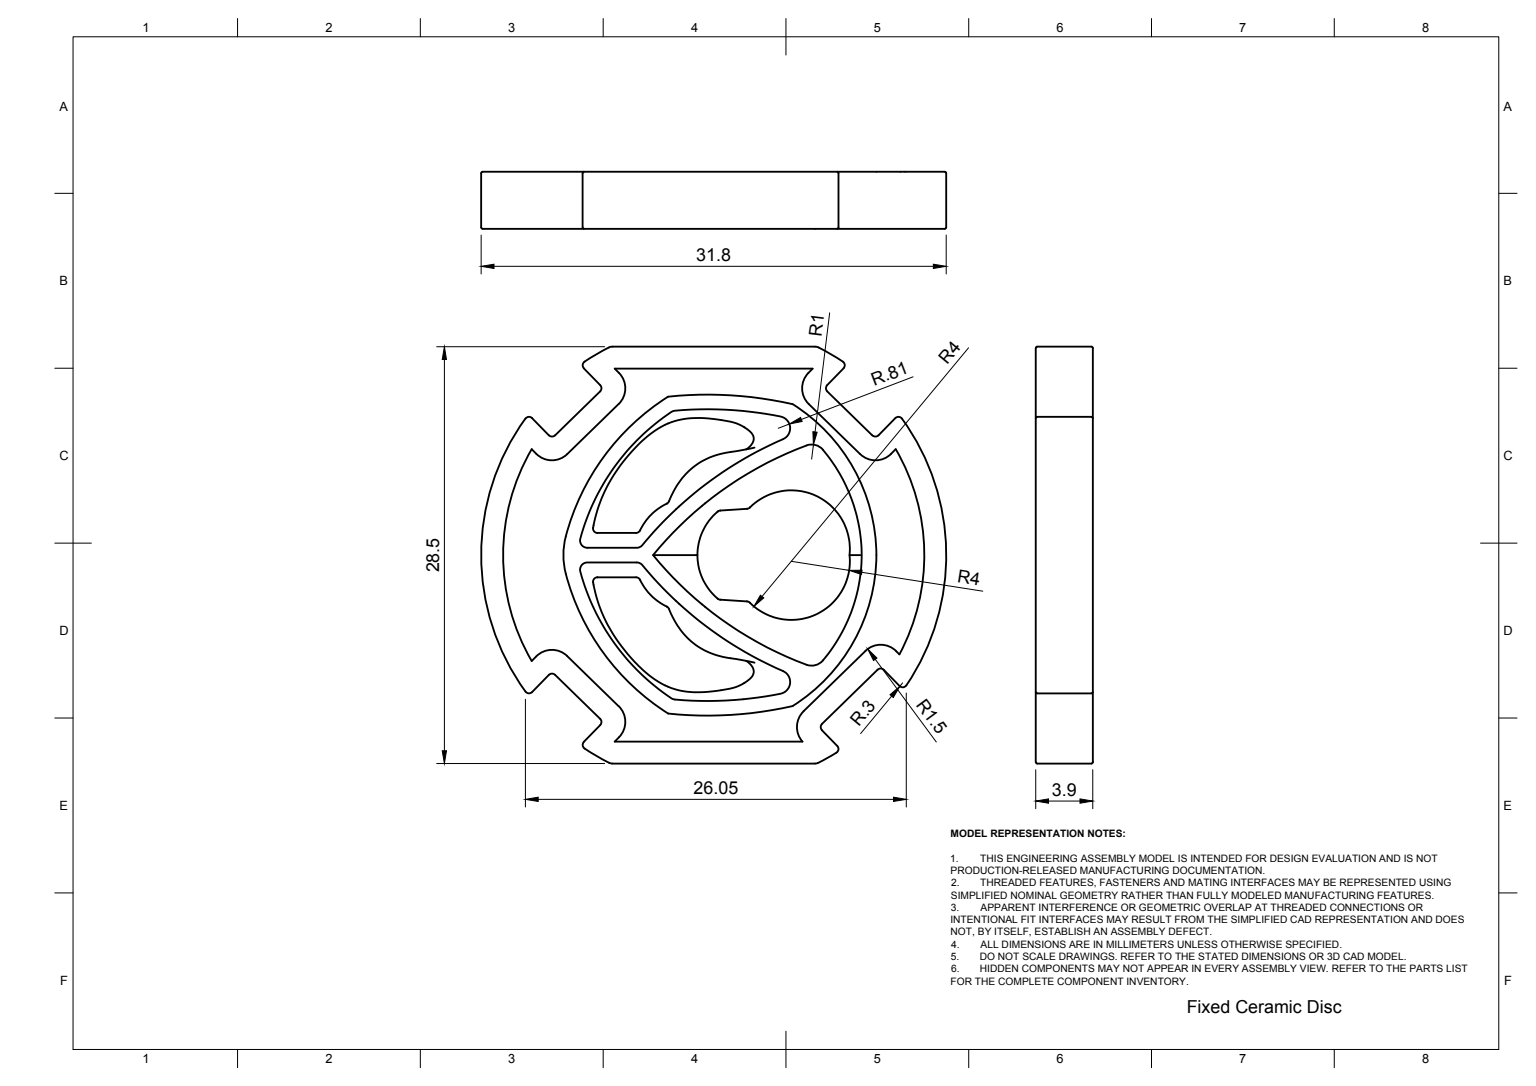
ISO-10303-21;
HEADER;
/* Generated by software containing ST-Developer
 * from STEP Tools, Inc. (www.steptools.com) 
 */

FILE_DESCRIPTION(
/* description */ ('STEP AP214'),
/* implementation_level */ '2;1');

FILE_NAME(
/* name */ 'Fixed Ceramic Disc.step',
/* time_stamp */ '2026-10-06T00:19:40-07:00',
/* author */ (''),
/* organization */ (''),
/* preprocessor_version */ 'ST-DEVELOPER v20.2',
/* originating_system */ 'Autodesk Translation Framework v15.15.0.0',
/* authorisation */ '');

FILE_SCHEMA (('AUTOMOTIVE_DESIGN { 1 0 10303 214 3 1 1 }'));
ENDSEC;

DATA;
#10=MECHANICAL_DESIGN_GEOMETRIC_PRESENTATION_REPRESENTATION('',(#2064),#98302);
#66=TOROIDAL_SURFACE('',#34375,15.8,0.1);
#67=TOROIDAL_SURFACE('',#34378,0.2,0.1);
#68=TOROIDAL_SURFACE('',#34386,0.4,0.1);
#69=TOROIDAL_SURFACE('',#34394,0.4,0.1);
#70=TOROIDAL_SURFACE('',#34402,0.2,0.1);
#71=TOROIDAL_SURFACE('',#34407,15.8,0.1);
#72=TOROIDAL_SURFACE('',#34412,0.4,0.1);
#73=TOROIDAL_SURFACE('',#34420,0.4,0.1);
#74=TOROIDAL_SURFACE('',#34425,15.8,0.1);
#75=TOROIDAL_SURFACE('',#34430,0.2,0.1);
#76=TOROIDAL_SURFACE('',#34438,0.4,0.1);
#77=TOROIDAL_SURFACE('',#34446,0.4,0.1);
#78=TOROIDAL_SURFACE('',#34454,0.2,0.1);
#79=TOROIDAL_SURFACE('',#34462,15.8,0.1);
#80=TOROIDAL_SURFACE('',#34464,0.2,0.1);
#81=TOROIDAL_SURFACE('',#34472,0.4,0.1);
#82=TOROIDAL_SURFACE('',#34480,0.4,0.1);
#83=TOROIDAL_SURFACE('',#34488,0.2,0.1);
#84=TOROIDAL_SURFACE('',#34493,15.8,0.1);
#85=TOROIDAL_SURFACE('',#34498,0.4,0.1);
#86=TOROIDAL_SURFACE('',#34506,0.4,0.1);
#87=TOROIDAL_SURFACE('',#34511,15.8,0.1);
#88=TOROIDAL_SURFACE('',#34516,0.2,0.1);
#89=TOROIDAL_SURFACE('',#34524,0.4,0.1);
#90=TOROIDAL_SURFACE('',#34532,0.2,0.1);
#91=TOROIDAL_SURFACE('',#34537,0.4,0.1);
#92=TOROIDAL_SURFACE('',#34602,15.8,0.1);
#93=TOROIDAL_SURFACE('',#34606,0.2,0.1);
#94=TOROIDAL_SURFACE('',#34611,0.4,0.1);
#95=TOROIDAL_SURFACE('',#34616,0.4,0.1);
#96=TOROIDAL_SURFACE('',#34621,0.2,0.1);
#97=TOROIDAL_SURFACE('',#34624,15.8,0.1);
#98=TOROIDAL_SURFACE('',#34627,0.4,0.1);
#99=TOROIDAL_SURFACE('',#34632,0.4,0.1);
#100=TOROIDAL_SURFACE('',#34635,15.8,0.1);
#101=TOROIDAL_SURFACE('',#34638,0.2,0.1);
#102=TOROIDAL_SURFACE('',#34643,0.4,0.1);
#103=TOROIDAL_SURFACE('',#34648,0.4,0.1);
#104=TOROIDAL_SURFACE('',#34653,0.2,0.1);
#105=TOROIDAL_SURFACE('',#34656,15.8,0.1);
#106=TOROIDAL_SURFACE('',#34659,0.2,0.1);
#107=TOROIDAL_SURFACE('',#34664,0.4,0.1);
#108=TOROIDAL_SURFACE('',#34669,0.4,0.1);
#109=TOROIDAL_SURFACE('',#34674,0.2,0.1);
#110=TOROIDAL_SURFACE('',#34677,15.8,0.1);
#111=TOROIDAL_SURFACE('',#34680,0.4,0.1);
#112=TOROIDAL_SURFACE('',#34685,0.4,0.1);
#113=TOROIDAL_SURFACE('',#34688,15.8,0.1);
#114=TOROIDAL_SURFACE('',#34691,0.2,0.1);
#115=TOROIDAL_SURFACE('',#34696,0.4,0.1);
#116=TOROIDAL_SURFACE('',#34701,0.2,0.1);
#117=TOROIDAL_SURFACE('',#34704,0.4,0.1);
#449=ELLIPSE('',#34351,0.0975089533003066,0.0318233698452749);
#450=ELLIPSE('',#34354,0.210203962458616,0.0684164528781414);
#451=ELLIPSE('',#34355,4.51181641557726,0.330426027279306);
#452=ELLIPSE('',#34356,0.371777616681055,0.0636641381433054);
#453=ELLIPSE('',#34358,1.12077531771054,0.208207940858736);
#454=ELLIPSE('',#34360,7.044836022966,0.27423437971207);
#455=ELLIPSE('',#34362,0.0975089533003066,0.0318233698452749);
#456=ELLIPSE('',#34364,7.044836022966,0.27423437971207);
#457=ELLIPSE('',#34365,1.12077531771054,0.208207940858736);
#458=ELLIPSE('',#34367,0.371777616681055,0.0636641381433054);
#459=ELLIPSE('',#34369,4.51181641557726,0.330426027279306);
#460=ELLIPSE('',#34370,0.210203962458616,0.0684164528781414);
#461=ELLIPSE('',#34546,4.64326105948723,1.41336611178093);
#462=ELLIPSE('',#34562,4.51762701288,1.39428357264109);
#463=ELLIPSE('',#34573,0.257803751558044,0.175002130709107);
#464=ELLIPSE('',#34575,0.1975438935833,0.117585941695249);
#465=ELLIPSE('',#34583,0.249924507512202,0.163903784221422);
#466=ELLIPSE('',#34586,0.1975438935833,0.117585941695249);
#467=ELLIPSE('',#34754,0.0363695267596646,0.0157585247759226);
#468=ELLIPSE('',#34757,0.0363695267596646,0.0157585247759226);
#469=ELLIPSE('',#34761,0.0439364458692703,0.0199986358668788);
#470=ELLIPSE('',#34763,0.751422058778054,0.147149952825287);
#471=ELLIPSE('',#34765,20.1759483174618,1.96800786553162);
#472=ELLIPSE('',#34766,20.1759483174618,1.96800786553162);
#473=ELLIPSE('',#34768,0.751422058778054,0.147149952825287);
#474=ELLIPSE('',#34770,0.0439364458692703,0.0199986358668788);
#475=ELLIPSE('',#34772,0.299969315421473,0.299941755102118);
#476=ELLIPSE('',#34773,0.299972264763754,0.299945275725425);
#477=ELLIPSE('',#34774,0.0990009013291418,0.0878823615802462);
#478=ELLIPSE('',#34780,0.299972288094039,0.299945322652049);
#479=ELLIPSE('',#34781,0.299969314787288,0.299941753885528);
#480=ELLIPSE('',#34782,0.0990009013291418,0.0878823615802462);
#481=ELLIPSE('',#34793,0.7851617239929,0.0246669925758606);
#482=ELLIPSE('',#34796,0.7851617239929,0.0246669925758606);
#710=SPHERICAL_SURFACE('',#34346,0.3);
#711=SPHERICAL_SURFACE('',#34785,0.3);
#862=B_SPLINE_SURFACE_WITH_KNOTS('',5,1,((#49366,#49367),(#49368,#49369),
(#49370,#49371),(#49372,#49373),(#49374,#49375),(#49376,#49377),(#49378,
#49379),(#49380,#49381),(#49382,#49383)),.UNSPECIFIED.,.F.,.F.,.F.,(6,3,
6),(2,2),(0.,2.10936312981,4.22279623369),(0.,3.10437234689),
 .UNSPECIFIED.);
#863=B_SPLINE_SURFACE_WITH_KNOTS('',5,1,((#49466,#49467),(#49468,#49469),
(#49470,#49471),(#49472,#49473),(#49474,#49475),(#49476,#49477),(#49478,
#49479),(#49480,#49481),(#49482,#49483)),.UNSPECIFIED.,.F.,.F.,.F.,(6,3,
6),(2,2),(0.11111371251,1.22636799075,2.75103476973),(0.,0.108300515181936),
 .UNSPECIFIED.);
#864=B_SPLINE_SURFACE_WITH_KNOTS('',5,1,((#49587,#49588),(#49589,#49590),
(#49591,#49592),(#49593,#49594),(#49595,#49596),(#49597,#49598),(#49599,
#49600),(#49601,#49602),(#49603,#49604),(#49605,#49606),(#49607,#49608),
(#49609,#49610),(#49611,#49612),(#49613,#49614),(#49615,#49616),(#49617,
#49618),(#49619,#49620),(#49621,#49622)),.UNSPECIFIED.,.F.,.F.,.F.,(6,3,
3,3,3,6),(2,2),(0.465128126763,3.42050470566,7.30063973795,10.0042092191,
12.4987596036,13.1731669678),(0.,0.115270049227219),.UNSPECIFIED.);
#865=B_SPLINE_SURFACE_WITH_KNOTS('',5,1,((#49746,#49747),(#49748,#49749),
(#49750,#49751),(#49752,#49753),(#49754,#49755),(#49756,#49757)),
 .UNSPECIFIED.,.F.,.F.,.F.,(6,6),(2,2),(0.,1.62525620495),(0.,0.103685293259447),
 .UNSPECIFIED.);
#866=B_SPLINE_SURFACE_WITH_KNOTS('',5,1,((#49791,#49792),(#49793,#49794),
(#49795,#49796),(#49797,#49798),(#49799,#49800),(#49801,#49802),(#49803,
#49804),(#49805,#49806),(#49807,#49808),(#49809,#49810),(#49811,#49812),
(#49813,#49814),(#49815,#49816),(#49817,#49818),(#49819,#49820)),
 .UNSPECIFIED.,.F.,.F.,.F.,(6,3,3,3,6),(2,2),(0.617889185003,0.915206541473,
1.58780472511,2.42003303229,2.57855093571),(0.,0.109749059692414),
 .UNSPECIFIED.);
#867=B_SPLINE_SURFACE_WITH_KNOTS('',5,1,((#49873,#49874),(#49875,#49876),
(#49877,#49878),(#49879,#49880),(#49881,#49882),(#49883,#49884)),
 .UNSPECIFIED.,.F.,.F.,.F.,(6,6),(2,2),(0.,0.788840280269),(0.,0.12),
 .UNSPECIFIED.);
#868=B_SPLINE_SURFACE_WITH_KNOTS('',5,1,((#49932,#49933),(#49934,#49935),
(#49936,#49937),(#49938,#49939),(#49940,#49941),(#49942,#49943),(#49944,
#49945),(#49946,#49947),(#49948,#49949)),.UNSPECIFIED.,.F.,.F.,.F.,(6,3,
6),(2,2),(0.248824060028,2.99459552346,6.14853595161),(0.,0.120001139724),
 .UNSPECIFIED.);
#869=B_SPLINE_SURFACE_WITH_KNOTS('',5,1,((#50067,#50068),(#50069,#50070),
(#50071,#50072),(#50073,#50074),(#50075,#50076),(#50077,#50078),(#50079,
#50080),(#50081,#50082),(#50083,#50084)),.UNSPECIFIED.,.F.,.F.,.F.,(6,3,
6),(2,2),(0.11111371251,1.22636799075,2.75103476973),(0.,0.108300515181936),
 .UNSPECIFIED.);
#870=B_SPLINE_SURFACE_WITH_KNOTS('',5,1,((#50165,#50166),(#50167,#50168),
(#50169,#50170),(#50171,#50172),(#50173,#50174),(#50175,#50176),(#50177,
#50178),(#50179,#50180),(#50181,#50182)),.UNSPECIFIED.,.F.,.F.,.F.,(6,3,
6),(2,2),(0.248824060028,2.99459552346,6.14853595161),(0.,0.120001139724),
 .UNSPECIFIED.);
#871=B_SPLINE_SURFACE_WITH_KNOTS('',5,1,((#50281,#50282),(#50283,#50284),
(#50285,#50286),(#50287,#50288),(#50289,#50290),(#50291,#50292)),
 .UNSPECIFIED.,.F.,.F.,.F.,(6,6),(2,2),(0.,0.788840280269),(0.,0.12),
 .UNSPECIFIED.);
#872=B_SPLINE_SURFACE_WITH_KNOTS('',5,1,((#50340,#50341),(#50342,#50343),
(#50344,#50345),(#50346,#50347),(#50348,#50349),(#50350,#50351),(#50352,
#50353),(#50354,#50355),(#50356,#50357),(#50358,#50359),(#50360,#50361),
(#50362,#50363),(#50364,#50365),(#50366,#50367),(#50368,#50369)),
 .UNSPECIFIED.,.F.,.F.,.F.,(6,3,3,3,6),(2,2),(0.617889185003,0.915206541473,
1.58780472511,2.42003303229,2.57855093571),(0.,0.109749059692414),
 .UNSPECIFIED.);
#873=B_SPLINE_SURFACE_WITH_KNOTS('',5,1,((#50555,#50556),(#50557,#50558),
(#50559,#50560),(#50561,#50562),(#50563,#50564),(#50565,#50566)),
 .UNSPECIFIED.,.F.,.F.,.F.,(6,6),(2,2),(0.,1.62525620495),(0.,0.103685293259447),
 .UNSPECIFIED.);
#874=B_SPLINE_SURFACE_WITH_KNOTS('',5,1,((#50600,#50601),(#50602,#50603),
(#50604,#50605),(#50606,#50607),(#50608,#50609),(#50610,#50611),(#50612,
#50613),(#50614,#50615),(#50616,#50617),(#50618,#50619),(#50620,#50621),
(#50622,#50623),(#50624,#50625),(#50626,#50627),(#50628,#50629),(#50630,
#50631),(#50632,#50633),(#50634,#50635)),.UNSPECIFIED.,.F.,.F.,.F.,(6,3,
3,3,3,6),(2,2),(0.465128126763,3.42050470566,7.30063973795,10.0042092191,
12.4987596036,13.1731669678),(0.,0.115270054056779),.UNSPECIFIED.);
#875=B_SPLINE_SURFACE_WITH_KNOTS('',5,1,((#51251,#51252),(#51253,#51254),
(#51255,#51256),(#51257,#51258),(#51259,#51260),(#51261,#51262)),
 .UNSPECIFIED.,.F.,.F.,.F.,(6,6),(2,2),(0.,0.600083611309),(0.,3.10437234689),
 .UNSPECIFIED.);
#876=B_SPLINE_SURFACE_WITH_KNOTS('',5,1,((#51336,#51337),(#51338,#51339),
(#51340,#51341),(#51342,#51343),(#51344,#51345),(#51346,#51347)),
 .UNSPECIFIED.,.F.,.F.,.F.,(6,6),(2,2),(0.,0.226010362356),(0.,3.10437234689),
 .UNSPECIFIED.);
#877=B_SPLINE_SURFACE_WITH_KNOTS('',5,1,((#51368,#51369),(#51370,#51371),
(#51372,#51373),(#51374,#51375),(#51376,#51377),(#51378,#51379),(#51380,
#51381),(#51382,#51383),(#51384,#51385),(#51386,#51387),(#51388,#51389),
(#51390,#51391)),.UNSPECIFIED.,.F.,.F.,.F.,(6,3,3,6),(2,2),(0.,2.83532528452,
6.09533201542,9.83397913335),(0.,3.10437234689),.UNSPECIFIED.);
#878=B_SPLINE_SURFACE_WITH_KNOTS('',5,1,((#51471,#51472),(#51473,#51474),
(#51475,#51476),(#51477,#51478),(#51479,#51480),(#51481,#51482)),
 .UNSPECIFIED.,.F.,.F.,.F.,(6,6),(2,2),(0.,0.224378834114),(0.,3.10437234689),
 .UNSPECIFIED.);
#879=B_SPLINE_SURFACE_WITH_KNOTS('',5,1,((#51514,#51515),(#51516,#51517),
(#51518,#51519),(#51520,#51521),(#51522,#51523),(#51524,#51525)),
 .UNSPECIFIED.,.F.,.F.,.F.,(6,6),(2,2),(0.,0.2489231439),(0.,3.10437234689),
 .UNSPECIFIED.);
#880=B_SPLINE_SURFACE_WITH_KNOTS('',5,1,((#51570,#51571),(#51572,#51573),
(#51574,#51575),(#51576,#51577),(#51578,#51579),(#51580,#51581),(#51582,
#51583),(#51584,#51585),(#51586,#51587),(#51588,#51589),(#51590,#51591),
(#51592,#51593)),.UNSPECIFIED.,.F.,.F.,.F.,(6,3,3,6),(2,2),(0.,0.629547398659,
1.2493532974,1.86132516749),(0.,3.10437234689),.UNSPECIFIED.);
#881=B_SPLINE_SURFACE_WITH_KNOTS('',5,1,((#51679,#51680),(#51681,#51682),
(#51683,#51684),(#51685,#51686),(#51687,#51688),(#51689,#51690)),
 .UNSPECIFIED.,.F.,.F.,.F.,(6,6),(2,2),(0.,0.482067685837),(0.,3.10437234689),
 .UNSPECIFIED.);
#882=B_SPLINE_SURFACE_WITH_KNOTS('',5,1,((#51717,#51718),(#51719,#51720),
(#51721,#51722),(#51723,#51724),(#51725,#51726),(#51727,#51728)),
 .UNSPECIFIED.,.F.,.F.,.F.,(6,6),(2,2),(0.,1.84813202664),(0.,3.10437234689),
 .UNSPECIFIED.);
#883=B_SPLINE_SURFACE_WITH_KNOTS('',5,5,((#51829,#51830,#51831,#51832,#51833,
#51834),(#51835,#51836,#51837,#51838,#51839,#51840),(#51841,#51842,#51843,
#51844,#51845,#51846),(#51847,#51848,#51849,#51850,#51851,#51852),(#51853,
#51854,#51855,#51856,#51857,#51858),(#51859,#51860,#51861,#51862,#51863,
#51864)),.UNSPECIFIED.,.F.,.F.,.F.,(6,6),(6,6),(0.840058180513,4.79280767082),
(0.,1.),.UNSPECIFIED.);
#884=B_SPLINE_SURFACE_WITH_KNOTS('',5,5,((#51900,#51901,#51902,#51903,#51904,
#51905),(#51906,#51907,#51908,#51909,#51910,#51911),(#51912,#51913,#51914,
#51915,#51916,#51917),(#51918,#51919,#51920,#51921,#51922,#51923),(#51924,
#51925,#51926,#51927,#51928,#51929),(#51930,#51931,#51932,#51933,#51934,
#51935),(#51936,#51937,#51938,#51939,#51940,#51941),(#51942,#51943,#51944,
#51945,#51946,#51947),(#51948,#51949,#51950,#51951,#51952,#51953)),
 .UNSPECIFIED.,.F.,.F.,.F.,(6,3,6),(6,6),(0.225815728085,0.523709124902,
0.747252061964),(0.,1.),.UNSPECIFIED.);
#885=B_SPLINE_SURFACE_WITH_KNOTS('',5,5,((#51995,#51996,#51997,#51998,#51999,
#52000),(#52001,#52002,#52003,#52004,#52005,#52006),(#52007,#52008,#52009,
#52010,#52011,#52012),(#52013,#52014,#52015,#52016,#52017,#52018),(#52019,
#52020,#52021,#52022,#52023,#52024),(#52025,#52026,#52027,#52028,#52029,
#52030)),.UNSPECIFIED.,.F.,.F.,.F.,(6,6),(6,6),(1.28339894164,1.34350433703),
(0.,1.),.UNSPECIFIED.);
#886=B_SPLINE_SURFACE_WITH_KNOTS('',5,5,((#52045,#52046,#52047,#52048,#52049,
#52050),(#52051,#52052,#52053,#52054,#52055,#52056),(#52057,#52058,#52059,
#52060,#52061,#52062),(#52063,#52064,#52065,#52066,#52067,#52068),(#52069,
#52070,#52071,#52072,#52073,#52074),(#52075,#52076,#52077,#52078,#52079,
#52080)),.UNSPECIFIED.,.F.,.F.,.F.,(6,6),(6,6),(1.036743613,1.10280574369),
(0.,1.),.UNSPECIFIED.);
#887=B_SPLINE_SURFACE_WITH_KNOTS('',5,5,((#52086,#52087,#52088,#52089,#52090,
#52091),(#52092,#52093,#52094,#52095,#52096,#52097),(#52098,#52099,#52100,
#52101,#52102,#52103),(#52104,#52105,#52106,#52107,#52108,#52109),(#52110,
#52111,#52112,#52113,#52114,#52115),(#52116,#52117,#52118,#52119,#52120,
#52121),(#52122,#52123,#52124,#52125,#52126,#52127),(#52128,#52129,#52130,
#52131,#52132,#52133),(#52134,#52135,#52136,#52137,#52138,#52139)),
 .UNSPECIFIED.,.F.,.F.,.F.,(6,3,6),(6,6),(0.342430056326,0.787545489389,
1.14838178471),(0.,1.),.UNSPECIFIED.);
#888=B_SPLINE_SURFACE_WITH_KNOTS('',5,5,((#52179,#52180,#52181,#52182,#52183,
#52184),(#52185,#52186,#52187,#52188,#52189,#52190),(#52191,#52192,#52193,
#52194,#52195,#52196),(#52197,#52198,#52199,#52200,#52201,#52202),(#52203,
#52204,#52205,#52206,#52207,#52208),(#52209,#52210,#52211,#52212,#52213,
#52214)),.UNSPECIFIED.,.F.,.F.,.F.,(6,6),(6,6),(1.40817420416,1.45205022904),
(0.,1.),.UNSPECIFIED.);
#889=B_SPLINE_SURFACE_WITH_KNOTS('',5,5,((#52216,#52217,#52218,#52219,#52220,
#52221),(#52222,#52223,#52224,#52225,#52226,#52227),(#52228,#52229,#52230,
#52231,#52232,#52233),(#52234,#52235,#52236,#52237,#52238,#52239),(#52240,
#52241,#52242,#52243,#52244,#52245),(#52246,#52247,#52248,#52249,#52250,
#52251),(#52252,#52253,#52254,#52255,#52256,#52257),(#52258,#52259,#52260,
#52261,#52262,#52263),(#52264,#52265,#52266,#52267,#52268,#52269),(#52270,
#52271,#52272,#52273,#52274,#52275),(#52276,#52277,#52278,#52279,#52280,
#52281),(#52282,#52283,#52284,#52285,#52286,#52287)),.UNSPECIFIED.,.F.,
 .F.,.F.,(6,3,3,6),(6,6),(4.46364567829,9.98301756848,13.6615164274,17.5757040899),
(0.,1.),.UNSPECIFIED.);
#890=B_SPLINE_SURFACE_WITH_KNOTS('',5,5,((#52425,#52426,#52427,#52428,#52429,
#52430),(#52431,#52432,#52433,#52434,#52435,#52436),(#52437,#52438,#52439,
#52440,#52441,#52442),(#52443,#52444,#52445,#52446,#52447,#52448),(#52449,
#52450,#52451,#52452,#52453,#52454),(#52455,#52456,#52457,#52458,#52459,
#52460),(#52461,#52462,#52463,#52464,#52465,#52466),(#52467,#52468,#52469,
#52470,#52471,#52472),(#52473,#52474,#52475,#52476,#52477,#52478)),
 .UNSPECIFIED.,.F.,.F.,.F.,(6,3,6),(6,6),(1.01054285509,1.23011259501,1.32384910338),
(0.,1.),.UNSPECIFIED.);
#891=B_SPLINE_SURFACE_WITH_KNOTS('',5,5,((#52506,#52507,#52508,#52509,#52510,
#52511),(#52512,#52513,#52514,#52515,#52516,#52517),(#52518,#52519,#52520,
#52521,#52522,#52523),(#52524,#52525,#52526,#52527,#52528,#52529),(#52530,
#52531,#52532,#52533,#52534,#52535),(#52536,#52537,#52538,#52539,#52540,
#52541),(#52542,#52543,#52544,#52545,#52546,#52547),(#52548,#52549,#52550,
#52551,#52552,#52553),(#52554,#52555,#52556,#52557,#52558,#52559)),
 .UNSPECIFIED.,.F.,.F.,.F.,(6,3,6),(6,6),(2.57539738198,5.72432320356,8.12037630607),
(0.,1.),.UNSPECIFIED.);
#892=B_SPLINE_SURFACE_WITH_KNOTS('',5,5,((#52650,#52651,#52652,#52653,#52654,
#52655),(#52656,#52657,#52658,#52659,#52660,#52661),(#52662,#52663,#52664,
#52665,#52666,#52667),(#52668,#52669,#52670,#52671,#52672,#52673),(#52674,
#52675,#52676,#52677,#52678,#52679),(#52680,#52681,#52682,#52683,#52684,
#52685)),.UNSPECIFIED.,.F.,.F.,.F.,(6,6),(6,6),(0.993700418328028,1.22287270565897),
(-0.00157928356897239,1.00011077696173),.UNSPECIFIED.);
#893=B_SPLINE_SURFACE_WITH_KNOTS('',5,5,((#52690,#52691,#52692,#52693,#52694,
#52695),(#52696,#52697,#52698,#52699,#52700,#52701),(#52702,#52703,#52704,
#52705,#52706,#52707),(#52708,#52709,#52710,#52711,#52712,#52713),(#52714,
#52715,#52716,#52717,#52718,#52719),(#52720,#52721,#52722,#52723,#52724,
#52725)),.UNSPECIFIED.,.F.,.F.,.F.,(6,6),(6,6),(2.37851323355,2.46410111513),
(0.,1.),.UNSPECIFIED.);
#894=B_SPLINE_SURFACE_WITH_KNOTS('',5,5,((#52738,#52739,#52740,#52741,#52742,
#52743),(#52744,#52745,#52746,#52747,#52748,#52749),(#52750,#52751,#52752,
#52753,#52754,#52755),(#52756,#52757,#52758,#52759,#52760,#52761),(#52762,
#52763,#52764,#52765,#52766,#52767),(#52768,#52769,#52770,#52771,#52772,
#52773),(#52774,#52775,#52776,#52777,#52778,#52779),(#52780,#52781,#52782,
#52783,#52784,#52785),(#52786,#52787,#52788,#52789,#52790,#52791)),
 .UNSPECIFIED.,.F.,.F.,.F.,(6,3,6),(6,6),(0.586327318555,1.59285457075,
2.96825275179),(0.,1.),.UNSPECIFIED.);
#895=B_SPLINE_SURFACE_WITH_KNOTS('',5,5,((#52906,#52907,#52908,#52909,#52910,
#52911),(#52912,#52913,#52914,#52915,#52916,#52917),(#52918,#52919,#52920,
#52921,#52922,#52923),(#52924,#52925,#52926,#52927,#52928,#52929),(#52930,
#52931,#52932,#52933,#52934,#52935),(#52936,#52937,#52938,#52939,#52940,
#52941)),.UNSPECIFIED.,.F.,.F.,.F.,(6,6),(6,6),(0.881014033286,0.963434555076),
(0.,1.),.UNSPECIFIED.);
#896=B_SPLINE_SURFACE_WITH_KNOTS('',5,5,((#52951,#52952,#52953,#52954,#52955,
#52956),(#52957,#52958,#52959,#52960,#52961,#52962),(#52963,#52964,#52965,
#52966,#52967,#52968),(#52969,#52970,#52971,#52972,#52973,#52974),(#52975,
#52976,#52977,#52978,#52979,#52980),(#52981,#52982,#52983,#52984,#52985,
#52986),(#52987,#52988,#52989,#52990,#52991,#52992),(#52993,#52994,#52995,
#52996,#52997,#52998),(#52999,#53000,#53001,#53002,#53003,#53004)),
 .UNSPECIFIED.,.F.,.F.,.F.,(6,3,6),(6,6),(0.734432475987,1.16119681048,
1.33983380059),(0.,1.),.UNSPECIFIED.);
#897=B_SPLINE_SURFACE_WITH_KNOTS('',5,5,((#53026,#53027,#53028,#53029,#53030,
#53031),(#53032,#53033,#53034,#53035,#53036,#53037),(#53038,#53039,#53040,
#53041,#53042,#53043),(#53044,#53045,#53046,#53047,#53048,#53049),(#53050,
#53051,#53052,#53053,#53054,#53055),(#53056,#53057,#53058,#53059,#53060,
#53061),(#53062,#53063,#53064,#53065,#53066,#53067),(#53068,#53069,#53070,
#53071,#53072,#53073),(#53074,#53075,#53076,#53077,#53078,#53079),(#53080,
#53081,#53082,#53083,#53084,#53085),(#53086,#53087,#53088,#53089,#53090,
#53091),(#53092,#53093,#53094,#53095,#53096,#53097)),.UNSPECIFIED.,.F.,
 .F.,.F.,(6,3,3,6),(6,6),(1.14300114544,1.64244110169,2.30706085766,3.58561463726),
(0.,1.),.UNSPECIFIED.);
#898=B_SPLINE_SURFACE_WITH_KNOTS('',5,5,((#53200,#53201,#53202,#53203,#53204,
#53205),(#53206,#53207,#53208,#53209,#53210,#53211),(#53212,#53213,#53214,
#53215,#53216,#53217),(#53218,#53219,#53220,#53221,#53222,#53223),(#53224,
#53225,#53226,#53227,#53228,#53229),(#53230,#53231,#53232,#53233,#53234,
#53235)),.UNSPECIFIED.,.F.,.F.,.F.,(6,6),(6,6),(1.26425849888,1.32115953697),
(0.,1.),.UNSPECIFIED.);
#899=B_SPLINE_SURFACE_WITH_KNOTS('',5,1,((#53242,#53243),(#53244,#53245),
(#53246,#53247),(#53248,#53249),(#53250,#53251),(#53252,#53253)),
 .UNSPECIFIED.,.F.,.F.,.F.,(6,6),(2,2),(0.,0.898161272296),(0.,3.10437234689),
 .UNSPECIFIED.);
#900=B_SPLINE_SURFACE_WITH_KNOTS('',3,5,((#53286,#53287,#53288,#53289,#53290,
#53291),(#53292,#53293,#53294,#53295,#53296,#53297),(#53298,#53299,#53300,
#53301,#53302,#53303),(#53304,#53305,#53306,#53307,#53308,#53309)),
 .UNSPECIFIED.,.F.,.F.,.F.,(4,4),(6,6),(0.338318706236,0.636935495757),
(0.,1.),.UNSPECIFIED.);
#901=B_SPLINE_SURFACE_WITH_KNOTS('',5,1,((#53310,#53311),(#53312,#53313),
(#53314,#53315),(#53316,#53317),(#53318,#53319),(#53320,#53321),(#53322,
#53323),(#53324,#53325),(#53326,#53327)),.UNSPECIFIED.,.F.,.F.,.F.,(6,3,
6),(2,2),(0.,3.38335932988,6.7689179912),(-4.93438140460603E-6,3.10437234689),
 .UNSPECIFIED.);
#902=B_SPLINE_SURFACE_WITH_KNOTS('',5,5,((#53466,#53467,#53468,#53469,#53470,
#53471),(#53472,#53473,#53474,#53475,#53476,#53477),(#53478,#53479,#53480,
#53481,#53482,#53483),(#53484,#53485,#53486,#53487,#53488,#53489),(#53490,
#53491,#53492,#53493,#53494,#53495),(#53496,#53497,#53498,#53499,#53500,
#53501),(#53502,#53503,#53504,#53505,#53506,#53507),(#53508,#53509,#53510,
#53511,#53512,#53513),(#53514,#53515,#53516,#53517,#53518,#53519),(#53520,
#53521,#53522,#53523,#53524,#53525),(#53526,#53527,#53528,#53529,#53530,
#53531),(#53532,#53533,#53534,#53535,#53536,#53537)),.UNSPECIFIED.,.F.,
 .F.,.F.,(6,3,3,6),(6,6),(0.,2.20713855153,4.85810064575,8.61717037377),
(0.,1.),.UNSPECIFIED.);
#903=B_SPLINE_SURFACE_WITH_KNOTS('',5,5,((#53539,#53540,#53541,#53542,#53543,
#53544),(#53545,#53546,#53547,#53548,#53549,#53550),(#53551,#53552,#53553,
#53554,#53555,#53556),(#53557,#53558,#53559,#53560,#53561,#53562),(#53563,
#53564,#53565,#53566,#53567,#53568),(#53569,#53570,#53571,#53572,#53573,
#53574)),.UNSPECIFIED.,.F.,.F.,.F.,(6,6),(6,6),(2.946262962,2.98811189909),
(0.,1.),.UNSPECIFIED.);
#904=B_SPLINE_SURFACE_WITH_KNOTS('',5,5,((#53578,#53579,#53580,#53581,#53582,
#53583),(#53584,#53585,#53586,#53587,#53588,#53589),(#53590,#53591,#53592,
#53593,#53594,#53595),(#53596,#53597,#53598,#53599,#53600,#53601),(#53602,
#53603,#53604,#53605,#53606,#53607),(#53608,#53609,#53610,#53611,#53612,
#53613),(#53614,#53615,#53616,#53617,#53618,#53619),(#53620,#53621,#53622,
#53623,#53624,#53625),(#53626,#53627,#53628,#53629,#53630,#53631)),
 .UNSPECIFIED.,.F.,.F.,.F.,(6,3,6),(6,6),(0.160705691504905,0.296334742315,
0.49268070055009),(-0.00285589455108982,1.),.UNSPECIFIED.);
#905=B_SPLINE_SURFACE_WITH_KNOTS('',5,5,((#53652,#53653,#53654,#53655,#53656,
#53657),(#53658,#53659,#53660,#53661,#53662,#53663),(#53664,#53665,#53666,
#53667,#53668,#53669),(#53670,#53671,#53672,#53673,#53674,#53675),(#53676,
#53677,#53678,#53679,#53680,#53681),(#53682,#53683,#53684,#53685,#53686,
#53687)),.UNSPECIFIED.,.F.,.F.,.F.,(6,6),(6,6),(1.51692742518,1.55221398826),
(0.,1.),.UNSPECIFIED.);
#906=B_SPLINE_SURFACE_WITH_KNOTS('',5,5,((#53688,#53689,#53690,#53691,#53692,
#53693),(#53694,#53695,#53696,#53697,#53698,#53699),(#53700,#53701,#53702,
#53703,#53704,#53705),(#53706,#53707,#53708,#53709,#53710,#53711),(#53712,
#53713,#53714,#53715,#53716,#53717),(#53718,#53719,#53720,#53721,#53722,
#53723)),.UNSPECIFIED.,.F.,.F.,.F.,(6,6),(6,6),(1.28339894164,1.34350433703),
(0.,1.),.UNSPECIFIED.);
#907=B_SPLINE_SURFACE_WITH_KNOTS('',5,5,((#53738,#53739,#53740,#53741,#53742,
#53743),(#53744,#53745,#53746,#53747,#53748,#53749),(#53750,#53751,#53752,
#53753,#53754,#53755),(#53756,#53757,#53758,#53759,#53760,#53761),(#53762,
#53763,#53764,#53765,#53766,#53767),(#53768,#53769,#53770,#53771,#53772,
#53773),(#53774,#53775,#53776,#53777,#53778,#53779),(#53780,#53781,#53782,
#53783,#53784,#53785),(#53786,#53787,#53788,#53789,#53790,#53791)),
 .UNSPECIFIED.,.F.,.F.,.F.,(6,3,6),(6,6),(0.225815728085,0.523709124902,
0.747252061964),(0.,1.),.UNSPECIFIED.);
#908=B_SPLINE_SURFACE_WITH_KNOTS('',5,5,((#53802,#53803,#53804,#53805,#53806,
#53807),(#53808,#53809,#53810,#53811,#53812,#53813),(#53814,#53815,#53816,
#53817,#53818,#53819),(#53820,#53821,#53822,#53823,#53824,#53825),(#53826,
#53827,#53828,#53829,#53830,#53831),(#53832,#53833,#53834,#53835,#53836,
#53837)),.UNSPECIFIED.,.F.,.F.,.F.,(6,6),(6,6),(0.840058180513,4.79280767082),
(0.,1.),.UNSPECIFIED.);
#909=B_SPLINE_SURFACE_WITH_KNOTS('',5,5,((#53846,#53847,#53848,#53849,#53850,
#53851),(#53852,#53853,#53854,#53855,#53856,#53857),(#53858,#53859,#53860,
#53861,#53862,#53863),(#53864,#53865,#53866,#53867,#53868,#53869),(#53870,
#53871,#53872,#53873,#53874,#53875),(#53876,#53877,#53878,#53879,#53880,
#53881)),.UNSPECIFIED.,.F.,.F.,.F.,(6,6),(6,6),(1.51692742518,1.55221398826),
(0.,1.),.UNSPECIFIED.);
#910=B_SPLINE_SURFACE_WITH_KNOTS('',5,5,((#53886,#53887,#53888,#53889,#53890,
#53891),(#53892,#53893,#53894,#53895,#53896,#53897),(#53898,#53899,#53900,
#53901,#53902,#53903),(#53904,#53905,#53906,#53907,#53908,#53909),(#53910,
#53911,#53912,#53913,#53914,#53915),(#53916,#53917,#53918,#53919,#53920,
#53921),(#53922,#53923,#53924,#53925,#53926,#53927),(#53928,#53929,#53930,
#53931,#53932,#53933),(#53934,#53935,#53936,#53937,#53938,#53939)),
 .UNSPECIFIED.,.F.,.F.,.F.,(6,3,6),(6,6),(0.163561586047,0.296334742315,
0.489824805999),(0.,1.),.UNSPECIFIED.);
#911=B_SPLINE_SURFACE_WITH_KNOTS('',5,5,((#53941,#53942,#53943,#53944,#53945,
#53946),(#53947,#53948,#53949,#53950,#53951,#53952),(#53953,#53954,#53955,
#53956,#53957,#53958),(#53959,#53960,#53961,#53962,#53963,#53964),(#53965,
#53966,#53967,#53968,#53969,#53970),(#53971,#53972,#53973,#53974,#53975,
#53976)),.UNSPECIFIED.,.F.,.F.,.F.,(6,6),(6,6),(2.946262962,2.98811189909),
(0.,1.),.UNSPECIFIED.);
#912=B_SPLINE_SURFACE_WITH_KNOTS('',5,5,((#53978,#53979,#53980,#53981,#53982,
#53983),(#53984,#53985,#53986,#53987,#53988,#53989),(#53990,#53991,#53992,
#53993,#53994,#53995),(#53996,#53997,#53998,#53999,#54000,#54001),(#54002,
#54003,#54004,#54005,#54006,#54007),(#54008,#54009,#54010,#54011,#54012,
#54013),(#54014,#54015,#54016,#54017,#54018,#54019),(#54020,#54021,#54022,
#54023,#54024,#54025),(#54026,#54027,#54028,#54029,#54030,#54031),(#54032,
#54033,#54034,#54035,#54036,#54037),(#54038,#54039,#54040,#54041,#54042,
#54043),(#54044,#54045,#54046,#54047,#54048,#54049)),.UNSPECIFIED.,.F.,
 .F.,.F.,(6,3,3,6),(6,6),(0.,2.20713855153,4.85810064575,8.61717037377),
(0.,1.),.UNSPECIFIED.);
#913=B_SPLINE_SURFACE_WITH_KNOTS('',5,1,((#54062,#54063),(#54064,#54065),
(#54066,#54067),(#54068,#54069),(#54070,#54071),(#54072,#54073),(#54074,
#54075),(#54076,#54077),(#54078,#54079)),.UNSPECIFIED.,.F.,.F.,.F.,(6,3,
6),(2,2),(0.,3.38335932988,6.7689179912),(-1.30243697672538E-5,3.10437234689),
 .UNSPECIFIED.);
#914=B_SPLINE_SURFACE_WITH_KNOTS('',5,1,((#54088,#54089),(#54090,#54091),
(#54092,#54093),(#54094,#54095),(#54096,#54097),(#54098,#54099)),
 .UNSPECIFIED.,.F.,.F.,.F.,(6,6),(2,2),(0.,0.898161272296),(0.,3.10437234689),
 .UNSPECIFIED.);
#915=B_SPLINE_SURFACE_WITH_KNOTS('',3,5,((#54135,#54136,#54137,#54138,#54139,
#54140),(#54141,#54142,#54143,#54144,#54145,#54146),(#54147,#54148,#54149,
#54150,#54151,#54152),(#54153,#54154,#54155,#54156,#54157,#54158)),
 .UNSPECIFIED.,.F.,.F.,.F.,(4,4),(6,6),(0.338318706236,0.636935495757),
(0.,1.),.UNSPECIFIED.);
#916=B_SPLINE_SURFACE_WITH_KNOTS('',5,5,((#54160,#54161,#54162,#54163,#54164,
#54165),(#54166,#54167,#54168,#54169,#54170,#54171),(#54172,#54173,#54174,
#54175,#54176,#54177),(#54178,#54179,#54180,#54181,#54182,#54183),(#54184,
#54185,#54186,#54187,#54188,#54189),(#54190,#54191,#54192,#54193,#54194,
#54195)),.UNSPECIFIED.,.F.,.F.,.F.,(6,6),(6,6),(1.26425849888,1.32115953697),
(0.,1.),.UNSPECIFIED.);
#917=B_SPLINE_SURFACE_WITH_KNOTS('',5,5,((#54197,#54198,#54199,#54200,#54201,
#54202),(#54203,#54204,#54205,#54206,#54207,#54208),(#54209,#54210,#54211,
#54212,#54213,#54214),(#54215,#54216,#54217,#54218,#54219,#54220),(#54221,
#54222,#54223,#54224,#54225,#54226),(#54227,#54228,#54229,#54230,#54231,
#54232),(#54233,#54234,#54235,#54236,#54237,#54238),(#54239,#54240,#54241,
#54242,#54243,#54244),(#54245,#54246,#54247,#54248,#54249,#54250),(#54251,
#54252,#54253,#54254,#54255,#54256),(#54257,#54258,#54259,#54260,#54261,
#54262),(#54263,#54264,#54265,#54266,#54267,#54268)),.UNSPECIFIED.,.F.,
 .F.,.F.,(6,3,3,6),(6,6),(1.14300114544,1.64244110169,2.30706085766,3.58561463726),
(0.,1.),.UNSPECIFIED.);
#918=B_SPLINE_SURFACE_WITH_KNOTS('',5,5,((#54270,#54271,#54272,#54273,#54274,
#54275),(#54276,#54277,#54278,#54279,#54280,#54281),(#54282,#54283,#54284,
#54285,#54286,#54287),(#54288,#54289,#54290,#54291,#54292,#54293),(#54294,
#54295,#54296,#54297,#54298,#54299),(#54300,#54301,#54302,#54303,#54304,
#54305),(#54306,#54307,#54308,#54309,#54310,#54311),(#54312,#54313,#54314,
#54315,#54316,#54317),(#54318,#54319,#54320,#54321,#54322,#54323)),
 .UNSPECIFIED.,.F.,.F.,.F.,(6,3,6),(6,6),(0.734432475987,1.16119681048,
1.33983380059),(0.,1.),.UNSPECIFIED.);
#919=B_SPLINE_SURFACE_WITH_KNOTS('',5,5,((#54325,#54326,#54327,#54328,#54329,
#54330),(#54331,#54332,#54333,#54334,#54335,#54336),(#54337,#54338,#54339,
#54340,#54341,#54342),(#54343,#54344,#54345,#54346,#54347,#54348),(#54349,
#54350,#54351,#54352,#54353,#54354),(#54355,#54356,#54357,#54358,#54359,
#54360)),.UNSPECIFIED.,.F.,.F.,.F.,(6,6),(6,6),(0.881014033286,0.963434555076),
(0.,1.),.UNSPECIFIED.);
#920=B_SPLINE_SURFACE_WITH_KNOTS('',5,5,((#54362,#54363,#54364,#54365,#54366,
#54367),(#54368,#54369,#54370,#54371,#54372,#54373),(#54374,#54375,#54376,
#54377,#54378,#54379),(#54380,#54381,#54382,#54383,#54384,#54385),(#54386,
#54387,#54388,#54389,#54390,#54391),(#54392,#54393,#54394,#54395,#54396,
#54397),(#54398,#54399,#54400,#54401,#54402,#54403),(#54404,#54405,#54406,
#54407,#54408,#54409),(#54410,#54411,#54412,#54413,#54414,#54415)),
 .UNSPECIFIED.,.F.,.F.,.F.,(6,3,6),(6,6),(0.586327318555,1.59285457075,
2.96825275179),(0.,1.),.UNSPECIFIED.);
#921=B_SPLINE_SURFACE_WITH_KNOTS('',5,5,((#54417,#54418,#54419,#54420,#54421,
#54422),(#54423,#54424,#54425,#54426,#54427,#54428),(#54429,#54430,#54431,
#54432,#54433,#54434),(#54435,#54436,#54437,#54438,#54439,#54440),(#54441,
#54442,#54443,#54444,#54445,#54446),(#54447,#54448,#54449,#54450,#54451,
#54452)),.UNSPECIFIED.,.F.,.F.,.F.,(6,6),(6,6),(2.37851323355,2.46410111513),
(0.,1.),.UNSPECIFIED.);
#922=B_SPLINE_SURFACE_WITH_KNOTS('',5,5,((#54454,#54455,#54456,#54457,#54458,
#54459),(#54460,#54461,#54462,#54463,#54464,#54465),(#54466,#54467,#54468,
#54469,#54470,#54471),(#54472,#54473,#54474,#54475,#54476,#54477),(#54478,
#54479,#54480,#54481,#54482,#54483),(#54484,#54485,#54486,#54487,#54488,
#54489),(#54490,#54491,#54492,#54493,#54494,#54495),(#54496,#54497,#54498,
#54499,#54500,#54501),(#54502,#54503,#54504,#54505,#54506,#54507)),
 .UNSPECIFIED.,.F.,.F.,.F.,(6,3,6),(6,6),(2.57539738198,5.72432320356,8.12037630607),
(0.,1.),.UNSPECIFIED.);
#923=B_SPLINE_SURFACE_WITH_KNOTS('',5,5,((#54509,#54510,#54511,#54512,#54513,
#54514),(#54515,#54516,#54517,#54518,#54519,#54520),(#54521,#54522,#54523,
#54524,#54525,#54526),(#54527,#54528,#54529,#54530,#54531,#54532),(#54533,
#54534,#54535,#54536,#54537,#54538),(#54539,#54540,#54541,#54542,#54543,
#54544),(#54545,#54546,#54547,#54548,#54549,#54550),(#54551,#54552,#54553,
#54554,#54555,#54556),(#54557,#54558,#54559,#54560,#54561,#54562)),
 .UNSPECIFIED.,.F.,.F.,.F.,(6,3,6),(6,6),(1.01054285509,1.23011259501,1.32384910338),
(0.,1.),.UNSPECIFIED.);
#924=B_SPLINE_SURFACE_WITH_KNOTS('',5,5,((#54564,#54565,#54566,#54567,#54568,
#54569),(#54570,#54571,#54572,#54573,#54574,#54575),(#54576,#54577,#54578,
#54579,#54580,#54581),(#54582,#54583,#54584,#54585,#54586,#54587),(#54588,
#54589,#54590,#54591,#54592,#54593),(#54594,#54595,#54596,#54597,#54598,
#54599),(#54600,#54601,#54602,#54603,#54604,#54605),(#54606,#54607,#54608,
#54609,#54610,#54611),(#54612,#54613,#54614,#54615,#54616,#54617),(#54618,
#54619,#54620,#54621,#54622,#54623),(#54624,#54625,#54626,#54627,#54628,
#54629),(#54630,#54631,#54632,#54633,#54634,#54635)),.UNSPECIFIED.,.F.,
 .F.,.F.,(6,3,3,6),(6,6),(4.46364567829,9.98301756848,13.6615164274,17.5757040899),
(0.,1.),.UNSPECIFIED.);
#925=B_SPLINE_SURFACE_WITH_KNOTS('',5,5,((#54637,#54638,#54639,#54640,#54641,
#54642),(#54643,#54644,#54645,#54646,#54647,#54648),(#54649,#54650,#54651,
#54652,#54653,#54654),(#54655,#54656,#54657,#54658,#54659,#54660),(#54661,
#54662,#54663,#54664,#54665,#54666),(#54667,#54668,#54669,#54670,#54671,
#54672)),.UNSPECIFIED.,.F.,.F.,.F.,(6,6),(6,6),(0.994217933968,1.222355190019),
(-0.00106176792899955,1.00011077696173),.UNSPECIFIED.);
#926=B_SPLINE_SURFACE_WITH_KNOTS('',5,5,((#54674,#54675,#54676,#54677,#54678,
#54679),(#54680,#54681,#54682,#54683,#54684,#54685),(#54686,#54687,#54688,
#54689,#54690,#54691),(#54692,#54693,#54694,#54695,#54696,#54697),(#54698,
#54699,#54700,#54701,#54702,#54703),(#54704,#54705,#54706,#54707,#54708,
#54709)),.UNSPECIFIED.,.F.,.F.,.F.,(6,6),(6,6),(1.40817420416,1.45205022904),
(0.,1.),.UNSPECIFIED.);
#927=B_SPLINE_SURFACE_WITH_KNOTS('',5,5,((#54712,#54713,#54714,#54715,#54716,
#54717),(#54718,#54719,#54720,#54721,#54722,#54723),(#54724,#54725,#54726,
#54727,#54728,#54729),(#54730,#54731,#54732,#54733,#54734,#54735),(#54736,
#54737,#54738,#54739,#54740,#54741),(#54742,#54743,#54744,#54745,#54746,
#54747),(#54748,#54749,#54750,#54751,#54752,#54753),(#54754,#54755,#54756,
#54757,#54758,#54759),(#54760,#54761,#54762,#54763,#54764,#54765)),
 .UNSPECIFIED.,.F.,.F.,.F.,(6,3,6),(6,6),(0.342430056326,0.787545489389,
1.14838178471),(0.,1.),.UNSPECIFIED.);
#928=B_SPLINE_SURFACE_WITH_KNOTS('',5,5,((#54767,#54768,#54769,#54770,#54771,
#54772),(#54773,#54774,#54775,#54776,#54777,#54778),(#54779,#54780,#54781,
#54782,#54783,#54784),(#54785,#54786,#54787,#54788,#54789,#54790),(#54791,
#54792,#54793,#54794,#54795,#54796),(#54797,#54798,#54799,#54800,#54801,
#54802)),.UNSPECIFIED.,.F.,.F.,.F.,(6,6),(6,6),(1.036743613,1.10280574369),
(0.,1.),.UNSPECIFIED.);
#929=B_SPLINE_SURFACE_WITH_KNOTS('',5,1,((#55071,#55072),(#55073,#55074),
(#55075,#55076),(#55077,#55078),(#55079,#55080),(#55081,#55082)),
 .UNSPECIFIED.,.F.,.F.,.F.,(6,6),(2,2),(0.,3.0373684949),(0.,3.10437234689),
 .UNSPECIFIED.);
#930=B_SPLINE_SURFACE_WITH_KNOTS('',5,1,((#55109,#55110),(#55111,#55112),
(#55113,#55114),(#55115,#55116),(#55117,#55118),(#55119,#55120)),
 .UNSPECIFIED.,.F.,.F.,.F.,(6,6),(2,2),(0.,0.392615054569),(0.,3.10437234689),
 .UNSPECIFIED.);
#931=B_SPLINE_SURFACE_WITH_KNOTS('',5,1,((#55137,#55138),(#55139,#55140),
(#55141,#55142),(#55143,#55144),(#55145,#55146),(#55147,#55148)),
 .UNSPECIFIED.,.F.,.F.,.F.,(6,6),(2,2),(0.,0.226010362356),(0.,3.10437234689),
 .UNSPECIFIED.);
#932=B_SPLINE_SURFACE_WITH_KNOTS('',5,1,((#55159,#55160),(#55161,#55162),
(#55163,#55164),(#55165,#55166),(#55167,#55168),(#55169,#55170)),
 .UNSPECIFIED.,.F.,.F.,.F.,(6,6),(2,2),(0.,0.600083611309),(0.,3.10437234689),
 .UNSPECIFIED.);
#933=B_SPLINE_SURFACE_WITH_KNOTS('',5,1,((#55181,#55182),(#55183,#55184),
(#55185,#55186),(#55187,#55188),(#55189,#55190),(#55191,#55192),(#55193,
#55194),(#55195,#55196),(#55197,#55198),(#55199,#55200),(#55201,#55202),
(#55203,#55204)),.UNSPECIFIED.,.F.,.F.,.F.,(6,3,3,6),(2,2),(0.,2.83532528452,
6.09533201542,9.83397913335),(0.,3.10437234689),.UNSPECIFIED.);
#934=B_SPLINE_SURFACE_WITH_KNOTS('',5,1,((#55271,#55272),(#55273,#55274),
(#55275,#55276),(#55277,#55278),(#55279,#55280),(#55281,#55282)),
 .UNSPECIFIED.,.F.,.F.,.F.,(6,6),(2,2),(0.,0.224378834114),(0.,3.10437234689),
 .UNSPECIFIED.);
#935=B_SPLINE_SURFACE_WITH_KNOTS('',5,1,((#55291,#55292),(#55293,#55294),
(#55295,#55296),(#55297,#55298),(#55299,#55300),(#55301,#55302),(#55303,
#55304),(#55305,#55306),(#55307,#55308)),.UNSPECIFIED.,.F.,.F.,.F.,(6,3,
6),(2,2),(0.,2.10936312981,4.22279623369),(0.,3.10437234689),
 .UNSPECIFIED.);
#936=B_SPLINE_SURFACE_WITH_KNOTS('',5,1,((#55351,#55352),(#55353,#55354),
(#55355,#55356),(#55357,#55358),(#55359,#55360),(#55361,#55362)),
 .UNSPECIFIED.,.F.,.F.,.F.,(6,6),(2,2),(0.,1.84821844080963),(0.,3.10437234689),
 .UNSPECIFIED.);
#937=B_SPLINE_SURFACE_WITH_KNOTS('',5,1,((#55396,#55397),(#55398,#55399),
(#55400,#55401),(#55402,#55403),(#55404,#55405),(#55406,#55407)),
 .UNSPECIFIED.,.F.,.F.,.F.,(6,6),(2,2),(0.,0.482067685837),(0.,3.10437234689),
 .UNSPECIFIED.);
#938=B_SPLINE_SURFACE_WITH_KNOTS('',5,1,((#55411,#55412),(#55413,#55414),
(#55415,#55416),(#55417,#55418),(#55419,#55420),(#55421,#55422),(#55423,
#55424),(#55425,#55426),(#55427,#55428),(#55429,#55430),(#55431,#55432),
(#55433,#55434)),.UNSPECIFIED.,.F.,.F.,.F.,(6,3,3,6),(2,2),(0.,0.629547398659,
1.2493532974,1.86132516749),(0.,3.10437234689),.UNSPECIFIED.);
#939=B_SPLINE_SURFACE_WITH_KNOTS('',5,1,((#55504,#55505),(#55506,#55507),
(#55508,#55509),(#55510,#55511),(#55512,#55513),(#55514,#55515)),
 .UNSPECIFIED.,.F.,.F.,.F.,(6,6),(2,2),(0.,0.2489231439),(0.,3.10437234689),
 .UNSPECIFIED.);
#940=B_SPLINE_SURFACE_WITH_KNOTS('',5,1,((#55517,#55518),(#55519,#55520),
(#55521,#55522),(#55523,#55524),(#55525,#55526),(#55527,#55528)),
 .UNSPECIFIED.,.F.,.F.,.F.,(6,6),(2,2),(0.,3.0373684949),(0.,3.10437234689),
 .UNSPECIFIED.);
#941=B_SPLINE_SURFACE_WITH_KNOTS('',5,1,((#55553,#55554),(#55555,#55556),
(#55557,#55558),(#55559,#55560),(#55561,#55562),(#55563,#55564)),
 .UNSPECIFIED.,.F.,.F.,.F.,(6,6),(2,2),(0.,0.392615054569),(0.,3.10437234689),
 .UNSPECIFIED.);
#942=B_SPLINE_SURFACE_WITH_KNOTS('',5,5,((#55575,#55576,#55577,#55578,#55579,
#55580),(#55581,#55582,#55583,#55584,#55585,#55586),(#55587,#55588,#55589,
#55590,#55591,#55592),(#55593,#55594,#55595,#55596,#55597,#55598),(#55599,
#55600,#55601,#55602,#55603,#55604),(#55605,#55606,#55607,#55608,#55609,
#55610),(#55611,#55612,#55613,#55614,#55615,#55616),(#55617,#55618,#55619,
#55620,#55621,#55622),(#55623,#55624,#55625,#55626,#55627,#55628)),
 .UNSPECIFIED.,.F.,.F.,.F.,(6,3,6),(6,6),(8.63627991204,12.3201261581,17.1386583361),
(0.,0.3),.UNSPECIFIED.);
#943=B_SPLINE_SURFACE_WITH_KNOTS('',5,5,((#55795,#55796,#55797,#55798,#55799,
#55800),(#55801,#55802,#55803,#55804,#55805,#55806),(#55807,#55808,#55809,
#55810,#55811,#55812),(#55813,#55814,#55815,#55816,#55817,#55818),(#55819,
#55820,#55821,#55822,#55823,#55824),(#55825,#55826,#55827,#55828,#55829,
#55830),(#55831,#55832,#55833,#55834,#55835,#55836),(#55837,#55838,#55839,
#55840,#55841,#55842),(#55843,#55844,#55845,#55846,#55847,#55848)),
 .UNSPECIFIED.,.F.,.F.,.F.,(6,3,6),(6,6),(1.56090158029,2.52299916049,2.93530749734),
(0.,0.3),.UNSPECIFIED.);
#944=B_SPLINE_SURFACE_WITH_KNOTS('',5,5,((#55877,#55878,#55879,#55880,#55881,
#55882),(#55883,#55884,#55885,#55886,#55887,#55888),(#55889,#55890,#55891,
#55892,#55893,#55894),(#55895,#55896,#55897,#55898,#55899,#55900),(#55901,
#55902,#55903,#55904,#55905,#55906),(#55907,#55908,#55909,#55910,#55911,
#55912),(#55913,#55914,#55915,#55916,#55917,#55918),(#55919,#55920,#55921,
#55922,#55923,#55924),(#55925,#55926,#55927,#55928,#55929,#55930)),
 .UNSPECIFIED.,.F.,.F.,.F.,(6,3,6),(6,6),(3.22008961045,5.63866638969,8.97249770267),
(0.,0.3),.UNSPECIFIED.);
#945=B_SPLINE_SURFACE_WITH_KNOTS('',5,5,((#55998,#55999,#56000,#56001,#56002,
#56003),(#56004,#56005,#56006,#56007,#56008,#56009),(#56010,#56011,#56012,
#56013,#56014,#56015),(#56016,#56017,#56018,#56019,#56020,#56021),(#56022,
#56023,#56024,#56025,#56026,#56027),(#56028,#56029,#56030,#56031,#56032,
#56033),(#56034,#56035,#56036,#56037,#56038,#56039),(#56040,#56041,#56042,
#56043,#56044,#56045),(#56046,#56047,#56048,#56049,#56050,#56051)),
 .UNSPECIFIED.,.F.,.F.,.F.,(6,3,6),(6,6),(1.72939840805139,1.80499037738,
1.87215083229958),(-2.7802799580615E-5,0.3),.UNSPECIFIED.);
#946=B_SPLINE_SURFACE_WITH_KNOTS('',5,5,((#56388,#56389,#56390,#56391,#56392,
#56393),(#56394,#56395,#56396,#56397,#56398,#56399),(#56400,#56401,#56402,
#56403,#56404,#56405),(#56406,#56407,#56408,#56409,#56410,#56411),(#56412,
#56413,#56414,#56415,#56416,#56417),(#56418,#56419,#56420,#56421,#56422,
#56423)),.UNSPECIFIED.,.F.,.F.,.F.,(6,6),(6,6),(1.03921348145,1.16363378049),
(0.,0.3),.UNSPECIFIED.);
#947=B_SPLINE_SURFACE_WITH_KNOTS('',5,5,((#56432,#56433,#56434,#56435,#56436,
#56437),(#56438,#56439,#56440,#56441,#56442,#56443),(#56444,#56445,#56446,
#56447,#56448,#56449),(#56450,#56451,#56452,#56453,#56454,#56455),(#56456,
#56457,#56458,#56459,#56460,#56461),(#56462,#56463,#56464,#56465,#56466,
#56467)),.UNSPECIFIED.,.F.,.F.,.F.,(6,6),(6,6),(0.594536305137334,3.46674155179467),
(-0.000626841014666089,0.3),.UNSPECIFIED.);
#948=B_SPLINE_SURFACE_WITH_KNOTS('',5,5,((#56486,#56487,#56488,#56489,#56490,
#56491),(#56492,#56493,#56494,#56495,#56496,#56497),(#56498,#56499,#56500,
#56501,#56502,#56503),(#56504,#56505,#56506,#56507,#56508,#56509),(#56510,
#56511,#56512,#56513,#56514,#56515),(#56516,#56517,#56518,#56519,#56520,
#56521)),.UNSPECIFIED.,.F.,.F.,.F.,(6,6),(6,6),(3.1034218264,3.1199806069),
(0.,0.3),.UNSPECIFIED.);
#949=B_SPLINE_SURFACE_WITH_KNOTS('',5,5,((#56525,#56526,#56527,#56528,#56529,
#56530),(#56531,#56532,#56533,#56534,#56535,#56536),(#56537,#56538,#56539,
#56540,#56541,#56542),(#56543,#56544,#56545,#56546,#56547,#56548),(#56549,
#56550,#56551,#56552,#56553,#56554),(#56555,#56556,#56557,#56558,#56559,
#56560),(#56561,#56562,#56563,#56564,#56565,#56566),(#56567,#56568,#56569,
#56570,#56571,#56572),(#56573,#56574,#56575,#56576,#56577,#56578)),
 .UNSPECIFIED.,.F.,.F.,.F.,(6,3,6),(6,6),(0.0737511682725,0.240560274088,
0.36600685554),(0.,0.3),.UNSPECIFIED.);
#950=B_SPLINE_SURFACE_WITH_KNOTS('',4,5,((#56590,#56591,#56592,#56593,#56594,
#56595),(#56596,#56597,#56598,#56599,#56600,#56601),(#56602,#56603,#56604,
#56605,#56606,#56607),(#56608,#56609,#56610,#56611,#56612,#56613),(#56614,
#56615,#56616,#56617,#56618,#56619)),.UNSPECIFIED.,.F.,.F.,.F.,(5,5),(6,
6),(1.03670984253,1.04687754685),(0.,0.3),.UNSPECIFIED.);
#951=B_SPLINE_SURFACE_WITH_KNOTS('',5,5,((#56626,#56627,#56628,#56629,#56630,
#56631),(#56632,#56633,#56634,#56635,#56636,#56637),(#56638,#56639,#56640,
#56641,#56642,#56643),(#56644,#56645,#56646,#56647,#56648,#56649),(#56650,
#56651,#56652,#56653,#56654,#56655),(#56656,#56657,#56658,#56659,#56660,
#56661),(#56662,#56663,#56664,#56665,#56666,#56667),(#56668,#56669,#56670,
#56671,#56672,#56673),(#56674,#56675,#56676,#56677,#56678,#56679)),
 .UNSPECIFIED.,.F.,.F.,.F.,(6,3,6),(6,6),(1.01756015018,3.02586880249,6.44209971341),
(0.,0.3),.UNSPECIFIED.);
#952=B_SPLINE_SURFACE_WITH_KNOTS('',5,5,((#56691,#56692,#56693,#56694,#56695,
#56696),(#56697,#56698,#56699,#56700,#56701,#56702),(#56703,#56704,#56705,
#56706,#56707,#56708),(#56709,#56710,#56711,#56712,#56713,#56714),(#56715,
#56716,#56717,#56718,#56719,#56720),(#56721,#56722,#56723,#56724,#56725,
#56726),(#56727,#56728,#56729,#56730,#56731,#56732),(#56733,#56734,#56735,
#56736,#56737,#56738),(#56739,#56740,#56741,#56742,#56743,#56744)),
 .UNSPECIFIED.,.F.,.F.,.F.,(6,3,6),(6,6),(1.01756015018,3.02586880249,6.44209971341),
(0.,0.3),.UNSPECIFIED.);
#953=B_SPLINE_SURFACE_WITH_KNOTS('',4,5,((#56844,#56845,#56846,#56847,#56848,
#56849),(#56850,#56851,#56852,#56853,#56854,#56855),(#56856,#56857,#56858,
#56859,#56860,#56861),(#56862,#56863,#56864,#56865,#56866,#56867),(#56868,
#56869,#56870,#56871,#56872,#56873)),.UNSPECIFIED.,.F.,.F.,.F.,(5,5),(6,
6),(1.03670984253,1.04687754685),(0.,0.3),.UNSPECIFIED.);
#954=B_SPLINE_SURFACE_WITH_KNOTS('',5,5,((#56880,#56881,#56882,#56883,#56884,
#56885),(#56886,#56887,#56888,#56889,#56890,#56891),(#56892,#56893,#56894,
#56895,#56896,#56897),(#56898,#56899,#56900,#56901,#56902,#56903),(#56904,
#56905,#56906,#56907,#56908,#56909),(#56910,#56911,#56912,#56913,#56914,
#56915),(#56916,#56917,#56918,#56919,#56920,#56921),(#56922,#56923,#56924,
#56925,#56926,#56927),(#56928,#56929,#56930,#56931,#56932,#56933)),
 .UNSPECIFIED.,.F.,.F.,.F.,(6,3,6),(6,6),(0.0737511682725,0.240560274088,
0.36600685554),(0.,0.3),.UNSPECIFIED.);
#955=B_SPLINE_SURFACE_WITH_KNOTS('',5,5,((#56958,#56959,#56960,#56961,#56962,
#56963),(#56964,#56965,#56966,#56967,#56968,#56969),(#56970,#56971,#56972,
#56973,#56974,#56975),(#56976,#56977,#56978,#56979,#56980,#56981),(#56982,
#56983,#56984,#56985,#56986,#56987),(#56988,#56989,#56990,#56991,#56992,
#56993)),.UNSPECIFIED.,.F.,.F.,.F.,(6,6),(6,6),(3.1034218264,3.1199806069),
(0.,0.3),.UNSPECIFIED.);
#956=B_SPLINE_SURFACE_WITH_KNOTS('',5,5,((#56997,#56998,#56999,#57000,#57001,
#57002),(#57003,#57004,#57005,#57006,#57007,#57008),(#57009,#57010,#57011,
#57012,#57013,#57014),(#57015,#57016,#57017,#57018,#57019,#57020),(#57021,
#57022,#57023,#57024,#57025,#57026),(#57027,#57028,#57029,#57030,#57031,
#57032)),.UNSPECIFIED.,.F.,.F.,.F.,(6,6),(6,6),(0.594419717825406,3.46685813910659),
(-0.000743428326593711,0.3),.UNSPECIFIED.);
#957=B_SPLINE_SURFACE_WITH_KNOTS('',5,5,((#57039,#57040,#57041,#57042,#57043,
#57044),(#57045,#57046,#57047,#57048,#57049,#57050),(#57051,#57052,#57053,
#57054,#57055,#57056),(#57057,#57058,#57059,#57060,#57061,#57062),(#57063,
#57064,#57065,#57066,#57067,#57068),(#57069,#57070,#57071,#57072,#57073,
#57074)),.UNSPECIFIED.,.F.,.F.,.F.,(6,6),(6,6),(1.03921348145,1.16363378049),
(0.,0.3),.UNSPECIFIED.);
#958=B_SPLINE_SURFACE_WITH_KNOTS('',5,5,((#57092,#57093,#57094,#57095,#57096,
#57097),(#57098,#57099,#57100,#57101,#57102,#57103),(#57104,#57105,#57106,
#57107,#57108,#57109),(#57110,#57111,#57112,#57113,#57114,#57115),(#57116,
#57117,#57118,#57119,#57120,#57121),(#57122,#57123,#57124,#57125,#57126,
#57127),(#57128,#57129,#57130,#57131,#57132,#57133),(#57134,#57135,#57136,
#57137,#57138,#57139),(#57140,#57141,#57142,#57143,#57144,#57145)),
 .UNSPECIFIED.,.F.,.F.,.F.,(6,3,6),(6,6),(1.72942608575,1.80499037738,1.8721230295),
(0.,0.3),.UNSPECIFIED.);
#959=B_SPLINE_SURFACE_WITH_KNOTS('',5,5,((#57164,#57165,#57166,#57167,#57168,
#57169),(#57170,#57171,#57172,#57173,#57174,#57175),(#57176,#57177,#57178,
#57179,#57180,#57181),(#57182,#57183,#57184,#57185,#57186,#57187),(#57188,
#57189,#57190,#57191,#57192,#57193),(#57194,#57195,#57196,#57197,#57198,
#57199),(#57200,#57201,#57202,#57203,#57204,#57205),(#57206,#57207,#57208,
#57209,#57210,#57211),(#57212,#57213,#57214,#57215,#57216,#57217)),
 .UNSPECIFIED.,.F.,.F.,.F.,(6,3,6),(6,6),(3.22008961045,5.63866638969,8.97249770267),
(0.,0.3),.UNSPECIFIED.);
#960=B_SPLINE_SURFACE_WITH_KNOTS('',5,5,((#57269,#57270,#57271,#57272,#57273,
#57274),(#57275,#57276,#57277,#57278,#57279,#57280),(#57281,#57282,#57283,
#57284,#57285,#57286),(#57287,#57288,#57289,#57290,#57291,#57292),(#57293,
#57294,#57295,#57296,#57297,#57298),(#57299,#57300,#57301,#57302,#57303,
#57304),(#57305,#57306,#57307,#57308,#57309,#57310),(#57311,#57312,#57313,
#57314,#57315,#57316),(#57317,#57318,#57319,#57320,#57321,#57322)),
 .UNSPECIFIED.,.F.,.F.,.F.,(6,3,6),(6,6),(1.56090158029,2.52299916049,2.93530749734),
(0.,0.3),.UNSPECIFIED.);
#961=B_SPLINE_SURFACE_WITH_KNOTS('',5,5,((#57341,#57342,#57343,#57344,#57345,
#57346),(#57347,#57348,#57349,#57350,#57351,#57352),(#57353,#57354,#57355,
#57356,#57357,#57358),(#57359,#57360,#57361,#57362,#57363,#57364),(#57365,
#57366,#57367,#57368,#57369,#57370),(#57371,#57372,#57373,#57374,#57375,
#57376),(#57377,#57378,#57379,#57380,#57381,#57382),(#57383,#57384,#57385,
#57386,#57387,#57388),(#57389,#57390,#57391,#57392,#57393,#57394)),
 .UNSPECIFIED.,.F.,.F.,.F.,(6,3,6),(6,6),(8.63480411392599,12.3201261581,
17.1386583361),(0.,0.301475798114014),.UNSPECIFIED.);
#962=B_SPLINE_SURFACE_WITH_KNOTS('',5,5,((#57528,#57529,#57530,#57531,#57532,
#57533),(#57534,#57535,#57536,#57537,#57538,#57539),(#57540,#57541,#57542,
#57543,#57544,#57545),(#57546,#57547,#57548,#57549,#57550,#57551),(#57552,
#57553,#57554,#57555,#57556,#57557),(#57558,#57559,#57560,#57561,#57562,
#57563),(#57564,#57565,#57566,#57567,#57568,#57569),(#57570,#57571,#57572,
#57573,#57574,#57575),(#57576,#57577,#57578,#57579,#57580,#57581)),
 .UNSPECIFIED.,.F.,.F.,.F.,(6,3,6),(6,6),(-3.25426975736,0.,6.50853951471),
(0.,3.45067933061),.UNSPECIFIED.);
#963=B_SPLINE_SURFACE_WITH_KNOTS('',5,5,((#57612,#57613,#57614,#57615,#57616,
#57617),(#57618,#57619,#57620,#57621,#57622,#57623),(#57624,#57625,#57626,
#57627,#57628,#57629),(#57630,#57631,#57632,#57633,#57634,#57635),(#57636,
#57637,#57638,#57639,#57640,#57641),(#57642,#57643,#57644,#57645,#57646,
#57647),(#57648,#57649,#57650,#57651,#57652,#57653),(#57654,#57655,#57656,
#57657,#57658,#57659),(#57660,#57661,#57662,#57663,#57664,#57665)),
 .UNSPECIFIED.,.F.,.F.,.F.,(6,3,6),(6,6),(-3.25426975736,0.,6.50853951471),
(0.,3.45067933061),.UNSPECIFIED.);
#964=B_SPLINE_SURFACE_WITH_KNOTS('',5,1,((#57674,#57675),(#57676,#57677),
(#57678,#57679),(#57680,#57681),(#57682,#57683),(#57684,#57685)),
 .UNSPECIFIED.,.F.,.F.,.F.,(6,6),(2,2),(0.,1.06471780544),(0.,3.45067933061),
 .UNSPECIFIED.);
#965=B_SPLINE_SURFACE_WITH_KNOTS('',5,1,((#57689,#57690),(#57691,#57692),
(#57693,#57694),(#57695,#57696),(#57697,#57698),(#57699,#57700)),
 .UNSPECIFIED.,.F.,.F.,.F.,(6,6),(2,2),(0.,4.45911142417),(0.,3.45067933061),
 .UNSPECIFIED.);
#966=B_SPLINE_SURFACE_WITH_KNOTS('',5,1,((#57704,#57705),(#57706,#57707),
(#57708,#57709),(#57710,#57711),(#57712,#57713),(#57714,#57715)),
 .UNSPECIFIED.,.F.,.F.,.F.,(6,6),(2,2),(0.,0.261676985017),(0.,3.45067933061),
 .UNSPECIFIED.);
#967=B_SPLINE_SURFACE_WITH_KNOTS('',5,1,((#57719,#57720),(#57721,#57722),
(#57723,#57724),(#57725,#57726),(#57727,#57728),(#57729,#57730)),
 .UNSPECIFIED.,.F.,.F.,.F.,(6,6),(2,2),(0.,2.2409741083),(0.,3.45067933061),
 .UNSPECIFIED.);
#968=B_SPLINE_SURFACE_WITH_KNOTS('',5,1,((#57739,#57740),(#57741,#57742),
(#57743,#57744),(#57745,#57746),(#57747,#57748),(#57749,#57750)),
 .UNSPECIFIED.,.F.,.F.,.F.,(6,6),(2,2),(0.,0.230635297438),(0.,3.45067933061),
 .UNSPECIFIED.);
#969=B_SPLINE_SURFACE_WITH_KNOTS('',5,1,((#57754,#57755),(#57756,#57757),
(#57758,#57759),(#57760,#57761),(#57762,#57763),(#57764,#57765)),
 .UNSPECIFIED.,.F.,.F.,.F.,(6,6),(2,2),(0.,4.13278827108),(0.,3.45067933061),
 .UNSPECIFIED.);
#970=B_SPLINE_SURFACE_WITH_KNOTS('',5,1,((#57769,#57770),(#57771,#57772),
(#57773,#57774),(#57775,#57776),(#57777,#57778),(#57779,#57780)),
 .UNSPECIFIED.,.F.,.F.,.F.,(6,6),(2,2),(0.,4.13278827108),(0.,3.45067933061),
 .UNSPECIFIED.);
#971=B_SPLINE_SURFACE_WITH_KNOTS('',5,1,((#57784,#57785),(#57786,#57787),
(#57788,#57789),(#57790,#57791),(#57792,#57793),(#57794,#57795)),
 .UNSPECIFIED.,.F.,.F.,.F.,(6,6),(2,2),(0.,0.230635297438),(0.,3.45067933061),
 .UNSPECIFIED.);
#972=B_SPLINE_SURFACE_WITH_KNOTS('',5,1,((#57799,#57800),(#57801,#57802),
(#57803,#57804),(#57805,#57806),(#57807,#57808),(#57809,#57810)),
 .UNSPECIFIED.,.F.,.F.,.F.,(6,6),(2,2),(0.,2.2409741083),(0.,3.45067933061),
 .UNSPECIFIED.);
#973=B_SPLINE_SURFACE_WITH_KNOTS('',5,1,((#57819,#57820),(#57821,#57822),
(#57823,#57824),(#57825,#57826),(#57827,#57828),(#57829,#57830)),
 .UNSPECIFIED.,.F.,.F.,.F.,(6,6),(2,2),(0.,0.261676985017),(0.,3.45067933061),
 .UNSPECIFIED.);
#974=B_SPLINE_SURFACE_WITH_KNOTS('',5,1,((#57834,#57835),(#57836,#57837),
(#57838,#57839),(#57840,#57841),(#57842,#57843),(#57844,#57845)),
 .UNSPECIFIED.,.F.,.F.,.F.,(6,6),(2,2),(0.,4.45911142417),(0.,3.45067933061),
 .UNSPECIFIED.);
#975=B_SPLINE_SURFACE_WITH_KNOTS('',5,1,((#57849,#57850),(#57851,#57852),
(#57853,#57854),(#57855,#57856),(#57857,#57858),(#57859,#57860)),
 .UNSPECIFIED.,.F.,.F.,.F.,(6,6),(2,2),(0.,1.06471780544),(0.,3.45067933061),
 .UNSPECIFIED.);
#1254=FACE_BOUND('',#5426,.T.);
#1255=FACE_BOUND('',#5427,.T.);
#1256=FACE_BOUND('',#5428,.T.);
#1257=FACE_BOUND('',#5633,.T.);
#1258=FACE_BOUND('',#5711,.T.);
#1259=FACE_BOUND('',#5712,.T.);
#1260=FACE_BOUND('',#5713,.T.);
#1261=FACE_BOUND('',#5722,.T.);
#1332=B_SPLINE_CURVE_WITH_KNOTS('',5,(#49225,#49226,#49227,#49228,#49229,
#49230,#49231),.UNSPECIFIED.,.F.,.F.,(6,1,6),(0.,0.465407720561711,1.),
 .UNSPECIFIED.);
#1333=B_SPLINE_CURVE_WITH_KNOTS('',5,(#49233,#49234,#49235,#49236,#49237,
#49238),.UNSPECIFIED.,.F.,.F.,(6,6),(0.,0.788840280269),.UNSPECIFIED.);
#1334=B_SPLINE_CURVE_WITH_KNOTS('',5,(#49240,#49241,#49242,#49243,#49244,
#49245,#49246,#49247,#49248,#49249,#49250),.UNSPECIFIED.,.F.,.F.,(6,3,1,
1,6),(0.,0.151641330465487,0.494687846976795,0.919150815604558,1.),
 .UNSPECIFIED.);
#1335=B_SPLINE_CURVE_WITH_KNOTS('',5,(#49252,#49253,#49254,#49255,#49256,
#49257),.UNSPECIFIED.,.F.,.F.,(6,6),(0.,1.62525620495),.UNSPECIFIED.);
#1336=B_SPLINE_CURVE_WITH_KNOTS('',5,(#49259,#49260,#49261,#49262,#49263,
#49264,#49265,#49266,#49267,#49268,#49269),.UNSPECIFIED.,.F.,.F.,(6,2,1,
1,1,6),(0.,0.232559611743824,0.537888788088502,0.750633611657941,0.946930649753588,
1.),.UNSPECIFIED.);
#1337=B_SPLINE_CURVE_WITH_KNOTS('',5,(#49276,#49277,#49278,#49279,#49280,
#49281,#49282,#49283),.UNSPECIFIED.,.F.,.F.,(6,2,6),(0.,0.422457434925888,
1.),.UNSPECIFIED.);
#1338=B_SPLINE_CURVE_WITH_KNOTS('',5,(#49305,#49306,#49307,#49308,#49309,
#49310,#49311,#49312,#49313,#49314,#49315,#49316,#49317,#49318,#49319,#49320,
#49321,#49322),.UNSPECIFIED.,.F.,.F.,(6,3,3,3,3,6),(0.465128126763,3.42050470566,
7.30063973795,10.0042092191,12.4987596036,13.1731669678),.UNSPECIFIED.);
#1339=B_SPLINE_CURVE_WITH_KNOTS('',5,(#49324,#49325,#49326,#49327,#49328,
#49329),.UNSPECIFIED.,.F.,.F.,(6,6),(0.,1.62525620495),.UNSPECIFIED.);
#1340=B_SPLINE_CURVE_WITH_KNOTS('',5,(#49331,#49332,#49333,#49334,#49335,
#49336,#49337,#49338,#49339,#49340,#49341,#49342,#49343,#49344,#49345),
 .UNSPECIFIED.,.F.,.F.,(6,3,3,3,6),(0.617889185003,0.915206541473,1.58780472511,
2.42003303229,2.57855093571),.UNSPECIFIED.);
#1341=B_SPLINE_CURVE_WITH_KNOTS('',5,(#49347,#49348,#49349,#49350,#49351,
#49352),.UNSPECIFIED.,.F.,.F.,(6,6),(0.,0.788840280269),.UNSPECIFIED.);
#1342=B_SPLINE_CURVE_WITH_KNOTS('',3,(#49354,#49355,#49356,#49357),
 .UNSPECIFIED.,.F.,.F.,(4,4),(0.,1.),.UNSPECIFIED.);
#1343=B_SPLINE_CURVE_WITH_KNOTS('',3,(#49361,#49362,#49363,#49364),
 .UNSPECIFIED.,.F.,.F.,(4,4),(0.,1.),.UNSPECIFIED.);
#1344=B_SPLINE_CURVE_WITH_KNOTS('',5,(#49388,#49389,#49390,#49391,#49392,
#49393,#49394,#49395,#49396),.UNSPECIFIED.,.F.,.F.,(6,3,6),(0.,0.500481905098514,
1.),.UNSPECIFIED.);
#1345=B_SPLINE_CURVE_WITH_KNOTS('',3,(#49400,#49401,#49402,#49403,#49404,
#49405,#49406,#49407,#49408,#49409),.UNSPECIFIED.,.F.,.F.,(4,3,3,4),(-2.46410111513,
-2.43212843610953,-2.39098596142,-2.37851323355),.UNSPECIFIED.);
#1346=B_SPLINE_CURVE_WITH_KNOTS('',3,(#49410,#49411,#49412,#49413,#49414,
#49415,#49416,#49417,#49418,#49419,#49420,#49421,#49422,#49423,#49424,#49425,
#49426,#49427,#49428,#49429,#49430,#49431,#49432,#49433,#49434,#49435,#49436,
#49437,#49438,#49439,#49440,#49441,#49442,#49443,#49444,#49445,#49446,#49447,
#49448,#49449,#49450,#49451,#49452),.UNSPECIFIED.,.F.,.F.,(4,3,3,3,3,3,
3,3,3,3,3,3,3,3,4),(0.,0.0613221810056141,0.125866562481823,0.192962198900169,
0.263336451623022,0.341802092378546,0.427968116931692,0.536199508330899,
0.56788778905896,0.661002984718601,0.746254481470477,0.828376996970244,
0.907920904739906,0.984520534711008,1.),.UNSPECIFIED.);
#1347=B_SPLINE_CURVE_WITH_KNOTS('',3,(#49487,#49488,#49489,#49490,#49491,
#49492,#49493,#49494,#49495,#49496,#49497,#49498,#49499,#49500,#49501,#49502,
#49503,#49504,#49505,#49506,#49507,#49508,#49509,#49510,#49511,#49512,#49513,
#49514,#49515,#49516,#49517,#49518,#49519,#49520),.UNSPECIFIED.,.F.,.F.,
(4,3,3,3,3,3,3,3,3,3,3,4),(0.,0.0987514676261084,0.196101602166033,0.2928935924342,
0.389205363491127,0.421433182784012,0.517619219660985,0.613998257361256,
0.711154034512961,0.808967652077894,0.908370062273473,1.),.UNSPECIFIED.);
#1348=B_SPLINE_CURVE_WITH_KNOTS('',5,(#49526,#49527,#49528,#49529,#49530,
#49531,#49532,#49533,#49534),.UNSPECIFIED.,.F.,.F.,(6,3,6),(0.,0.571293900064368,
1.),.UNSPECIFIED.);
#1349=B_SPLINE_CURVE_WITH_KNOTS('',3,(#49546,#49547,#49548,#49549,#49550,
#49551,#49552,#49553,#49554,#49555,#49556,#49557,#49558,#49559,#49560,#49561,
#49562,#49563,#49564,#49565,#49566,#49567,#49568,#49569,#49570,#49571,#49572,
#49573,#49574,#49575,#49576,#49577,#49578,#49579,#49580,#49581,#49582,#49583,
#49584,#49585),.UNSPECIFIED.,.F.,.F.,(4,3,3,3,3,3,3,3,3,3,3,3,3,4),(0.342430056326,
0.416647889440572,0.493342454420148,0.569706842465,0.648977821089767,0.726755174830412,
0.787545489389,0.864698238944471,0.942373129697395,1.0113837312,1.09481342684991,
1.13043704811,1.14340426682165,1.14838178471),.UNSPECIFIED.);
#1350=B_SPLINE_CURVE_WITH_KNOTS('',3,(#49626,#49627,#49628,#49629,#49630,
#49631,#49632,#49633,#49634,#49635,#49636,#49637,#49638,#49639,#49640,#49641,
#49642,#49643,#49644,#49645,#49646,#49647,#49648,#49649,#49650,#49651,#49652,
#49653,#49654,#49655,#49656,#49657,#49658,#49659,#49660,#49661,#49662,#49663,
#49664,#49665,#49666,#49667,#49668),.UNSPECIFIED.,.F.,.F.,(4,3,3,3,3,3,
3,3,3,3,3,3,3,3,4),(0.,0.0615954828555703,0.126643630853992,0.19444062384319,
0.265752116217026,0.345130620933528,0.430362574402989,0.517900008063448,
0.56788778905896,0.648999236771598,0.731976639456588,0.810477923749653,
0.885206012171236,0.955092587390329,1.),.UNSPECIFIED.);
#1351=B_SPLINE_CURVE_WITH_KNOTS('',3,(#49672,#49673,#49674,#49675,#49676,
#49677,#49678,#49679,#49680,#49681,#49682,#49683,#49684,#49685,#49686,#49687,
#49688,#49689,#49690,#49691,#49692,#49693,#49694,#49695,#49696,#49697,#49698,
#49699,#49700,#49701,#49702,#49703,#49704,#49705,#49706,#49707,#49708,#49709,
#49710,#49711,#49712,#49713,#49714,#49715,#49716,#49717,#49718,#49719,#49720,
#49721,#49722,#49723,#49724,#49725,#49726,#49727,#49728,#49729,#49730,#49731,
#49732,#49733,#49734,#49735,#49736,#49737,#49738,#49739,#49740,#49741,#49742,
#49743,#49744),.UNSPECIFIED.,.F.,.F.,(4,3,3,3,3,3,3,3,3,3,3,3,3,3,3,3,3,
3,3,3,3,3,3,3,4),(0.,0.0579967491242001,0.114812082591792,0.170568659950085,
0.225368908089845,0.278879773402611,0.331734010550692,0.383645284356977,
0.420938628926706,0.491074429566194,0.5407475186248,0.583067918566761,0.62318719578254,
0.662334513633599,0.699082071276243,0.701481831484658,0.731160497591717,
0.762275003148169,0.796507016141887,0.833748546202765,0.875311409652074,
0.913808413863513,0.949129309301143,0.981275404426876,1.),.UNSPECIFIED.);
#1352=B_SPLINE_CURVE_WITH_KNOTS('',5,(#49761,#49762,#49763,#49764,#49765,
#49766,#49767,#49768,#49769,#49770,#49771,#49772,#49773,#49774,#49775,#49776,
#49777,#49778,#49779,#49780,#49781),.UNSPECIFIED.,.F.,.F.,(6,3,3,3,3,3,
6),(-2.96825275179,-2.92587181617,-2.2858594369,-1.59285457075,-0.896955996606,
-0.723663994252,-0.586327318555),.UNSPECIFIED.);
#1353=B_SPLINE_CURVE_WITH_KNOTS('',5,(#49782,#49783,#49784,#49785,#49786,
#49787,#49788,#49789,#49790),.UNSPECIFIED.,.F.,.F.,(6,3,6),(-2.46410111513,
-2.39098596142,-2.37851323355),.UNSPECIFIED.);
#1354=B_SPLINE_CURVE_WITH_KNOTS('',5,(#49824,#49825,#49826,#49827,#49828,
#49829),.UNSPECIFIED.,.F.,.F.,(6,6),(1.26425849888,1.32115953697),
 .UNSPECIFIED.);
#1355=B_SPLINE_CURVE_WITH_KNOTS('',5,(#49831,#49832,#49833,#49834,#49835,
#49836,#49837,#49838,#49839,#49840,#49841,#49842),.UNSPECIFIED.,.F.,.F.,
(6,3,3,6),(0.,0.204469498724444,0.476563204173844,1.),.UNSPECIFIED.);
#1356=B_SPLINE_CURVE_WITH_KNOTS('',3,(#49844,#49845,#49846,#49847,#49848,
#49849,#49850,#49851,#49852,#49853,#49854,#49855,#49856,#49857,#49858,#49859,
#49860,#49861,#49862,#49863,#49864,#49865,#49866,#49867,#49868,#49869,#49870,
#49871),.UNSPECIFIED.,.F.,.F.,(4,3,3,3,3,3,3,3,3,4),(0.734432475987,0.878942275291463,
1.02006954288573,1.13913894251985,1.16119681048,1.21800796315046,1.27362568942023,
1.32243285508689,1.32924341569,1.33983380059),.UNSPECIFIED.);
#1357=B_SPLINE_CURVE_WITH_KNOTS('',3,(#49888,#49889,#49890,#49891,#49892,
#49893,#49894,#49895,#49896,#49897,#49898,#49899,#49900,#49901,#49902,#49903,
#49904,#49905,#49906,#49907,#49908,#49909,#49910,#49911,#49912,#49913,#49914,
#49915),.UNSPECIFIED.,.F.,.F.,(4,3,3,3,3,3,3,3,3,4),(-0.449080636148,-0.386865408847563,
-0.322025197047738,-0.251338921065949,-0.174920549069412,-0.0882035124128814,
0.0321179319799293,0.11744275401646,0.190820231313568,0.223602276698668),
 .UNSPECIFIED.);
#1358=B_SPLINE_CURVE_WITH_KNOTS('',3,(#49916,#49917,#49918,#49919,#49920,
#49921,#49922,#49923,#49924,#49925,#49926,#49927,#49928,#49929,#49930,#49931),
 .UNSPECIFIED.,.F.,.F.,(4,3,3,3,3,4),(0.338318706278865,0.442835581668533,
0.499233337792,0.619722435757,0.632996657825859,0.636935495757),
 .UNSPECIFIED.);
#1359=B_SPLINE_CURVE_WITH_KNOTS('',5,(#49953,#49954,#49955,#49956,#49957,
#49958,#49959,#49960,#49961,#49962,#49963,#49964),.UNSPECIFIED.,.F.,.F.,
(6,3,3,6),(0.,0.256132634704352,0.563769826408177,1.),.UNSPECIFIED.);
#1360=B_SPLINE_CURVE_WITH_KNOTS('',3,(#49965,#49966,#49967,#49968,#49969,
#49970,#49971,#49972,#49973,#49974),.UNSPECIFIED.,.F.,.F.,(4,3,3,4),(-0.0251761006649752,
-0.0188988511851622,-0.0125941833993852,0.),.UNSPECIFIED.);
#1361=B_SPLINE_CURVE_WITH_KNOTS('',3,(#49979,#49980,#49981,#49982,#49983,
#49984,#49985,#49986,#49987,#49988,#49989,#49990,#49991,#49992,#49993,#49994,
#49995,#49996,#49997,#49998,#49999,#50000,#50001,#50002,#50003,#50004,#50005,
#50006,#50007,#50008,#50009,#50010,#50011,#50012,#50013,#50014,#50015),
 .UNSPECIFIED.,.F.,.F.,(4,3,3,3,3,3,3,3,3,3,3,3,4),(0.163561610997277,0.16915058569,
0.199330059882,0.239135552965268,0.288418810440543,0.296334742315,0.337325345442903,
0.387217551940764,0.393295704107,0.436743632052119,0.473947536009189,0.486796678315,
0.489824805999),.UNSPECIFIED.);
#1362=B_SPLINE_CURVE_WITH_KNOTS('',3,(#50016,#50017,#50018,#50019),
 .UNSPECIFIED.,.F.,.F.,(4,4),(1.51692742518,1.55218902186356),
 .UNSPECIFIED.);
#1363=B_SPLINE_CURVE_WITH_KNOTS('',3,(#50026,#50027,#50028,#50029,#50030,
#50031,#50032,#50033,#50034,#50035,#50036,#50037,#50038,#50039,#50040,#50041,
#50042,#50043,#50044,#50045,#50046,#50047,#50048,#50049,#50050,#50051,#50052,
#50053,#50054,#50055,#50056,#50057,#50058,#50059,#50060,#50061,#50062,#50063,
#50064,#50065),.UNSPECIFIED.,.F.,.F.,(4,3,3,3,3,3,3,3,3,3,3,3,3,4),(0.,
0.0857703502139699,0.202245136770962,0.249999999999987,0.374999999999982,
0.422227909912381,0.468749804048871,0.499999999999978,0.574024073550536,
0.678093006562412,0.80341871283679,0.901709356418395,0.986122227259525,
1.),.UNSPECIFIED.);
#1364=B_SPLINE_CURVE_WITH_KNOTS('',3,(#50087,#50088,#50089,#50090,#50091,
#50092,#50093,#50094,#50095,#50096,#50097,#50098,#50099,#50100,#50101,#50102,
#50103,#50104,#50105,#50106,#50107,#50108,#50109,#50110,#50111,#50112,#50113,
#50114,#50115,#50116,#50117),.UNSPECIFIED.,.F.,.F.,(4,3,3,3,3,3,3,3,3,3,
4),(0.,0.11725177973149,0.25,0.345012070684631,0.440412902381579,0.5,0.640595034330486,
0.770463094223691,0.885231547111846,0.984266783604693,1.),.UNSPECIFIED.);
#1365=B_SPLINE_CURVE_WITH_KNOTS('',3,(#50122,#50123,#50124,#50125),
 .UNSPECIFIED.,.F.,.F.,(4,4),(1.51692742518,1.55218902180838),
 .UNSPECIFIED.);
#1366=B_SPLINE_CURVE_WITH_KNOTS('',3,(#50127,#50128,#50129,#50130,#50131,
#50132,#50133,#50134,#50135,#50136,#50137,#50138,#50139,#50140,#50141,#50142,
#50143,#50144,#50145,#50146,#50147,#50148,#50149,#50150,#50151,#50152,#50153,
#50154,#50155,#50156,#50157,#50158,#50159,#50160,#50161,#50162,#50163),
 .UNSPECIFIED.,.F.,.F.,(4,3,3,3,3,3,3,3,3,3,3,3,4),(0.163561610982573,0.16915058569,
0.199330059882,0.239135552965207,0.288418810441504,0.296334742315,0.337325345442626,
0.387217551940201,0.393295704107,0.436743632052091,0.473947536009078,0.486796678315,
0.489824805999),.UNSPECIFIED.);
#1367=B_SPLINE_CURVE_WITH_KNOTS('',3,(#50186,#50187,#50188,#50189,#50190,
#50191,#50192,#50193,#50194,#50195),.UNSPECIFIED.,.F.,.F.,(4,3,3,4),(-0.00626621565194798,
0.,0.0062935857631533,0.0188656317516384),.UNSPECIFIED.);
#1368=B_SPLINE_CURVE_WITH_KNOTS('',3,(#50196,#50197,#50198,#50199,#50200,
#50201,#50202,#50203,#50204,#50205,#50206,#50207,#50208,#50209,#50210,#50211,
#50212,#50213,#50214,#50215,#50216,#50217,#50218,#50219,#50220,#50221,#50222,
#50223,#50224,#50225,#50226,#50227,#50228,#50229,#50230,#50231,#50232,#50233,
#50234,#50235,#50236,#50237,#50238,#50239,#50240,#50241,#50242,#50243,#50244,
#50245,#50246,#50247,#50248,#50249,#50250,#50251,#50252,#50253,#50254,#50255,
#50256,#50257,#50258,#50259,#50260,#50261,#50262,#50263,#50264,#50265,#50266,
#50267,#50268,#50269,#50270,#50271,#50272,#50273,#50274,#50275,#50276,#50277,
#50278,#50279,#50280),.UNSPECIFIED.,.F.,.F.,(4,3,3,3,3,3,3,3,3,3,3,3,3,
3,3,3,3,3,3,3,3,3,3,3,3,3,3,3,4),(0.,0.0261765866933127,0.0558812683481721,
0.0885809143277048,0.125000000000002,0.183303332963854,0.187500000000003,
0.218750000000004,0.234375000000004,0.242187500000004,0.248195335397347,
0.250000000000004,0.256143136739208,0.313732104674438,0.375000000000005,
0.459378985198149,0.468750000000005,0.484375000000005,0.500000000000005,
0.564457131029769,0.625000000000004,0.709768961389738,0.734375000000003,
0.744291071006186,0.750000000000003,0.840934014400701,0.920467007200351,
0.992154975959462,1.),.UNSPECIFIED.);
#1369=B_SPLINE_CURVE_WITH_KNOTS('',3,(#50296,#50297,#50298,#50299,#50300,
#50301,#50302,#50303,#50304,#50305,#50306,#50307,#50308,#50309,#50310,#50311),
 .UNSPECIFIED.,.F.,.F.,(4,3,3,3,3,4),(0.338318706280354,0.44283558131635,
0.499233337792,0.619722435757,0.63299665782586,0.636935495757),
 .UNSPECIFIED.);
#1370=B_SPLINE_CURVE_WITH_KNOTS('',3,(#50312,#50313,#50314,#50315,#50316,
#50317,#50318,#50319,#50320,#50321,#50322,#50323,#50324,#50325,#50326,#50327,
#50328,#50329,#50330,#50331,#50332,#50333,#50334,#50335,#50336,#50337,#50338,
#50339),.UNSPECIFIED.,.F.,.F.,(4,3,3,3,3,3,3,3,3,4),(-0.449080636148,-0.386865408847633,
-0.32202519704816,-0.251338921067123,-0.174920549071681,-0.0882035124172373,
0.0321179319856406,0.117442754022834,0.190820231321014,0.223602276698669),
 .UNSPECIFIED.);
#1371=B_SPLINE_CURVE_WITH_KNOTS('',3,(#50375,#50376,#50377,#50378,#50379,
#50380,#50381,#50382,#50383,#50384,#50385,#50386,#50387,#50388,#50389,#50390,
#50391,#50392,#50393,#50394,#50395,#50396,#50397,#50398,#50399,#50400,#50401,
#50402),.UNSPECIFIED.,.F.,.F.,(4,3,3,3,3,3,3,3,3,4),(0.734432475987,0.878942275291463,
1.02006954288573,1.13913894251985,1.16119681048,1.21800796315046,1.27362568942023,
1.32243285508689,1.32924341569,1.33983380059),.UNSPECIFIED.);
#1372=B_SPLINE_CURVE_WITH_KNOTS('',3,(#50404,#50405,#50406,#50407,#50408,
#50409,#50410,#50411,#50412,#50413,#50414,#50415,#50416,#50417,#50418,#50419,
#50420,#50421,#50422,#50423,#50424,#50425,#50426,#50427,#50428,#50429,#50430,
#50431,#50432,#50433,#50434,#50435,#50436,#50437,#50438,#50439,#50440,#50441,
#50442,#50443,#50444,#50445,#50446,#50447,#50448,#50449,#50450,#50451,#50452,
#50453,#50454,#50455,#50456,#50457,#50458,#50459,#50460,#50461,#50462,#50463,
#50464,#50465,#50466,#50467,#50468,#50469,#50470,#50471,#50472,#50473,#50474,
#50475,#50476,#50477,#50478,#50479,#50480,#50481,#50482,#50483,#50484,#50485,
#50486,#50487,#50488,#50489,#50490,#50491,#50492,#50493,#50494,#50495,#50496,
#50497,#50498,#50499,#50500,#50501,#50502,#50503,#50504,#50505,#50506,#50507,
#50508,#50509,#50510,#50511,#50512,#50513,#50514,#50515,#50516,#50517,#50518,
#50519,#50520,#50521,#50522,#50523,#50524,#50525,#50526,#50527,#50528,#50529,
#50530,#50531,#50532,#50533,#50534,#50535,#50536,#50537,#50538,#50539,#50540,
#50541,#50542,#50543,#50544,#50545,#50546,#50547,#50548),.UNSPECIFIED.,
 .F.,.F.,(4,3,3,3,3,3,3,3,3,3,3,3,3,3,3,3,3,3,3,3,3,3,3,3,3,3,3,3,3,3,3,
3,3,3,3,3,3,3,3,3,3,3,3,3,3,3,3,3,4),(0.,0.0231346004295628,0.0500178550406402,
0.0845397778945774,0.119463675079143,0.125000000000173,0.165311219448787,
0.185320585969123,0.187500000000259,0.218750000000302,0.234375000000321,
0.242187500000328,0.247147468670735,0.250000000000335,0.286201553004801,
0.312500000000395,0.343750000000423,0.357088132051338,0.370908028354747,
0.375000000000451,0.411074730266149,0.437500000000507,0.465051541454789,
0.468750000000537,0.479325552184636,0.484375000000548,0.492187500000553,
0.496093750000553,0.498918789229101,0.500000000000554,0.536570602248778,
0.57402753795025,0.613446187852256,0.625000000000409,0.661047947208312,
0.687500000000338,0.717129701733469,0.718750000000303,0.734375000000285,
0.742187500000277,0.747463775729895,0.750000000000268,0.788333005300937,
0.827104022079326,0.867124780858469,0.875000000000134,0.915207770758867,
0.958291812587217,1.),.UNSPECIFIED.);
#1373=B_SPLINE_CURVE_WITH_KNOTS('',5,(#50549,#50550,#50551,#50552,#50553,
#50554),.UNSPECIFIED.,.F.,.F.,(6,6),(1.26425849888,1.32115953697),
 .UNSPECIFIED.);
#1374=B_SPLINE_CURVE_WITH_KNOTS('',5,(#50570,#50571,#50572,#50573,#50574,
#50575,#50576,#50577,#50578),.UNSPECIFIED.,.F.,.F.,(6,3,6),(-2.46410111513,
-2.39098596142,-2.37851323355),.UNSPECIFIED.);
#1375=B_SPLINE_CURVE_WITH_KNOTS('',5,(#50579,#50580,#50581,#50582,#50583,
#50584,#50585,#50586,#50587,#50588,#50589,#50590,#50591,#50592,#50593,#50594,
#50595,#50596,#50597,#50598,#50599),.UNSPECIFIED.,.F.,.F.,(6,3,3,3,3,3,
6),(-2.96825275179,-2.92587181617,-2.2858594369,-1.59285457075,-0.896955996606,
-0.723663994252,-0.586327318555),.UNSPECIFIED.);
#1376=B_SPLINE_CURVE_WITH_KNOTS('',3,(#50641,#50642,#50643,#50644,#50645,
#50646,#50647,#50648,#50649,#50650,#50651,#50652,#50653,#50654,#50655,#50656,
#50657,#50658,#50659,#50660,#50661,#50662,#50663,#50664,#50665,#50666,#50667,
#50668,#50669,#50670,#50671,#50672,#50673,#50674,#50675,#50676,#50677,#50678,
#50679,#50680,#50681,#50682,#50683,#50684,#50685,#50686,#50687,#50688,#50689,
#50690,#50691,#50692,#50693,#50694,#50695,#50696,#50697,#50698,#50699,#50700,
#50701,#50702,#50703,#50704,#50705,#50706,#50707,#50708,#50709,#50710,#50711,
#50712,#50713,#50714,#50715,#50716,#50717,#50718,#50719,#50720,#50721,#50722,
#50723,#50724,#50725,#50726,#50727,#50728,#50729,#50730,#50731,#50732,#50733,
#50734,#50735,#50736,#50737,#50738,#50739,#50740,#50741,#50742,#50743,#50744,
#50745,#50746,#50747,#50748,#50749,#50750,#50751,#50752,#50753,#50754,#50755,
#50756,#50757,#50758,#50759,#50760,#50761,#50762,#50763,#50764,#50765,#50766,
#50767,#50768,#50769,#50770,#50771,#50772,#50773,#50774,#50775,#50776,#50777,
#50778,#50779,#50780,#50781,#50782),.UNSPECIFIED.,.F.,.F.,(4,3,3,3,3,3,
3,3,3,3,3,3,3,3,3,3,3,3,3,3,3,3,3,3,3,3,3,3,3,3,3,3,3,3,3,3,3,3,3,3,3,3,
3,3,3,3,3,4),(0.,0.0482800745763561,0.0999928168250673,0.124999999999995,
0.174135612129771,0.229896375932678,0.249999999999991,0.316269512578206,
0.374999999999986,0.422793611779239,0.428296583176361,0.478606275337593,
0.492187499999981,0.497939634911579,0.499999999999981,0.534178550728474,
0.569174422590688,0.606755351723731,0.624999999999974,0.668818159693521,
0.687499999999971,0.690040383775526,0.718749999999969,0.734374999999968,
0.742187499999968,0.746337890624969,0.748348236083954,0.748842969536751,
0.74896984420037,0.749080959617201,0.749572830868696,0.749817805808406,
0.749921584695242,0.749993974242736,0.750061734871237,0.783289856320991,
0.81080130211654,0.842900651058264,0.858950325529126,0.866975162764558,
0.870987581382273,0.872993790691131,0.873164733602404,0.874999999999989,
0.909721106998409,0.943020259505496,0.975183165959494,1.),.UNSPECIFIED.);
#1377=B_SPLINE_CURVE_WITH_KNOTS('',3,(#50785,#50786,#50787,#50788,#50789,
#50790,#50791,#50792,#50793,#50794,#50795,#50796,#50797,#50798,#50799,#50800,
#50801,#50802,#50803,#50804,#50805,#50806,#50807,#50808,#50809,#50810,#50811,
#50812,#50813,#50814,#50815,#50816,#50817,#50818,#50819,#50820,#50821,#50822,
#50823,#50824,#50825,#50826,#50827,#50828,#50829,#50830,#50831,#50832,#50833,
#50834,#50835,#50836,#50837,#50838,#50839,#50840,#50841,#50842,#50843,#50844,
#50845,#50846,#50847,#50848,#50849,#50850,#50851,#50852,#50853,#50854,#50855,
#50856,#50857,#50858,#50859,#50860,#50861,#50862,#50863,#50864,#50865,#50866,
#50867,#50868,#50869,#50870,#50871,#50872),.UNSPECIFIED.,.F.,.F.,(4,3,3,
3,3,3,3,3,3,3,3,3,3,3,3,3,3,3,3,3,3,3,3,3,3,3,3,3,3,4),(0.,0.0677279874926389,
0.125000000000004,0.187500000000006,0.234375000000007,0.238769531250007,
0.240898132324226,0.241827442804597,0.242623468185741,0.246760234804936,
0.24876398113611,0.249960312481452,0.250461958420372,0.319628467835613,
0.37500000000001,0.43750000000001,0.468750000000011,0.484375000000011,0.492187500000011,
0.496093750000011,0.500000000000011,0.581594064625126,0.590609029780262,
0.664723012700118,0.735690189997278,0.750000000000005,0.823627905476949,
0.911813952738474,0.970263966690367,1.),.UNSPECIFIED.);
#1378=B_SPLINE_CURVE_WITH_KNOTS('',3,(#50879,#50880,#50881,#50882,#50883,
#50884,#50885,#50886,#50887,#50888,#50889,#50890,#50891,#50892,#50893,#50894,
#50895,#50896,#50897,#50898,#50899,#50900,#50901,#50902,#50903,#50904,#50905,
#50906,#50907,#50908,#50909,#50910,#50911,#50912,#50913,#50914,#50915,#50916,
#50917,#50918),.UNSPECIFIED.,.F.,.F.,(4,3,3,3,3,3,3,3,3,3,3,3,3,4),(0.342430056326,
0.416647889440572,0.493342454420148,0.569706842465,0.648977821089767,0.726755174830412,
0.787545489389,0.864698238944471,0.942373129697395,1.0113837312,1.09481342684991,
1.13043704811,1.14340426682165,1.14838178471),.UNSPECIFIED.);
#1379=B_SPLINE_CURVE_WITH_KNOTS('',3,(#51267,#51268,#51269,#51270,#51271,
#51272,#51273,#51274,#51275,#51276),.UNSPECIFIED.,.F.,.F.,(4,2,2,2,4),(0.,
0.0166816603056456,0.0333322760364835,0.0499757597117433,0.0666639750956066),
 .UNSPECIFIED.);
#1380=B_SPLINE_CURVE_WITH_KNOTS('',3,(#51279,#51280,#51281,#51282,#51283,
#51284,#51285,#51286,#51287,#51288,#51289,#51290,#51291,#51292,#51293,#51294,
#51295,#51296,#51297,#51298,#51299,#51300,#51301,#51302,#51303,#51304,#51305,
#51306,#51307,#51308,#51309,#51310,#51311,#51312,#51313,#51314,#51315,#51316,
#51317,#51318,#51319,#51320,#51321,#51322,#51323,#51324,#51325,#51326,#51327),
 .UNSPECIFIED.,.F.,.F.,(4,3,3,3,3,3,3,3,3,3,3,3,3,3,3,3,4),(0.342430099983039,
0.406155276626072,0.471478495422541,0.538329105188344,0.569706842465,0.635135726209432,
0.678900017195,0.741518988230734,0.787545489389,0.852180995271464,0.919332213618591,
0.987762598983568,1.0113837312,1.07392703039314,1.13043704811,1.14591870241,
1.14838178471),.UNSPECIFIED.);
#1381=B_SPLINE_CURVE_WITH_KNOTS('',3,(#51349,#51350,#51351,#51352,#51353,
#51354),.UNSPECIFIED.,.F.,.F.,(4,2,4),(-0.025439056349247,-0.0127192586494339,
0.),.UNSPECIFIED.);
#1382=B_SPLINE_CURVE_WITH_KNOTS('',5,(#51358,#51359,#51360,#51361,#51362,
#51363,#51364,#51365,#51366),.UNSPECIFIED.,.F.,.F.,(6,3,6),(0.995280026640254,
1.21544696444,1.22129342209),.UNSPECIFIED.);
#1383=B_SPLINE_CURVE_WITH_KNOTS('',3,(#51393,#51394,#51395,#51396,#51397,
#51398,#51399,#51400,#51401,#51402,#51403,#51404,#51405,#51406,#51407,#51408,
#51409,#51410,#51411,#51412,#51413,#51414,#51415,#51416,#51417,#51418,#51419,
#51420,#51421,#51422,#51423,#51424,#51425,#51426,#51427,#51428,#51429,#51430,
#51431,#51432,#51433,#51434,#51435,#51436,#51437,#51438,#51439,#51440,#51441,
#51442,#51443,#51444,#51445,#51446,#51447,#51448,#51449,#51450,#51451,#51452,
#51453,#51454,#51455,#51456),.UNSPECIFIED.,.F.,.F.,(4,3,3,3,3,3,3,3,3,3,
3,3,3,3,3,3,3,3,3,3,3,4),(0.,0.948237676895928,2.04200576184201,3.37474848426459,
4.40850535538508,5.30596315772473,5.58045964467773,6.71900177794048,8.10021196688407,
9.27267325358068,10.1040285365416,10.4451345402773,10.8737182939327,11.3495434571161,
11.699840638544,11.8670612467535,12.5378975955484,13.1340007751306,13.642280142205,
14.1090493942805,14.5397893196166,14.6803195994),.UNSPECIFIED.);
#1384=B_SPLINE_CURVE_WITH_KNOTS('',5,(#51459,#51460,#51461,#51462,#51463,
#51464,#51465,#51466,#51467,#51468,#51469,#51470),.UNSPECIFIED.,.F.,.F.,
(6,3,3,6),(6.85951996631323E-8,0.420938628926706,0.701481831484658,0.999999989476295),
 .UNSPECIFIED.);
#1385=B_SPLINE_CURVE_WITH_KNOTS('',3,(#51483,#51484,#51485,#51486,#51487,
#51488),.UNSPECIFIED.,.F.,.F.,(4,2,4),(-0.0251203830680402,-0.0125600919312397,
0.),.UNSPECIFIED.);
#1386=B_SPLINE_CURVE_WITH_KNOTS('',3,(#51489,#51490,#51491,#51492,#51493,
#51494,#51495,#51496,#51497,#51498,#51499,#51500,#51501,#51502,#51503,#51504,
#51505,#51506,#51507,#51508,#51509,#51510,#51511,#51512,#51513),
 .UNSPECIFIED.,.F.,.F.,(4,3,3,3,3,3,3,3,4),(1.01054286647469,1.0614593193646,
1.11979310493141,1.18952357816526,1.23011259501,1.26531612164489,1.29489655211715,
1.31773496162,1.32384910338),.UNSPECIFIED.);
#1387=B_SPLINE_CURVE_WITH_KNOTS('',3,(#51533,#51534,#51535,#51536,#51537,
#51538,#51539,#51540,#51541,#51542,#51543,#51544,#51545,#51546,#51547,#51548,
#51549,#51550,#51551,#51552,#51553,#51554,#51555,#51556,#51557,#51558,#51559,
#51560,#51561,#51562,#51563,#51564,#51565,#51566,#51567,#51568,#51569),
 .UNSPECIFIED.,.F.,.F.,(4,3,3,3,3,3,3,3,3,3,3,3,4),(0.163561586048556,0.16915058569,
0.199330059882,0.239717424431074,0.289567767371195,0.296334742315,0.342221563674437,
0.389994474503767,0.393295704107,0.435638979152134,0.473912817661004,0.486796678315,
0.489824805999),.UNSPECIFIED.);
#1388=B_SPLINE_CURVE_WITH_KNOTS('',3,(#51598,#51599,#51600,#51601,#51602,
#51603,#51604,#51605,#51606,#51607,#51608,#51609,#51610,#51611,#51612,#51613,
#51614,#51615,#51616,#51617,#51618,#51619,#51620,#51621,#51622,#51623,#51624,
#51625,#51626,#51627,#51628,#51629,#51630,#51631,#51632,#51633,#51634,#51635,
#51636,#51637,#51638,#51639,#51640,#51641,#51642,#51643,#51644,#51645,#51646,
#51647,#51648,#51649,#51650,#51651,#51652,#51653,#51654,#51655,#51656,#51657,
#51658,#51659,#51660,#51661,#51662,#51663,#51664),.UNSPECIFIED.,.F.,.F.,
(4,3,3,3,3,3,3,3,3,3,3,3,3,3,3,3,3,3,3,3,3,3,4),(0.,0.150485130188399,0.30297850459967,
0.457031628712122,0.561567306255,0.709215379177615,0.854264253416426,0.913473553147556,
1.04884917352124,1.12559454297,1.28001930589065,1.43693558960681,1.58742667059295,
1.69044089606,1.82557173927566,1.8394563651115,1.98772408517656,2.13847260473739,
2.25475688458,2.40866618427487,2.56165891031834,2.71215471728285,2.77932659819),
 .UNSPECIFIED.);
#1389=B_SPLINE_CURVE_WITH_KNOTS('',5,(#51667,#51668,#51669,#51670,#51671,
#51672,#51673,#51674,#51675,#51676,#51677,#51678),.UNSPECIFIED.,.F.,.F.,
(6,3,3,6),(0.,0.204469498724444,0.476563204173844,1.),.UNSPECIFIED.);
#1390=B_SPLINE_CURVE_WITH_KNOTS('',3,(#51695,#51696,#51697,#51698,#51699,
#51700,#51701,#51702,#51703,#51704,#51705,#51706,#51707,#51708,#51709,#51710,
#51711,#51712,#51713,#51714,#51715,#51716),.UNSPECIFIED.,.F.,.F.,(4,3,3,
3,3,3,3,4),(0.734432475987,0.897425480061445,1.04019709468454,1.16119681048,
1.22610423484268,1.28628740602881,1.32924341569,1.33983379849382),
 .UNSPECIFIED.);
#1391=B_SPLINE_CURVE_WITH_KNOTS('',3,(#51729,#51730,#51731,#51732,#51733,
#51734,#51735,#51736,#51737,#51738,#51739,#51740,#51741,#51742,#51743,#51744,
#51745,#51746,#51747,#51748,#51749,#51750,#51751,#51752,#51753,#51754,#51755,
#51756,#51757,#51758,#51759),.UNSPECIFIED.,.F.,.F.,(4,3,3,3,3,3,3,3,3,3,
4),(0.,0.244795327918773,0.502847705033991,0.780409654548682,1.09688525358557,
1.52122108872678,1.83404989561054,2.11578718796133,2.37921313711228,2.62468126213379,
2.75757599775),.UNSPECIFIED.);
#1392=B_SPLINE_CURVE_WITH_KNOTS('',3,(#51761,#51762,#51763,#51764,#51765,
#51766,#51767),.UNSPECIFIED.,.F.,.F.,(4,3,4),(0.881014033286,0.948965831295187,
0.963434555076),.UNSPECIFIED.);
#1393=B_SPLINE_CURVE_WITH_KNOTS('',3,(#51768,#51769,#51770,#51771,#51772,
#51773,#51774,#51775,#51776,#51777,#51778,#51779,#51780,#51781,#51782,#51783,
#51784,#51785,#51786,#51787,#51788,#51789,#51790,#51791,#51792,#51793,#51794,
#51795,#51796,#51797,#51798,#51799,#51800,#51801,#51802,#51803,#51804,#51805,
#51806,#51807,#51808,#51809,#51810,#51811,#51812,#51813,#51814,#51815,#51816),
 .UNSPECIFIED.,.F.,.F.,(4,3,3,3,3,3,3,3,3,3,3,3,3,3,3,3,4),(-2.96825275179,
-2.92587181617,-2.75740998902055,-2.58343808727891,-2.39896382434401,-2.2858594369,
-2.08411702426915,-1.87893514117023,-1.67994580319545,-1.59285457075,-1.39361191417081,
-1.20541337865871,-1.0344021207881,-0.896955996606,-0.740414779189322,-0.723663994252,
-0.586327318555),.UNSPECIFIED.);
#1394=B_SPLINE_CURVE_WITH_KNOTS('',3,(#51868,#51869,#51870,#51871,#51872,
#51873,#51874,#51875,#51876,#51877,#51878,#51879,#51880,#51881,#51882,#51883,
#51884,#51885,#51886,#51887,#51888,#51889,#51890,#51891,#51892,#51893,#51894,
#51895,#51896,#51897,#51898),.UNSPECIFIED.,.F.,.F.,(4,3,3,3,3,3,3,3,3,3,
4),(0.,0.106507047524963,0.214193650328982,0.326022688788743,0.446688121212756,
0.5,0.610700523139681,0.71326332802124,0.814167331458963,0.917046982929181,
1.),.UNSPECIFIED.);
#1395=B_SPLINE_CURVE_WITH_KNOTS('',3,(#51957,#51958,#51959,#51960,#51961,
#51962,#51963,#51964,#51965,#51966,#51967,#51968,#51969,#51970,#51971,#51972,
#51973,#51974,#51975,#51976,#51977,#51978,#51979,#51980,#51981,#51982,#51983,
#51984,#51985,#51986,#51987,#51988,#51989,#51990,#51991,#51992,#51993),
 .UNSPECIFIED.,.F.,.F.,(4,3,3,3,3,3,3,3,3,3,3,3,4),(0.,0.109774660407206,
0.236893273816627,0.249999999999999,0.323861363638668,0.396238624772552,
0.463887957515316,0.499999999999997,0.565010634550699,0.71662408184464,
0.842148144824872,0.956539659898614,1.),.UNSPECIFIED.);
#1396=B_SPLINE_CURVE_WITH_KNOTS('',3,(#52031,#52032,#52033,#52034,#52035,
#52036,#52037,#52038,#52039,#52040),.UNSPECIFIED.,.F.,.F.,(4,3,3,4),(1.28339894164,
1.30680607386887,1.3328892219684,1.34350433703),.UNSPECIFIED.);
#1397=B_SPLINE_CURVE_WITH_KNOTS('',3,(#52141,#52142,#52143,#52144,#52145,
#52146,#52147,#52148,#52149,#52150,#52151,#52152,#52153,#52154,#52155,#52156,
#52157,#52158,#52159,#52160,#52161,#52162,#52163,#52164,#52165,#52166,#52167,
#52168,#52169,#52170,#52171,#52172,#52173,#52174,#52175,#52176,#52177),
 .UNSPECIFIED.,.F.,.F.,(4,3,3,3,3,3,3,3,3,3,3,3,4),(5.1954086812113E-8,
0.0881831468536577,0.192584408778802,0.301488460118701,0.404564094688347,
0.5,0.561992944439645,0.652033254324342,0.748248539918247,0.841547093326746,
0.920773546663373,0.993552974112633,1.),.UNSPECIFIED.);
#1398=B_SPLINE_CURVE_WITH_KNOTS('',3,(#52291,#52292,#52293,#52294,#52295,
#52296,#52297,#52298,#52299,#52300,#52301,#52302,#52303,#52304,#52305,#52306,
#52307,#52308,#52309,#52310,#52311,#52312,#52313,#52314,#52315,#52316,#52317,
#52318,#52319,#52320,#52321,#52322,#52323,#52324,#52325,#52326,#52327,#52328,
#52329,#52330,#52331,#52332,#52333,#52334,#52335,#52336,#52337,#52338,#52339,
#52340,#52341,#52342,#52343,#52344,#52345,#52346,#52347,#52348,#52349,#52350,
#52351,#52352,#52353,#52354,#52355,#52356,#52357,#52358,#52359,#52360,#52361,
#52362,#52363,#52364,#52365,#52366,#52367,#52368,#52369,#52370,#52371,#52372,
#52373,#52374,#52375,#52376,#52377,#52378,#52379,#52380,#52381,#52382,#52383,
#52384,#52385,#52386,#52387,#52388,#52389,#52390,#52391,#52392,#52393,#52394,
#52395,#52396,#52397,#52398,#52399,#52400,#52401,#52402,#52403,#52404,#52405,
#52406,#52407,#52408,#52409,#52410,#52411,#52412,#52413,#52414,#52415,#52416,
#52417,#52418,#52419,#52420,#52421,#52422,#52423),.UNSPECIFIED.,.F.,.F.,
(4,3,3,3,3,3,3,3,3,3,3,3,3,3,3,3,3,3,3,3,3,3,3,3,3,3,3,3,3,3,3,3,3,3,3,
3,3,3,3,3,3,3,3,3,4),(0.,0.0449839752208177,0.094648655991429,0.125000000000001,
0.180289664252898,0.187500000000002,0.218750000000002,0.234375000000002,
0.242187500000002,0.246093750000002,0.250000000000003,0.307559572351956,
0.356504949280997,0.375000000000005,0.417469288796414,0.426882497257103,
0.437500000000006,0.468750000000007,0.487024846094567,0.500000000000007,
0.539444949446193,0.579065581700542,0.619687961577662,0.62500000000001,
0.667322932809044,0.687500000000011,0.696132105409999,0.718750000000011,
0.734375000000012,0.742187500000012,0.746093750000011,0.748046875000011,
0.750000000000011,0.787230005409161,0.812500000000007,0.843750000000005,
0.859375000000004,0.867187500000004,0.871093750000003,0.874404103182036,
0.875000000000003,0.910890016908024,0.944438319456343,0.97591609698468,
0.999999989299826),.UNSPECIFIED.);
#1399=B_SPLINE_CURVE_WITH_KNOTS('',3,(#52481,#52482,#52483,#52484,#52485,
#52486,#52487,#52488,#52489,#52490,#52491,#52492,#52493,#52494,#52495,#52496,
#52497,#52498,#52499,#52500,#52501,#52502,#52503,#52504,#52505),
 .UNSPECIFIED.,.F.,.F.,(4,3,3,3,3,3,3,3,4),(1.01054286443581,1.06145887153934,
1.11979195427008,1.18952209299618,1.23011254057257,1.26581096316738,1.29483003327369,
1.3210114243818,1.32384910338),.UNSPECIFIED.);
#1400=B_SPLINE_CURVE_WITH_KNOTS('',3,(#52562,#52563,#52564,#52565,#52566,
#52567,#52568,#52569,#52570,#52571,#52572,#52573,#52574,#52575,#52576,#52577,
#52578,#52579,#52580,#52581,#52582,#52583,#52584,#52585,#52586,#52587,#52588,
#52589,#52590,#52591,#52592,#52593,#52594,#52595,#52596,#52597,#52598,#52599,
#52600,#52601,#52602,#52603,#52604,#52605,#52606,#52607,#52608,#52609,#52610,
#52611,#52612,#52613,#52614,#52615,#52616,#52617,#52618,#52619,#52620,#52621,
#52622,#52623,#52624,#52625,#52626,#52627,#52628,#52629,#52630,#52631,#52632,
#52633,#52634,#52635,#52636,#52637,#52638,#52639,#52640,#52641,#52642,#52643,
#52644,#52645,#52646,#52647,#52648,#52649),.UNSPECIFIED.,.F.,.F.,(4,3,3,
3,3,3,3,3,3,3,3,3,3,3,3,3,3,3,3,3,3,3,3,3,3,3,3,3,3,4),(0.,0.0642476278262248,
0.125,0.1875,0.234375000000001,0.238769531250001,0.240898132324219,0.24178163869067,
0.242599226648374,0.246736750815612,0.248740864084118,0.249891670367119,
0.25033373353469,0.318681145396987,0.375000000000002,0.437500000000002,
0.468750000000002,0.484375000000002,0.492187500000003,0.496093750000003,
0.498046875000003,0.500000000000003,0.582577073350837,0.601597297982624,
0.677425679242019,0.750000000000001,0.824704147685727,0.912352073842863,
0.976551486277736,1.),.UNSPECIFIED.);
#1401=B_SPLINE_CURVE_WITH_KNOTS('',3,(#52686,#52687,#52688,#52689),
 .UNSPECIFIED.,.F.,.F.,(4,4),(0.995280026642634,1.22129342209),
 .UNSPECIFIED.);
#1402=B_SPLINE_CURVE_WITH_KNOTS('',3,(#52728,#52729,#52730,#52731,#52732,
#52733,#52734,#52735,#52736,#52737),.UNSPECIFIED.,.F.,.F.,(4,3,3,4),(-2.46410111513,
-2.43156045184461,-2.3842002845234,-2.37851323355),.UNSPECIFIED.);
#1403=B_SPLINE_CURVE_WITH_KNOTS('',3,(#52794,#52795,#52796,#52797,#52798,
#52799,#52800,#52801,#52802,#52803,#52804,#52805,#52806,#52807,#52808,#52809,
#52810,#52811,#52812,#52813,#52814,#52815,#52816,#52817,#52818,#52819,#52820,
#52821,#52822,#52823,#52824,#52825,#52826,#52827,#52828,#52829,#52830,#52831,
#52832,#52833,#52834,#52835,#52836,#52837,#52838,#52839,#52840,#52841,#52842,
#52843,#52844,#52845,#52846,#52847,#52848,#52849,#52850,#52851,#52852,#52853,
#52854,#52855,#52856,#52857,#52858,#52859,#52860,#52861,#52862,#52863,#52864,
#52865,#52866,#52867,#52868,#52869,#52870,#52871,#52872,#52873,#52874,#52875,
#52876,#52877,#52878,#52879,#52880,#52881,#52882,#52883,#52884,#52885,#52886,
#52887,#52888,#52889,#52890,#52891,#52892,#52893,#52894,#52895,#52896,#52897,
#52898,#52899,#52900,#52901,#52902,#52903,#52904,#52905),.UNSPECIFIED.,
 .F.,.F.,(4,3,3,3,3,3,3,3,3,3,3,3,3,3,3,3,3,3,3,3,3,3,3,3,3,3,3,3,3,3,3,
3,3,3,3,3,3,4),(0.,0.0477135724161135,0.0625000000000017,0.0937500000000023,
0.109375000000002,0.117187500000002,0.125000000000003,0.181640986341184,
0.187500000000002,0.218750000000002,0.234375000000003,0.248990132814251,
0.250000000000003,0.329265328614751,0.375000000000004,0.46359821529961,
0.479221960529419,0.483322124721982,0.48530594038562,0.498216219979678,
0.499936854854124,0.500928588655433,0.566229497664171,0.588588177138087,
0.624999999999997,0.684372375983187,0.687499999999994,0.718749999999992,
0.734374999999992,0.742187499999992,0.749136996345081,0.749999999999992,
0.796469608533299,0.844400751682625,0.891704275157033,0.93900736088884,
0.987732013854371,1.),.UNSPECIFIED.);
#1404=B_SPLINE_CURVE_WITH_KNOTS('',3,(#52944,#52945,#52946,#52947,#52948,
#52949,#52950),.UNSPECIFIED.,.F.,.F.,(4,3,4),(0.881014033286,0.948706774547412,
0.963434555076),.UNSPECIFIED.);
#1405=B_SPLINE_CURVE_WITH_KNOTS('',3,(#53007,#53008,#53009,#53010,#53011,
#53012,#53013,#53014,#53015,#53016,#53017,#53018,#53019,#53020,#53021,#53022,
#53023,#53024,#53025),.UNSPECIFIED.,.F.,.F.,(4,3,3,3,3,3,4),(0.,0.324828279928709,
0.585140352773158,0.649656559857417,0.772280636003616,0.895427880757141,
0.999999948942922),.UNSPECIFIED.);
#1406=B_SPLINE_CURVE_WITH_KNOTS('',3,(#53100,#53101,#53102,#53103,#53104,
#53105,#53106,#53107,#53108,#53109,#53110,#53111,#53112,#53113,#53114,#53115,
#53116,#53117,#53118,#53119,#53120,#53121,#53122,#53123,#53124,#53125,#53126,
#53127,#53128,#53129,#53130,#53131,#53132,#53133,#53134,#53135,#53136,#53137,
#53138,#53139,#53140,#53141,#53142,#53143,#53144,#53145,#53146,#53147,#53148,
#53149,#53150,#53151,#53152,#53153,#53154,#53155,#53156,#53157,#53158,#53159,
#53160,#53161,#53162,#53163,#53164,#53165,#53166,#53167,#53168,#53169,#53170,
#53171,#53172,#53173,#53174,#53175,#53176,#53177,#53178,#53179,#53180,#53181,
#53182,#53183,#53184,#53185,#53186,#53187,#53188,#53189,#53190,#53191,#53192,
#53193,#53194,#53195,#53196,#53197,#53198,#53199),.UNSPECIFIED.,.F.,.F.,
(4,3,3,3,3,3,3,3,3,3,3,3,3,3,3,3,3,3,3,3,3,3,3,3,3,3,3,3,3,3,3,3,3,4),(2.31347827906944E-9,
0.0304523904386003,0.0667565854045198,0.111071614656439,0.125000000000009,
0.166228903356154,0.196195787703402,0.218750000000012,0.23437500000001,
0.242763564282923,0.250000000000009,0.286657323311203,0.322698560618276,
0.357210368699332,0.375000000000006,0.406250000000004,0.437500000000003,
0.465316625673246,0.468750000000002,0.478007170175177,0.490299230010994,
0.500000000000001,0.533658524008943,0.56889649930393,0.606784435493325,
0.625000000000001,0.667117677043821,0.713500024564271,0.750000000000001,
0.806522802216992,0.865633153944195,0.9249705316322,0.984382807636567,1.),
 .UNSPECIFIED.);
#1407=B_SPLINE_CURVE_WITH_KNOTS('',3,(#53238,#53239,#53240,#53241),
 .UNSPECIFIED.,.F.,.F.,(4,4),(1.26426572301,1.32115953697),
 .UNSPECIFIED.);
#1408=B_SPLINE_CURVE_WITH_KNOTS('',3,(#53254,#53255,#53256,#53257,#53258,
#53259,#53260,#53261,#53262,#53263,#53264,#53265,#53266,#53267,#53268,#53269,
#53270,#53271,#53272,#53273,#53274,#53275),.UNSPECIFIED.,.F.,.F.,(4,3,3,
3,3,3,3,4),(0.338318706236,0.438258273139173,0.499233337792,0.545290114175537,
0.592030438707663,0.619722435757,0.633910105997971,0.636934808527437),
 .UNSPECIFIED.);
#1409=B_SPLINE_CURVE_WITH_KNOTS('',3,(#53279,#53280,#53281,#53282,#53283,
#53284),.UNSPECIFIED.,.F.,.F.,(4,2,4),(-0.10130067680855,-0.0506503369484061,
0.),.UNSPECIFIED.);
#1410=B_SPLINE_CURVE_WITH_KNOTS('',3,(#53329,#53330,#53331,#53332,#53333,
#53334,#53335,#53336,#53337,#53338,#53339,#53340,#53341,#53342,#53343,#53344,
#53345,#53346,#53347,#53348,#53349,#53350,#53351,#53352,#53353,#53354,#53355,
#53356,#53357,#53358,#53359,#53360,#53361,#53362,#53363,#53364,#53365,#53366,
#53367,#53368,#53369,#53370,#53371,#53372,#53373,#53374,#53375,#53376,#53377,
#53378,#53379,#53380,#53381,#53382,#53383,#53384,#53385,#53386,#53387,#53388,
#53389,#53390,#53391,#53392,#53393,#53394,#53395,#53396,#53397,#53398,#53399,
#53400,#53401,#53402,#53403,#53404,#53405,#53406,#53407,#53408,#53409,#53410,
#53411,#53412,#53413,#53414,#53415,#53416,#53417,#53418,#53419,#53420,#53421,
#53422,#53423,#53424,#53425,#53426,#53427,#53428,#53429,#53430,#53431,#53432,
#53433,#53434,#53435,#53436,#53437,#53438,#53439,#53440,#53441,#53442,#53443,
#53444,#53445,#53446,#53447,#53448,#53449,#53450,#53451,#53452,#53453,#53454,
#53455),.UNSPECIFIED.,.F.,.F.,(4,3,3,3,3,3,3,3,3,3,3,3,3,3,3,3,3,3,3,3,
3,3,3,3,3,3,3,3,3,3,3,3,3,3,3,3,3,3,3,3,3,3,4),(0.,0.0327143155580901,0.0625000000000028,
0.0937500000000044,0.109578455637257,0.125000000000006,0.163523013959447,
0.18750000000001,0.218750000000012,0.234375000000013,0.242187500000013,
0.246093750000014,0.249607117920692,0.250000000000014,0.257249878340838,
0.310510045979528,0.365381093929824,0.375000000000014,0.437500000000014,
0.468750000000014,0.484375000000014,0.489260595055283,0.491884315109107,
0.492587087124586,0.496959426734569,0.499008960926749,0.499641842136478,
0.500058671728224,0.552911785914761,0.56254452088432,0.615548813869578,
0.676384667730263,0.687500000000005,0.718750000000004,0.734375000000003,
0.742187500000003,0.74809367806907,0.750000000000003,0.809173214063901,
0.86756885888069,0.925738391101094,0.984348401097454,1.),.UNSPECIFIED.);
#1411=B_SPLINE_CURVE_WITH_KNOTS('',3,(#53460,#53461,#53462,#53463,#53464,
#53465),.UNSPECIFIED.,.F.,.F.,(4,2,4),(-0.750622279262213,-0.375340681565196,
0.),.UNSPECIFIED.);
#1412=B_SPLINE_CURVE_WITH_KNOTS('',3,(#53632,#53633,#53634,#53635,#53636,
#53637,#53638,#53639,#53640,#53641,#53642,#53643,#53644,#53645,#53646,#53647,
#53648,#53649,#53650),.UNSPECIFIED.,.F.,.F.,(4,3,3,3,3,3,4),(0.,0.158500319086325,
0.31863860447099,0.487780059128932,0.719403646007813,0.865891955512973,
0.999999739264845),.UNSPECIFIED.);
#1413=B_SPLINE_CURVE_WITH_KNOTS('',3,(#53727,#53728,#53729,#53730,#53731,
#53732,#53733,#53734,#53735,#53736),.UNSPECIFIED.,.F.,.F.,(4,3,3,4),(1.28339894164,
1.30680607386887,1.3328892219684,1.34350433703),.UNSPECIFIED.);
#1414=B_SPLINE_CURVE_WITH_KNOTS('',5,(#53792,#53793,#53794,#53795,#53796,
#53797,#53798,#53799,#53800),.UNSPECIFIED.,.F.,.F.,(6,3,6),(0.,0.571293900064368,
1.),.UNSPECIFIED.);
#1415=B_SPLINE_CURVE_WITH_KNOTS('',5,(#53840,#53841,#53842,#53843,#53844,
#53845),.UNSPECIFIED.,.F.,.F.,(6,6),(0.,1.),.UNSPECIFIED.);
#1416=B_SPLINE_CURVE_WITH_KNOTS('',5,(#54050,#54051,#54052,#54053,#54054,
#54055,#54056,#54057,#54058,#54059,#54060,#54061),.UNSPECIFIED.,.F.,.F.,
(6,3,3,6),(1.3907936820211E-8,0.256132634704352,0.563769826408177,1.),
 .UNSPECIFIED.);
#1417=B_SPLINE_CURVE_WITH_KNOTS('',3,(#54082,#54083,#54084,#54085,#54086,
#54087),.UNSPECIFIED.,.F.,.F.,(4,2,4),(-0.750622269444262,-0.375342208613163,
0.),.UNSPECIFIED.);
#1418=B_SPLINE_CURVE_WITH_KNOTS('',3,(#54100,#54101,#54102,#54103,#54104,
#54105),.UNSPECIFIED.,.F.,.F.,(4,2,4),(-0.101300676824578,-0.0506503372063276,
0.),.UNSPECIFIED.);
#1419=B_SPLINE_CURVE_WITH_KNOTS('',3,(#54107,#54108,#54109,#54110,#54111,
#54112,#54113,#54114,#54115,#54116,#54117,#54118,#54119,#54120,#54121,#54122,
#54123,#54124,#54125,#54126,#54127,#54128),.UNSPECIFIED.,.F.,.F.,(4,3,3,
3,3,3,3,4),(0.338318706236,0.438258273139173,0.499233337792,0.545290114175537,
0.592030438707663,0.619722435757,0.633910105997956,0.636934808527438),
 .UNSPECIFIED.);
#1420=B_SPLINE_CURVE_WITH_KNOTS('',5,(#54129,#54130,#54131,#54132,#54133,
#54134),.UNSPECIFIED.,.F.,.F.,(6,6),(1.26425849888,1.32115953697),
 .UNSPECIFIED.);
#1421=B_SPLINE_CURVE_WITH_KNOTS('',3,(#55086,#55087,#55088,#55089,#55090,
#55091,#55092,#55093,#55094,#55095,#55096,#55097,#55098,#55099,#55100,#55101,
#55102,#55103,#55104,#55105,#55106,#55107),.UNSPECIFIED.,.F.,.F.,(4,3,3,
3,3,3,3,4),(0.,0.528382896990167,1.08470689628943,1.66556978220358,2.28030783605745,
2.98182977652019,3.78815962830722,4.53770086709),.UNSPECIFIED.);
#1422=B_SPLINE_CURVE_WITH_KNOTS('',3,(#55123,#55124,#55125,#55126,#55127,
#55128,#55129,#55130,#55131,#55132),.UNSPECIFIED.,.F.,.F.,(4,2,2,2,4),(0.,
0.0110292280070327,0.0220815628933708,0.0331350655826502,0.0441631624440209),
 .UNSPECIFIED.);
#1423=B_SPLINE_CURVE_WITH_KNOTS('',3,(#55152,#55153,#55154,#55155,#55156,
#55157),.UNSPECIFIED.,.F.,.F.,(4,2,4),(-0.0254390562091683,-0.0127192554937957,
0.),.UNSPECIFIED.);
#1424=B_SPLINE_CURVE_WITH_KNOTS('',3,(#55171,#55172,#55173,#55174,#55175,
#55176,#55177,#55178,#55179,#55180),.UNSPECIFIED.,.F.,.F.,(4,2,2,2,4),(0.,
0.0166816603056456,0.0333322760364837,0.0499757597117436,0.066663975095607),
 .UNSPECIFIED.);
#1425=B_SPLINE_CURVE_WITH_KNOTS('',3,(#55207,#55208,#55209,#55210,#55211,
#55212,#55213,#55214,#55215,#55216,#55217,#55218,#55219,#55220,#55221,#55222,
#55223,#55224,#55225,#55226,#55227,#55228,#55229,#55230,#55231,#55232,#55233,
#55234,#55235,#55236,#55237,#55238,#55239,#55240,#55241,#55242,#55243,#55244,
#55245,#55246,#55247,#55248,#55249,#55250,#55251,#55252,#55253,#55254,#55255,
#55256,#55257,#55258,#55259,#55260,#55261,#55262,#55263,#55264,#55265,#55266,
#55267,#55268,#55269,#55270),.UNSPECIFIED.,.F.,.F.,(4,3,3,3,3,3,3,3,3,3,
3,3,3,3,3,3,3,3,3,3,3,4),(0.,0.948237676895928,2.04200576184201,3.37474848426459,
4.40850535538508,5.30596315772473,5.58045964467773,6.71900177794048,8.10021196688407,
9.27267325358068,10.1040285365416,10.4451345402773,10.8737182939327,11.3495434571161,
11.699840638544,11.8670612467535,12.5378975955484,13.1340007751306,13.642280142205,
14.1090493942805,14.5397893196166,14.6803195994),.UNSPECIFIED.);
#1426=B_SPLINE_CURVE_WITH_KNOTS('',3,(#55285,#55286,#55287,#55288,#55289,
#55290),.UNSPECIFIED.,.F.,.F.,(4,2,4),(-0.0251203830131541,-0.0125600904510716,
0.),.UNSPECIFIED.);
#1427=B_SPLINE_CURVE_WITH_KNOTS('',3,(#55311,#55312,#55313,#55314,#55315,
#55316,#55317,#55318,#55319,#55320,#55321,#55322,#55323,#55324,#55325,#55326,
#55327,#55328,#55329,#55330,#55331,#55332,#55333,#55334,#55335,#55336,#55337,
#55338,#55339,#55340,#55341,#55342,#55343,#55344,#55345,#55346,#55347,#55348,
#55349,#55350),.UNSPECIFIED.,.F.,.F.,(4,3,3,3,3,3,3,3,3,3,3,3,3,4),(0.,
0.070670504624755,0.148932316631556,0.249833176006254,0.34320409673537,
0.421793259367904,0.490751031937973,0.500382422000438,0.579388004174185,
0.668243342711819,0.83412167135591,0.917060835677955,0.993028978346361,
1.),.UNSPECIFIED.);
#1428=B_SPLINE_CURVE_WITH_KNOTS('',3,(#55365,#55366,#55367,#55368,#55369,
#55370,#55371,#55372,#55373,#55374,#55375,#55376,#55377,#55378,#55379,#55380,
#55381,#55382,#55383,#55384,#55385,#55386,#55387,#55388,#55389,#55390,#55391,
#55392,#55393,#55394,#55395),.UNSPECIFIED.,.F.,.F.,(4,3,3,3,3,3,3,3,3,3,
4),(0.,0.244795327918776,0.502847705033982,0.780409654548611,1.09688525358519,
1.52122108872658,1.83404989561042,2.11578718796133,2.37921313711243,2.62468126213374,
2.75757599775),.UNSPECIFIED.);
#1429=B_SPLINE_CURVE_WITH_KNOTS('',3,(#55435,#55436,#55437,#55438,#55439,
#55440,#55441,#55442,#55443,#55444,#55445,#55446,#55447,#55448,#55449,#55450,
#55451,#55452,#55453,#55454,#55455,#55456,#55457,#55458,#55459,#55460,#55461,
#55462,#55463,#55464,#55465,#55466,#55467,#55468,#55469,#55470,#55471,#55472,
#55473,#55474,#55475,#55476,#55477,#55478,#55479,#55480,#55481,#55482,#55483,
#55484,#55485,#55486,#55487,#55488,#55489,#55490,#55491,#55492,#55493,#55494,
#55495,#55496,#55497,#55498,#55499,#55500,#55501),.UNSPECIFIED.,.F.,.F.,
(4,3,3,3,3,3,3,3,3,3,3,3,3,3,3,3,3,3,3,3,3,3,4),(0.,0.150485130188399,0.30297850459967,
0.457031628712122,0.561567306255,0.709215379177615,0.854264253416426,0.913473553147556,
1.04884917352124,1.12559454297,1.28001930589065,1.43693558960681,1.58742667059295,
1.69044089606,1.82557173927566,1.8394563651115,1.98772408517656,2.13847260473739,
2.25475688458,2.40866618427487,2.56165891031834,2.71215471728285,2.77932659819),
 .UNSPECIFIED.);
#1430=B_SPLINE_CURVE_WITH_KNOTS('',3,(#55530,#55531,#55532,#55533,#55534,
#55535,#55536,#55537,#55538,#55539,#55540,#55541,#55542,#55543,#55544,#55545,
#55546,#55547,#55548,#55549,#55550,#55551),.UNSPECIFIED.,.F.,.F.,(4,3,3,
3,3,3,3,4),(0.,0.528382896990167,1.08470689628943,1.66556978220358,2.28030783605745,
2.98182977652019,3.78815962830722,4.53770086709),.UNSPECIFIED.);
#1431=B_SPLINE_CURVE_WITH_KNOTS('',3,(#55565,#55566,#55567,#55568,#55569,
#55570,#55571,#55572,#55573,#55574),.UNSPECIFIED.,.F.,.F.,(4,2,2,2,4),(0.,
0.0110292280070327,0.0220815628933709,0.0331350655826503,0.0441631624440211),
 .UNSPECIFIED.);
#1432=B_SPLINE_CURVE_WITH_KNOTS('',3,(#55631,#55632,#55633,#55634,#55635,
#55636,#55637,#55638,#55639,#55640,#55641,#55642,#55643,#55644,#55645,#55646,
#55647,#55648,#55649,#55650,#55651,#55652,#55653,#55654,#55655,#55656,#55657,
#55658,#55659,#55660,#55661,#55662,#55663,#55664,#55665,#55666,#55667,#55668,
#55669,#55670,#55671,#55672,#55673,#55674,#55675,#55676,#55677,#55678,#55679,
#55680,#55681,#55682,#55683,#55684,#55685,#55686,#55687,#55688,#55689,#55690,
#55691,#55692,#55693,#55694,#55695,#55696,#55697,#55698,#55699,#55700,#55701,
#55702,#55703,#55704,#55705,#55706,#55707,#55708,#55709,#55710,#55711,#55712,
#55713,#55714,#55715,#55716,#55717,#55718,#55719,#55720,#55721,#55722,#55723,
#55724,#55725,#55726,#55727,#55728,#55729,#55730,#55731,#55732,#55733,#55734,
#55735,#55736),.UNSPECIFIED.,.F.,.F.,(4,3,3,3,3,3,3,3,3,3,3,3,3,3,3,3,3,
3,3,3,3,3,3,3,3,3,3,3,3,3,3,3,3,3,3,4),(0.,0.0384119876990658,0.0763318975960008,
0.113412177947531,0.124999999999992,0.160716651462973,0.187499999999989,
0.218749999999986,0.232928769092456,0.246751174516542,0.249999999999984,
0.282386237316996,0.31654907127058,0.350680938752922,0.386159172447775,
0.419037573131334,0.455347724810625,0.489388492009961,0.497366796822306,
0.497748630780966,0.497988260492532,0.498153598164076,0.499133766917662,
0.499622894098407,0.499829505667003,0.499975189523554,0.500092687390758,
0.554153889445409,0.611580585028303,0.671171736573759,0.727934368287542,
0.770051355331336,0.840365849439072,0.913615318512178,0.990483335368595,
1.),.UNSPECIFIED.);
#1433=B_SPLINE_CURVE_WITH_KNOTS('',3,(#55740,#55741,#55742,#55743,#55744,
#55745,#55746,#55747,#55748,#55749,#55750,#55751,#55752,#55753,#55754,#55755,
#55756,#55757,#55758,#55759,#55760,#55761,#55762,#55763,#55764,#55765,#55766,
#55767,#55768,#55769,#55770,#55771,#55772,#55773,#55774,#55775,#55776,#55777,
#55778,#55779,#55780,#55781,#55782,#55783,#55784,#55785,#55786,#55787,#55788),
 .UNSPECIFIED.,.F.,.F.,(4,3,3,3,3,3,3,3,3,3,3,3,3,3,3,3,4),(0.,0.0676604284666797,
0.135784861932871,0.20460798040263,0.25,0.319653372776603,0.389866426888844,
0.437436993869913,0.504795728664956,0.576501433821266,0.649794474217745,
0.722270051336813,0.75,0.817235207241609,0.882009314671392,0.943423886769645,
1.),.UNSPECIFIED.);
#1434=B_SPLINE_CURVE_WITH_KNOTS('',3,(#55789,#55790,#55791,#55792,#55793,
#55794),.UNSPECIFIED.,.F.,.F.,(4,2,4),(3.06785140422797E-6,0.00589378101525545,
0.00795361422578012),.UNSPECIFIED.);
#1435=B_SPLINE_CURVE_WITH_KNOTS('',5,(#55852,#55853,#55854,#55855,#55856,
#55857,#55858,#55859,#55860),.UNSPECIFIED.,.F.,.F.,(6,3,6),(0.,0.70000977750811,
1.),.UNSPECIFIED.);
#1436=B_SPLINE_CURVE_WITH_KNOTS('',3,(#55861,#55862,#55863,#55864,#55865,
#55866,#55867,#55868,#55869,#55870,#55871,#55872,#55873,#55874,#55875,#55876),
 .UNSPECIFIED.,.F.,.F.,(4,3,3,3,3,4),(0.,0.310429118799804,0.624797217736552,
0.699629793433942,0.877551619350703,1.),.UNSPECIFIED.);
#1437=B_SPLINE_CURVE_WITH_KNOTS('',5,(#55934,#55935,#55936,#55937,#55938,
#55939,#55940,#55941,#55942),.UNSPECIFIED.,.F.,.F.,(6,3,6),(0.,0.420445966361648,
1.),.UNSPECIFIED.);
#1438=B_SPLINE_CURVE_WITH_KNOTS('',3,(#55943,#55944,#55945,#55946,#55947,
#55948,#55949,#55950,#55951,#55952,#55953,#55954,#55955,#55956,#55957,#55958,
#55959,#55960,#55961,#55962,#55963,#55964,#55965,#55966,#55967,#55968,#55969,
#55970,#55971,#55972,#55973,#55974,#55975,#55976,#55977,#55978,#55979,#55980,
#55981,#55982,#55983,#55984,#55985,#55986,#55987,#55988,#55989,#55990,#55991,
#55992,#55993,#55994,#55995,#55996,#55997),.UNSPECIFIED.,.F.,.F.,(4,3,3,
3,3,3,3,3,3,3,3,3,3,3,3,3,3,3,4),(0.,0.0948842995124858,0.190085202830028,
0.285409913484093,0.378133360715178,0.423302343602271,0.49609374999998,
0.499550986594487,0.49999999999998,0.557470780273894,0.613908528426856,
0.669611200661826,0.724088620846792,0.74999999999999,0.802588612033394,
0.853469118232013,0.903394163463505,0.951763239695998,1.),.UNSPECIFIED.);
#1439=B_SPLINE_CURVE_WITH_KNOTS('',3,(#56052,#56053,#56054,#56055,#56056,
#56057,#56058,#56059,#56060,#56061,#56062,#56063,#56064),.UNSPECIFIED.,
 .F.,.F.,(4,3,3,3,4),(0.,0.394963839602928,0.529543868594593,0.809415847321762,
1.),.UNSPECIFIED.);
#1440=B_SPLINE_CURVE_WITH_KNOTS('',3,(#56070,#56071,#56072,#56073,#56074,
#56075,#56076,#56077,#56078,#56079,#56080,#56081,#56082,#56083,#56084,#56085,
#56086,#56087,#56088,#56089,#56090,#56091,#56092,#56093,#56094,#56095,#56096,
#56097,#56098,#56099,#56100,#56101,#56102,#56103,#56104,#56105,#56106,#56107,
#56108,#56109,#56110,#56111,#56112,#56113,#56114,#56115,#56116,#56117,#56118),
 .UNSPECIFIED.,.F.,.F.,(4,3,3,3,3,3,3,3,3,3,3,3,3,3,3,3,4),(1.85172896462502E-10,
0.0694020177073269,0.138700016353406,0.207902958120875,0.27699293171057,
0.346014007423806,0.414958141095058,0.437324236739737,0.50765870411793,
0.575665169523303,0.643655775825584,0.711642092460888,0.779635683547978,
0.847672155976127,0.915732654483638,0.983852595780531,0.999999975765285),
 .UNSPECIFIED.);
#1441=B_SPLINE_CURVE_WITH_KNOTS('',3,(#56120,#56121,#56122,#56123,#56124,
#56125,#56126,#56127,#56128,#56129,#56130,#56131,#56132,#56133,#56134,#56135,
#56136,#56137,#56138),.UNSPECIFIED.,.F.,.F.,(4,3,3,3,3,3,4),(1.56090158029,
1.97847928202979,2.40343448569499,2.52299916049,2.76927079046744,2.93187648001,
2.93530749734),.UNSPECIFIED.);
#1442=B_SPLINE_CURVE_WITH_KNOTS('',5,(#56140,#56141,#56142,#56143,#56144,
#56145,#56146,#56147,#56148,#56149,#56150,#56151,#56152,#56153,#56154),
 .UNSPECIFIED.,.F.,.F.,(6,3,3,3,6),(3.22008961045,5.63866638969,7.2508178231,
8.95983620486,8.97249770267),.UNSPECIFIED.);
#1443=B_SPLINE_CURVE_WITH_KNOTS('',3,(#56166,#56167,#56168,#56169,#56170,
#56171,#56172,#56173,#56174,#56175,#56176,#56177,#56178,#56179,#56180,#56181,
#56182,#56183,#56184,#56185,#56186,#56187),.UNSPECIFIED.,.F.,.F.,(4,3,3,
3,3,3,3,4),(0.595163146152,1.08064893071393,1.40157444353,1.97827761057397,
2.70225888679198,3.29249008213981,3.42624016301,3.46611471078),
 .UNSPECIFIED.);
#1444=B_SPLINE_CURVE_WITH_KNOTS('',3,(#56193,#56194,#56195,#56196,#56197,
#56198,#56199,#56200,#56201,#56202,#56203,#56204,#56205,#56206,#56207,#56208,
#56209,#56210,#56211,#56212,#56213,#56214,#56215,#56216,#56217,#56218,#56219,
#56220),.UNSPECIFIED.,.F.,.F.,(4,3,3,3,3,3,3,3,3,4),(0.0737511725012,0.120582377595235,
0.156939526058,0.213622987505703,0.240560274088,0.296963246825959,0.324594419288,
0.356043030607,0.361284468446,0.36600685554),.UNSPECIFIED.);
#1445=B_SPLINE_CURVE_WITH_KNOTS('',5,(#56226,#56227,#56228,#56229,#56230,
#56231,#56232,#56233,#56234),.UNSPECIFIED.,.F.,.F.,(6,3,6),(7.03940069458791E-8,
0.360882270523195,1.),.UNSPECIFIED.);
#1446=B_SPLINE_CURVE_WITH_KNOTS('',3,(#56236,#56237,#56238,#56239,#56240,
#56241,#56242,#56243,#56244,#56245,#56246,#56247,#56248,#56249,#56250,#56251,
#56252,#56253,#56254,#56255,#56256,#56257,#56258,#56259,#56260,#56261,#56262,
#56263,#56264,#56265,#56266,#56267,#56268,#56269,#56270,#56271,#56272,#56273,
#56274,#56275,#56276,#56277,#56278,#56279,#56280,#56281,#56282,#56283,#56284,
#56285,#56286,#56287,#56288,#56289,#56290,#56291,#56292,#56293,#56294,#56295,
#56296,#56297,#56298,#56299,#56300,#56301,#56302,#56303,#56304,#56305,#56306,
#56307,#56308,#56309,#56310,#56311,#56312,#56313,#56314,#56315,#56316,#56317,
#56318,#56319,#56320,#56321,#56322,#56323,#56324,#56325,#56326),
 .UNSPECIFIED.,.F.,.F.,(4,3,3,3,3,3,3,3,3,3,3,3,3,3,3,3,3,3,3,3,3,3,3,3,
3,3,3,3,3,3,4),(7.24577941808172E-8,0.0512940021506198,0.103630723688098,
0.125000000000011,0.179593986387468,0.187500000000017,0.218750000000019,
0.234375000000021,0.242187500000021,0.248234663203568,0.250000000000022,
0.290930951812491,0.331940468398339,0.337768593684404,0.375000000000028,
0.417102508489356,0.459628379401037,0.496093750000034,0.498046875000034,
0.499027252197299,0.499516483396325,0.499778569489927,0.49997746513499,
0.500101039385769,0.576525095455382,0.652447461005577,0.72856119175266,
0.811259005869195,0.889711323751863,0.970201629824757,1.),.UNSPECIFIED.);
#1447=B_SPLINE_CURVE_WITH_KNOTS('',3,(#56332,#56333,#56334,#56335,#56336,
#56337,#56338,#56339,#56340,#56341,#56342,#56343,#56344,#56345,#56346,#56347,
#56348,#56349,#56350,#56351,#56352,#56353,#56354,#56355,#56356,#56357,#56358,
#56359),.UNSPECIFIED.,.F.,.F.,(4,3,3,3,3,3,3,3,3,4),(0.0737511725012,0.120582377595233,
0.156939526058,0.213622987505703,0.240560274088,0.296963246825932,0.324594419288,
0.356043030607,0.361284468446,0.36600685554),.UNSPECIFIED.);
#1448=B_SPLINE_CURVE_WITH_KNOTS('',3,(#56365,#56366,#56367,#56368,#56369,
#56370,#56371,#56372,#56373,#56374,#56375,#56376,#56377,#56378,#56379,#56380,
#56381,#56382,#56383,#56384,#56385,#56386),.UNSPECIFIED.,.F.,.F.,(4,3,3,
3,3,3,3,4),(0.595163146152,1.080648930714,1.40157444353,1.97827761057532,
2.70225888679266,3.29249008214117,3.42624016301,3.46611471078),
 .UNSPECIFIED.);
#1449=B_SPLINE_CURVE_WITH_KNOTS('',5,(#56426,#56427,#56428,#56429,#56430,
#56431),.UNSPECIFIED.,.F.,.F.,(6,6),(0.,1.),.UNSPECIFIED.);
#1450=B_SPLINE_CURVE_WITH_KNOTS('',3,(#56470,#56471,#56472,#56473,#56474,
#56475,#56476,#56477,#56478,#56479,#56480,#56481,#56482,#56483,#56484,#56485),
 .UNSPECIFIED.,.F.,.F.,(4,3,3,3,3,4),(0.,0.207236770649871,0.449803912628789,
0.724901956314395,0.939507656121702,1.),.UNSPECIFIED.);
#1451=B_SPLINE_CURVE_WITH_KNOTS('',5,(#56581,#56582,#56583,#56584,#56585,
#56586,#56587,#56588,#56589),.UNSPECIFIED.,.F.,.F.,(6,3,6),(0.,0.570764276223718,
1.),.UNSPECIFIED.);
#1452=B_SPLINE_CURVE_WITH_KNOTS('',3,(#56622,#56623,#56624,#56625),
 .UNSPECIFIED.,.F.,.F.,(4,4),(1.03670984253,1.04687754685),
 .UNSPECIFIED.);
#1453=B_SPLINE_CURVE_WITH_KNOTS('',5,(#56681,#56682,#56683,#56684,#56685,
#56686,#56687,#56688,#56689),.UNSPECIFIED.,.F.,.F.,(6,3,6),(2.76258508985744E-8,
0.359893824506783,1.),.UNSPECIFIED.);
#1454=B_SPLINE_CURVE_WITH_KNOTS('',3,(#56747,#56748,#56749,#56750,#56751,
#56752,#56753,#56754,#56755,#56756,#56757,#56758,#56759,#56760,#56761,#56762,
#56763,#56764,#56765,#56766,#56767,#56768,#56769,#56770,#56771,#56772,#56773,
#56774,#56775,#56776,#56777,#56778,#56779,#56780,#56781,#56782,#56783,#56784,
#56785,#56786,#56787,#56788,#56789,#56790,#56791,#56792,#56793,#56794,#56795,
#56796,#56797,#56798,#56799,#56800,#56801,#56802,#56803,#56804,#56805,#56806,
#56807,#56808,#56809,#56810,#56811,#56812,#56813,#56814,#56815,#56816,#56817,
#56818,#56819,#56820,#56821,#56822,#56823,#56824,#56825,#56826,#56827,#56828,
#56829,#56830,#56831,#56832,#56833,#56834,#56835,#56836,#56837,#56838,#56839,
#56840,#56841,#56842,#56843),.UNSPECIFIED.,.F.,.F.,(4,3,3,3,3,3,3,3,3,3,
3,3,3,3,3,3,3,3,3,3,3,3,3,3,3,3,3,3,3,3,3,3,4),(3.38230551104713E-8,0.0661085210548239,
0.130590121983721,0.196883083653977,0.250000000000032,0.331618079659059,
0.375000000000048,0.377020948134889,0.437500000000056,0.46875000000006,
0.484375000000062,0.492187500000063,0.496093750000063,0.498046875000064,
0.500000000000064,0.528452399150718,0.557731830669541,0.587365305364137,
0.617341747325477,0.625000000000077,0.65576171875008,0.685986908865822,
0.717016891932956,0.732531883466523,0.740289379233306,0.744677047469246,
0.747820353842888,0.748046875000089,0.750000000000089,0.812529999338103,
0.876411794971792,0.942357563683105,1.),.UNSPECIFIED.);
#1455=B_SPLINE_CURVE_WITH_KNOTS('',3,(#56876,#56877,#56878,#56879),
 .UNSPECIFIED.,.F.,.F.,(4,4),(1.03670984253,1.04687754685),
 .UNSPECIFIED.);
#1456=B_SPLINE_CURVE_WITH_KNOTS('',3,(#56936,#56937,#56938,#56939,#56940,
#56941,#56942,#56943,#56944,#56945,#56946,#56947,#56948,#56949,#56950,#56951,
#56952,#56953,#56954,#56955,#56956,#56957),.UNSPECIFIED.,.F.,.F.,(4,3,3,
3,3,3,3,4),(0.,0.164952116135099,0.340839944519898,0.529302228005302,0.588843624721089,
0.765500311524726,0.902274076507374,1.),.UNSPECIFIED.);
#1457=B_SPLINE_CURVE_WITH_KNOTS('',3,(#57035,#57036,#57037,#57038),
 .UNSPECIFIED.,.F.,.F.,(4,4),(0.,1.),.UNSPECIFIED.);
#1458=B_SPLINE_CURVE_WITH_KNOTS('',3,(#57077,#57078,#57079,#57080,#57081,
#57082,#57083,#57084,#57085,#57086,#57087,#57088,#57089),.UNSPECIFIED.,
 .F.,.F.,(4,3,3,3,4),(0.,0.302812745334426,0.611175192673633,0.89306501651859,
0.999999645076241),.UNSPECIFIED.);
#1459=B_SPLINE_CURVE_WITH_KNOTS('',3,(#57148,#57149,#57150,#57151,#57152,
#57153,#57154,#57155,#57156,#57157,#57158,#57159,#57160,#57161,#57162,#57163),
 .UNSPECIFIED.,.F.,.F.,(4,3,3,3,3,4),(0.,0.265384459220342,0.530768918440684,
0.765384459220342,0.96786815318798,1.),.UNSPECIFIED.);
#1460=B_SPLINE_CURVE_WITH_KNOTS('',3,(#57220,#57221,#57222,#57223,#57224,
#57225,#57226,#57227,#57228,#57229,#57230,#57231,#57232,#57233,#57234,#57235,
#57236,#57237,#57238,#57239,#57240,#57241,#57242,#57243,#57244,#57245,#57246,
#57247,#57248,#57249,#57250,#57251,#57252,#57253,#57254,#57255,#57256,#57257,
#57258,#57259,#57260,#57261,#57262,#57263,#57264,#57265,#57266,#57267,#57268),
 .UNSPECIFIED.,.F.,.F.,(4,3,3,3,3,3,3,3,3,3,3,3,3,3,3,3,4),(0.,0.076900072948699,
0.152363307739898,0.225801136908131,0.250000000000011,0.321091761249945,
0.390059812546072,0.430282639543951,0.492187500000021,0.49823793040025,
0.500000000000021,0.588209486901966,0.676836259388543,0.75000000000001,
0.850717574299832,0.949663866823197,1.),.UNSPECIFIED.);
#1461=B_SPLINE_CURVE_WITH_KNOTS('',3,(#57325,#57326,#57327,#57328,#57329,
#57330,#57331,#57332,#57333,#57334,#57335,#57336,#57337,#57338,#57339,#57340),
 .UNSPECIFIED.,.F.,.F.,(4,3,3,3,3,4),(0.,0.225369815259222,0.483809499590606,
0.692086551442115,0.90274357771896,1.),.UNSPECIFIED.);
#1462=B_SPLINE_CURVE_WITH_KNOTS('',3,(#57395,#57396,#57397,#57398,#57399,
#57400,#57401,#57402,#57403,#57404,#57405,#57406,#57407,#57408,#57409,#57410,
#57411,#57412,#57413,#57414,#57415,#57416,#57417,#57418,#57419,#57420,#57421,
#57422,#57423,#57424,#57425,#57426,#57427,#57428,#57429,#57430,#57431,#57432,
#57433,#57434,#57435,#57436,#57437,#57438,#57439,#57440,#57441,#57442,#57443,
#57444,#57445,#57446,#57447,#57448,#57449,#57450,#57451,#57452,#57453,#57454,
#57455,#57456,#57457,#57458,#57459,#57460,#57461,#57462,#57463,#57464,#57465,
#57466,#57467,#57468,#57469,#57470,#57471,#57472,#57473,#57474,#57475,#57476,
#57477,#57478,#57479,#57480,#57481,#57482,#57483,#57484,#57485,#57486,#57487,
#57488,#57489,#57490,#57491,#57492,#57493,#57494,#57495,#57496,#57497,#57498,
#57499,#57500,#57501,#57502,#57503,#57504,#57505,#57506,#57507,#57508,#57509,
#57510,#57511,#57512,#57513,#57514,#57515,#57516,#57517,#57518,#57519,#57520,
#57521,#57522,#57523,#57524,#57525,#57526,#57527),.UNSPECIFIED.,.F.,.F.,
(4,3,3,3,3,3,3,3,3,3,3,3,3,3,3,3,3,3,3,3,3,3,3,3,3,3,3,3,3,3,3,3,3,3,3,
3,3,3,3,3,3,3,3,3,4),(0.,0.0693839705898158,0.125000000000017,0.187500000000025,
0.218750000000029,0.234375000000031,0.242187500000032,0.246093750000032,
0.248046875000033,0.250000000000033,0.284634412927758,0.318997381436396,
0.352787785209862,0.375000000000025,0.407562306964218,0.437500000000021,
0.452477592263182,0.468750000000019,0.484375000000018,0.488525390625018,
0.49056816101076,0.491821161209957,0.49257078993287,0.496593121340169,0.498572862579699,
0.499804266710987,0.500267006315948,0.537432084962121,0.575039819621256,
0.61324330769772,0.652808414709024,0.693105958577131,0.721552979288567,
0.735776489644284,0.742888244822143,0.744666183616608,0.745999637712457,
0.746288571798483,0.749674538265303,0.750000000000002,0.812500000000002,
0.873474261559203,0.933084762257831,0.990543844166144,1.),.UNSPECIFIED.);
#1463=B_SPLINE_CURVE_WITH_KNOTS('',3,(#57583,#57584,#57585,#57586,#57587,
#57588,#57589,#57590,#57591,#57592,#57593,#57594,#57595),.UNSPECIFIED.,
 .F.,.F.,(4,3,3,3,4),(0.,0.242939372158968,0.486368987740473,0.730792780934889,
0.91853342156656),.UNSPECIFIED.);
#1464=B_SPLINE_CURVE_WITH_KNOTS('',3,(#57597,#57598,#57599,#57600),
 .UNSPECIFIED.,.F.,.F.,(4,4),(0.91853342156656,1.),.UNSPECIFIED.);
#1465=B_SPLINE_CURVE_WITH_KNOTS('',5,(#57602,#57603,#57604,#57605,#57606,
#57607,#57608,#57609,#57610),.UNSPECIFIED.,.F.,.F.,(6,3,6),(0.,0.0437456503794834,
1.),.UNSPECIFIED.);
#1466=B_SPLINE_CURVE_WITH_KNOTS('',3,(#57668,#57669,#57670,#57671,#57672,
#57673),.UNSPECIFIED.,.F.,.F.,(4,2,4),(0.,0.216978430582008,0.361147653076782),
 .UNSPECIFIED.);
#1467=B_SPLINE_CURVE_WITH_KNOTS('',3,(#57733,#57734,#57735,#57736,#57737,
#57738),.UNSPECIFIED.,.F.,.F.,(4,2,4),(-0.258354222257529,-0.129177105593006,
0.),.UNSPECIFIED.);
#1468=B_SPLINE_CURVE_WITH_KNOTS('',3,(#57813,#57814,#57815,#57816,#57817,
#57818),.UNSPECIFIED.,.F.,.F.,(4,2,4),(-0.258354222257541,-0.129177105593007,
0.),.UNSPECIFIED.);
#2044=SHAPE_REPRESENTATION_RELATIONSHIP('SRR','None',#98341,#2054);
#2054=ADVANCED_BREP_SHAPE_REPRESENTATION('',(#2074),#98293);
#2064=STYLED_ITEM('',(#98399),#2074);
#2074=MANIFOLD_SOLID_BREP('Body1',#34168);
#2084=PLANE('',#34307);
#2085=PLANE('',#34349);
#2086=PLANE('',#34352);
#2087=PLANE('',#34371);
#2088=PLANE('',#34385);
#2089=PLANE('',#34393);
#2090=PLANE('',#34401);
#2091=PLANE('',#34419);
#2092=PLANE('',#34437);
#2093=PLANE('',#34445);
#2094=PLANE('',#34453);
#2095=PLANE('',#34471);
#2096=PLANE('',#34479);
#2097=PLANE('',#34487);
#2098=PLANE('',#34505);
#2099=PLANE('',#34523);
#2100=PLANE('',#34531);
#2101=PLANE('',#34543);
#2102=PLANE('',#34544);
#2103=PLANE('',#34545);
#2104=PLANE('',#34550);
#2105=PLANE('',#34551);
#2106=PLANE('',#34708);
#2107=PLANE('',#34721);
#2108=PLANE('',#34722);
#2109=PLANE('',#34725);
#2110=PLANE('',#34728);
#2111=PLANE('',#34733);
#2112=PLANE('',#34736);
#2113=PLANE('',#34739);
#2114=PLANE('',#34742);
#2115=PLANE('',#34745);
#2116=PLANE('',#34746);
#2117=PLANE('',#34760);
#2118=PLANE('',#34769);
#2119=PLANE('',#34800);
#2120=PLANE('',#34822);
#2522=CYLINDRICAL_SURFACE('',#34304,0.3);
#2523=CYLINDRICAL_SURFACE('',#34350,0.3);
#2524=CYLINDRICAL_SURFACE('',#34353,0.3);
#2525=CYLINDRICAL_SURFACE('',#34359,0.3);
#2526=CYLINDRICAL_SURFACE('',#34361,0.3);
#2527=CYLINDRICAL_SURFACE('',#34363,0.3);
#2528=CYLINDRICAL_SURFACE('',#34368,0.3);
#2529=CYLINDRICAL_SURFACE('',#34372,15.9);
#2530=CYLINDRICAL_SURFACE('',#34381,0.3);
#2531=CYLINDRICAL_SURFACE('',#34383,0.100000000000003);
#2532=CYLINDRICAL_SURFACE('',#34389,0.300000000000001);
#2533=CYLINDRICAL_SURFACE('',#34391,0.100000000000003);
#2534=CYLINDRICAL_SURFACE('',#34397,0.299999999999999);
#2535=CYLINDRICAL_SURFACE('',#34399,0.1);
#2536=CYLINDRICAL_SURFACE('',#34405,0.3);
#2537=CYLINDRICAL_SURFACE('',#34410,15.9);
#2538=CYLINDRICAL_SURFACE('',#34415,0.5);
#2539=CYLINDRICAL_SURFACE('',#34417,0.0999999999999994);
#2540=CYLINDRICAL_SURFACE('',#34423,0.499999999999999);
#2541=CYLINDRICAL_SURFACE('',#34428,15.9);
#2542=CYLINDRICAL_SURFACE('',#34433,0.3);
#2543=CYLINDRICAL_SURFACE('',#34435,0.100000000000003);
#2544=CYLINDRICAL_SURFACE('',#34441,0.3);
#2545=CYLINDRICAL_SURFACE('',#34443,0.1);
#2546=CYLINDRICAL_SURFACE('',#34449,0.300000000000001);
#2547=CYLINDRICAL_SURFACE('',#34451,0.1);
#2548=CYLINDRICAL_SURFACE('',#34457,0.3);
#2549=CYLINDRICAL_SURFACE('',#34459,15.9);
#2550=CYLINDRICAL_SURFACE('',#34467,0.3);
#2551=CYLINDRICAL_SURFACE('',#34469,0.100000000000003);
#2552=CYLINDRICAL_SURFACE('',#34475,0.300000000000001);
#2553=CYLINDRICAL_SURFACE('',#34477,0.100000000000003);
#2554=CYLINDRICAL_SURFACE('',#34483,0.299999999999999);
#2555=CYLINDRICAL_SURFACE('',#34485,0.1);
#2556=CYLINDRICAL_SURFACE('',#34491,0.3);
#2557=CYLINDRICAL_SURFACE('',#34496,15.9);
#2558=CYLINDRICAL_SURFACE('',#34501,0.499999999999999);
#2559=CYLINDRICAL_SURFACE('',#34503,0.100000000000003);
#2560=CYLINDRICAL_SURFACE('',#34509,0.5);
#2561=CYLINDRICAL_SURFACE('',#34514,15.9);
#2562=CYLINDRICAL_SURFACE('',#34519,0.300000000000001);
#2563=CYLINDRICAL_SURFACE('',#34521,0.100000000000003);
#2564=CYLINDRICAL_SURFACE('',#34527,0.3);
#2565=CYLINDRICAL_SURFACE('',#34529,0.1);
#2566=CYLINDRICAL_SURFACE('',#34535,0.3);
#2567=CYLINDRICAL_SURFACE('',#34540,0.3);
#2568=CYLINDRICAL_SURFACE('',#34542,0.1);
#2569=CYLINDRICAL_SURFACE('',#34556,0.999997171346093);
#2570=CYLINDRICAL_SURFACE('',#34601,0.999997171346093);
#2571=CYLINDRICAL_SURFACE('',#34609,0.1);
#2572=CYLINDRICAL_SURFACE('',#34614,0.1);
#2573=CYLINDRICAL_SURFACE('',#34619,0.100000000000003);
#2574=CYLINDRICAL_SURFACE('',#34630,0.100000000000003);
#2575=CYLINDRICAL_SURFACE('',#34641,0.1);
#2576=CYLINDRICAL_SURFACE('',#34646,0.100000000000003);
#2577=CYLINDRICAL_SURFACE('',#34651,0.100000000000003);
#2578=CYLINDRICAL_SURFACE('',#34662,0.1);
#2579=CYLINDRICAL_SURFACE('',#34667,0.1);
#2580=CYLINDRICAL_SURFACE('',#34672,0.100000000000003);
#2581=CYLINDRICAL_SURFACE('',#34683,0.0999999999999994);
#2582=CYLINDRICAL_SURFACE('',#34694,0.1);
#2583=CYLINDRICAL_SURFACE('',#34699,0.100000000000003);
#2584=CYLINDRICAL_SURFACE('',#34707,0.100000000000003);
#2585=CYLINDRICAL_SURFACE('',#34719,14.4);
#2586=CYLINDRICAL_SURFACE('',#34723,1.5);
#2587=CYLINDRICAL_SURFACE('',#34726,1.5);
#2588=CYLINDRICAL_SURFACE('',#34729,1.5);
#2589=CYLINDRICAL_SURFACE('',#34731,1.5);
#2590=CYLINDRICAL_SURFACE('',#34734,14.4);
#2591=CYLINDRICAL_SURFACE('',#34737,1.5);
#2592=CYLINDRICAL_SURFACE('',#34740,1.5);
#2593=CYLINDRICAL_SURFACE('',#34743,1.5);
#2594=CYLINDRICAL_SURFACE('',#34748,1.5);
#2595=CYLINDRICAL_SURFACE('',#34755,4.00389099741);
#2596=CYLINDRICAL_SURFACE('',#34756,4.00389099741);
#2597=CYLINDRICAL_SURFACE('',#34758,0.3);
#2598=CYLINDRICAL_SURFACE('',#34762,0.3);
#2599=CYLINDRICAL_SURFACE('',#34764,3.89050581799);
#2600=CYLINDRICAL_SURFACE('',#34767,0.3);
#2601=CYLINDRICAL_SURFACE('',#34808,16.1875296363);
#2602=CYLINDRICAL_SURFACE('',#34810,26.2647265892);
#2603=CYLINDRICAL_SURFACE('',#34812,12.2773059952);
#2604=CYLINDRICAL_SURFACE('',#34814,12.2773059952);
#2605=CYLINDRICAL_SURFACE('',#34816,26.2647265892);
#2606=CYLINDRICAL_SURFACE('',#34818,16.1875296363);
#2607=CYLINDRICAL_SURFACE('',#34820,5.);
#3284=FACE_OUTER_BOUND('',#5424,.T.);
#3285=FACE_OUTER_BOUND('',#5425,.T.);
#3286=FACE_OUTER_BOUND('',#5429,.T.);
#3287=FACE_OUTER_BOUND('',#5430,.T.);
#3288=FACE_OUTER_BOUND('',#5431,.T.);
#3289=FACE_OUTER_BOUND('',#5432,.T.);
#3290=FACE_OUTER_BOUND('',#5433,.T.);
#3291=FACE_OUTER_BOUND('',#5434,.T.);
#3292=FACE_OUTER_BOUND('',#5435,.T.);
#3293=FACE_OUTER_BOUND('',#5436,.T.);
#3294=FACE_OUTER_BOUND('',#5437,.T.);
#3295=FACE_OUTER_BOUND('',#5438,.T.);
#3296=FACE_OUTER_BOUND('',#5439,.T.);
#3297=FACE_OUTER_BOUND('',#5440,.T.);
#3298=FACE_OUTER_BOUND('',#5441,.T.);
#3299=FACE_OUTER_BOUND('',#5442,.T.);
#3300=FACE_OUTER_BOUND('',#5443,.T.);
#3301=FACE_OUTER_BOUND('',#5444,.T.);
#3302=FACE_OUTER_BOUND('',#5445,.T.);
#3303=FACE_OUTER_BOUND('',#5446,.T.);
#3304=FACE_OUTER_BOUND('',#5447,.T.);
#3305=FACE_OUTER_BOUND('',#5448,.T.);
#3306=FACE_OUTER_BOUND('',#5449,.T.);
#3307=FACE_OUTER_BOUND('',#5450,.T.);
#3308=FACE_OUTER_BOUND('',#5451,.T.);
#3309=FACE_OUTER_BOUND('',#5452,.T.);
#3310=FACE_OUTER_BOUND('',#5453,.T.);
#3311=FACE_OUTER_BOUND('',#5454,.T.);
#3312=FACE_OUTER_BOUND('',#5455,.T.);
#3313=FACE_OUTER_BOUND('',#5456,.T.);
#3314=FACE_OUTER_BOUND('',#5457,.T.);
#3315=FACE_OUTER_BOUND('',#5458,.T.);
#3316=FACE_OUTER_BOUND('',#5459,.T.);
#3317=FACE_OUTER_BOUND('',#5460,.T.);
#3318=FACE_OUTER_BOUND('',#5461,.T.);
#3319=FACE_OUTER_BOUND('',#5462,.T.);
#3320=FACE_OUTER_BOUND('',#5463,.T.);
#3321=FACE_OUTER_BOUND('',#5464,.T.);
#3322=FACE_OUTER_BOUND('',#5465,.T.);
#3323=FACE_OUTER_BOUND('',#5466,.T.);
#3324=FACE_OUTER_BOUND('',#5467,.T.);
#3325=FACE_OUTER_BOUND('',#5468,.T.);
#3326=FACE_OUTER_BOUND('',#5469,.T.);
#3327=FACE_OUTER_BOUND('',#5470,.T.);
#3328=FACE_OUTER_BOUND('',#5471,.T.);
#3329=FACE_OUTER_BOUND('',#5472,.T.);
#3330=FACE_OUTER_BOUND('',#5473,.T.);
#3331=FACE_OUTER_BOUND('',#5474,.T.);
#3332=FACE_OUTER_BOUND('',#5475,.T.);
#3333=FACE_OUTER_BOUND('',#5476,.T.);
#3334=FACE_OUTER_BOUND('',#5477,.T.);
#3335=FACE_OUTER_BOUND('',#5478,.T.);
#3336=FACE_OUTER_BOUND('',#5479,.T.);
#3337=FACE_OUTER_BOUND('',#5480,.T.);
#3338=FACE_OUTER_BOUND('',#5481,.T.);
#3339=FACE_OUTER_BOUND('',#5482,.T.);
#3340=FACE_OUTER_BOUND('',#5483,.T.);
#3341=FACE_OUTER_BOUND('',#5484,.T.);
#3342=FACE_OUTER_BOUND('',#5485,.T.);
#3343=FACE_OUTER_BOUND('',#5486,.T.);
#3344=FACE_OUTER_BOUND('',#5487,.T.);
#3345=FACE_OUTER_BOUND('',#5488,.T.);
#3346=FACE_OUTER_BOUND('',#5489,.T.);
#3347=FACE_OUTER_BOUND('',#5490,.T.);
#3348=FACE_OUTER_BOUND('',#5491,.T.);
#3349=FACE_OUTER_BOUND('',#5492,.T.);
#3350=FACE_OUTER_BOUND('',#5493,.T.);
#3351=FACE_OUTER_BOUND('',#5494,.T.);
#3352=FACE_OUTER_BOUND('',#5495,.T.);
#3353=FACE_OUTER_BOUND('',#5496,.T.);
#3354=FACE_OUTER_BOUND('',#5497,.T.);
#3355=FACE_OUTER_BOUND('',#5498,.T.);
#3356=FACE_OUTER_BOUND('',#5499,.T.);
#3357=FACE_OUTER_BOUND('',#5500,.T.);
#3358=FACE_OUTER_BOUND('',#5501,.T.);
#3359=FACE_OUTER_BOUND('',#5502,.T.);
#3360=FACE_OUTER_BOUND('',#5503,.T.);
#3361=FACE_OUTER_BOUND('',#5504,.T.);
#3362=FACE_OUTER_BOUND('',#5505,.T.);
#3363=FACE_OUTER_BOUND('',#5506,.T.);
#3364=FACE_OUTER_BOUND('',#5507,.T.);
#3365=FACE_OUTER_BOUND('',#5508,.T.);
#3366=FACE_OUTER_BOUND('',#5509,.T.);
#3367=FACE_OUTER_BOUND('',#5510,.T.);
#3368=FACE_OUTER_BOUND('',#5511,.T.);
#3369=FACE_OUTER_BOUND('',#5512,.T.);
#3370=FACE_OUTER_BOUND('',#5513,.T.);
#3371=FACE_OUTER_BOUND('',#5514,.T.);
#3372=FACE_OUTER_BOUND('',#5515,.T.);
#3373=FACE_OUTER_BOUND('',#5516,.T.);
#3374=FACE_OUTER_BOUND('',#5517,.T.);
#3375=FACE_OUTER_BOUND('',#5518,.T.);
#3376=FACE_OUTER_BOUND('',#5519,.T.);
#3377=FACE_OUTER_BOUND('',#5520,.T.);
#3378=FACE_OUTER_BOUND('',#5521,.T.);
#3379=FACE_OUTER_BOUND('',#5522,.T.);
#3380=FACE_OUTER_BOUND('',#5523,.T.);
#3381=FACE_OUTER_BOUND('',#5524,.T.);
#3382=FACE_OUTER_BOUND('',#5525,.T.);
#3383=FACE_OUTER_BOUND('',#5526,.T.);
#3384=FACE_OUTER_BOUND('',#5527,.T.);
#3385=FACE_OUTER_BOUND('',#5528,.T.);
#3386=FACE_OUTER_BOUND('',#5529,.T.);
#3387=FACE_OUTER_BOUND('',#5530,.T.);
#3388=FACE_OUTER_BOUND('',#5531,.T.);
#3389=FACE_OUTER_BOUND('',#5532,.T.);
#3390=FACE_OUTER_BOUND('',#5533,.T.);
#3391=FACE_OUTER_BOUND('',#5534,.T.);
#3392=FACE_OUTER_BOUND('',#5535,.T.);
#3393=FACE_OUTER_BOUND('',#5536,.T.);
#3394=FACE_OUTER_BOUND('',#5537,.T.);
#3395=FACE_OUTER_BOUND('',#5538,.T.);
#3396=FACE_OUTER_BOUND('',#5539,.T.);
#3397=FACE_OUTER_BOUND('',#5540,.T.);
#3398=FACE_OUTER_BOUND('',#5541,.T.);
#3399=FACE_OUTER_BOUND('',#5542,.T.);
#3400=FACE_OUTER_BOUND('',#5543,.T.);
#3401=FACE_OUTER_BOUND('',#5544,.T.);
#3402=FACE_OUTER_BOUND('',#5545,.T.);
#3403=FACE_OUTER_BOUND('',#5546,.T.);
#3404=FACE_OUTER_BOUND('',#5547,.T.);
#3405=FACE_OUTER_BOUND('',#5548,.T.);
#3406=FACE_OUTER_BOUND('',#5549,.T.);
#3407=FACE_OUTER_BOUND('',#5550,.T.);
#3408=FACE_OUTER_BOUND('',#5551,.T.);
#3409=FACE_OUTER_BOUND('',#5552,.T.);
#3410=FACE_OUTER_BOUND('',#5553,.T.);
#3411=FACE_OUTER_BOUND('',#5554,.T.);
#3412=FACE_OUTER_BOUND('',#5555,.T.);
#3413=FACE_OUTER_BOUND('',#5556,.T.);
#3414=FACE_OUTER_BOUND('',#5557,.T.);
#3415=FACE_OUTER_BOUND('',#5558,.T.);
#3416=FACE_OUTER_BOUND('',#5559,.T.);
#3417=FACE_OUTER_BOUND('',#5560,.T.);
#3418=FACE_OUTER_BOUND('',#5561,.T.);
#3419=FACE_OUTER_BOUND('',#5562,.T.);
#3420=FACE_OUTER_BOUND('',#5563,.T.);
#3421=FACE_OUTER_BOUND('',#5564,.T.);
#3422=FACE_OUTER_BOUND('',#5565,.T.);
#3423=FACE_OUTER_BOUND('',#5566,.T.);
#3424=FACE_OUTER_BOUND('',#5567,.T.);
#3425=FACE_OUTER_BOUND('',#5568,.T.);
#3426=FACE_OUTER_BOUND('',#5569,.T.);
#3427=FACE_OUTER_BOUND('',#5570,.T.);
#3428=FACE_OUTER_BOUND('',#5571,.T.);
#3429=FACE_OUTER_BOUND('',#5572,.T.);
#3430=FACE_OUTER_BOUND('',#5573,.T.);
#3431=FACE_OUTER_BOUND('',#5574,.T.);
#3432=FACE_OUTER_BOUND('',#5575,.T.);
#3433=FACE_OUTER_BOUND('',#5576,.T.);
#3434=FACE_OUTER_BOUND('',#5577,.T.);
#3435=FACE_OUTER_BOUND('',#5578,.T.);
#3436=FACE_OUTER_BOUND('',#5579,.T.);
#3437=FACE_OUTER_BOUND('',#5580,.T.);
#3438=FACE_OUTER_BOUND('',#5581,.T.);
#3439=FACE_OUTER_BOUND('',#5582,.T.);
#3440=FACE_OUTER_BOUND('',#5583,.T.);
#3441=FACE_OUTER_BOUND('',#5584,.T.);
#3442=FACE_OUTER_BOUND('',#5585,.T.);
#3443=FACE_OUTER_BOUND('',#5586,.T.);
#3444=FACE_OUTER_BOUND('',#5587,.T.);
#3445=FACE_OUTER_BOUND('',#5588,.T.);
#3446=FACE_OUTER_BOUND('',#5589,.T.);
#3447=FACE_OUTER_BOUND('',#5590,.T.);
#3448=FACE_OUTER_BOUND('',#5591,.T.);
#3449=FACE_OUTER_BOUND('',#5592,.T.);
#3450=FACE_OUTER_BOUND('',#5593,.T.);
#3451=FACE_OUTER_BOUND('',#5594,.T.);
#3452=FACE_OUTER_BOUND('',#5595,.T.);
#3453=FACE_OUTER_BOUND('',#5596,.T.);
#3454=FACE_OUTER_BOUND('',#5597,.T.);
#3455=FACE_OUTER_BOUND('',#5598,.T.);
#3456=FACE_OUTER_BOUND('',#5599,.T.);
#3457=FACE_OUTER_BOUND('',#5600,.T.);
#3458=FACE_OUTER_BOUND('',#5601,.T.);
#3459=FACE_OUTER_BOUND('',#5602,.T.);
#3460=FACE_OUTER_BOUND('',#5603,.T.);
#3461=FACE_OUTER_BOUND('',#5604,.T.);
#3462=FACE_OUTER_BOUND('',#5605,.T.);
#3463=FACE_OUTER_BOUND('',#5606,.T.);
#3464=FACE_OUTER_BOUND('',#5607,.T.);
#3465=FACE_OUTER_BOUND('',#5608,.T.);
#3466=FACE_OUTER_BOUND('',#5609,.T.);
#3467=FACE_OUTER_BOUND('',#5610,.T.);
#3468=FACE_OUTER_BOUND('',#5611,.T.);
#3469=FACE_OUTER_BOUND('',#5612,.T.);
#3470=FACE_OUTER_BOUND('',#5613,.T.);
#3471=FACE_OUTER_BOUND('',#5614,.T.);
#3472=FACE_OUTER_BOUND('',#5615,.T.);
#3473=FACE_OUTER_BOUND('',#5616,.T.);
#3474=FACE_OUTER_BOUND('',#5617,.T.);
#3475=FACE_OUTER_BOUND('',#5618,.T.);
#3476=FACE_OUTER_BOUND('',#5619,.T.);
#3477=FACE_OUTER_BOUND('',#5620,.T.);
#3478=FACE_OUTER_BOUND('',#5621,.T.);
#3479=FACE_OUTER_BOUND('',#5622,.T.);
#3480=FACE_OUTER_BOUND('',#5623,.T.);
#3481=FACE_OUTER_BOUND('',#5624,.T.);
#3482=FACE_OUTER_BOUND('',#5625,.T.);
#3483=FACE_OUTER_BOUND('',#5626,.T.);
#3484=FACE_OUTER_BOUND('',#5627,.T.);
#3485=FACE_OUTER_BOUND('',#5628,.T.);
#3486=FACE_OUTER_BOUND('',#5629,.T.);
#3487=FACE_OUTER_BOUND('',#5630,.T.);
#3488=FACE_OUTER_BOUND('',#5631,.T.);
#3489=FACE_OUTER_BOUND('',#5632,.T.);
#3490=FACE_OUTER_BOUND('',#5634,.T.);
#3491=FACE_OUTER_BOUND('',#5635,.T.);
#3492=FACE_OUTER_BOUND('',#5636,.T.);
#3493=FACE_OUTER_BOUND('',#5637,.T.);
#3494=FACE_OUTER_BOUND('',#5638,.T.);
#3495=FACE_OUTER_BOUND('',#5639,.T.);
#3496=FACE_OUTER_BOUND('',#5640,.T.);
#3497=FACE_OUTER_BOUND('',#5641,.T.);
#3498=FACE_OUTER_BOUND('',#5642,.T.);
#3499=FACE_OUTER_BOUND('',#5643,.T.);
#3500=FACE_OUTER_BOUND('',#5644,.T.);
#3501=FACE_OUTER_BOUND('',#5645,.T.);
#3502=FACE_OUTER_BOUND('',#5646,.T.);
#3503=FACE_OUTER_BOUND('',#5647,.T.);
#3504=FACE_OUTER_BOUND('',#5648,.T.);
#3505=FACE_OUTER_BOUND('',#5649,.T.);
#3506=FACE_OUTER_BOUND('',#5650,.T.);
#3507=FACE_OUTER_BOUND('',#5651,.T.);
#3508=FACE_OUTER_BOUND('',#5652,.T.);
#3509=FACE_OUTER_BOUND('',#5653,.T.);
#3510=FACE_OUTER_BOUND('',#5654,.T.);
#3511=FACE_OUTER_BOUND('',#5655,.T.);
#3512=FACE_OUTER_BOUND('',#5656,.T.);
#3513=FACE_OUTER_BOUND('',#5657,.T.);
#3514=FACE_OUTER_BOUND('',#5658,.T.);
#3515=FACE_OUTER_BOUND('',#5659,.T.);
#3516=FACE_OUTER_BOUND('',#5660,.T.);
#3517=FACE_OUTER_BOUND('',#5661,.T.);
#3518=FACE_OUTER_BOUND('',#5662,.T.);
#3519=FACE_OUTER_BOUND('',#5663,.T.);
#3520=FACE_OUTER_BOUND('',#5664,.T.);
#3521=FACE_OUTER_BOUND('',#5665,.T.);
#3522=FACE_OUTER_BOUND('',#5666,.T.);
#3523=FACE_OUTER_BOUND('',#5667,.T.);
#3524=FACE_OUTER_BOUND('',#5668,.T.);
#3525=FACE_OUTER_BOUND('',#5669,.T.);
#3526=FACE_OUTER_BOUND('',#5670,.T.);
#3527=FACE_OUTER_BOUND('',#5671,.T.);
#3528=FACE_OUTER_BOUND('',#5672,.T.);
#3529=FACE_OUTER_BOUND('',#5673,.T.);
#3530=FACE_OUTER_BOUND('',#5674,.T.);
#3531=FACE_OUTER_BOUND('',#5675,.T.);
#3532=FACE_OUTER_BOUND('',#5676,.T.);
#3533=FACE_OUTER_BOUND('',#5677,.T.);
#3534=FACE_OUTER_BOUND('',#5678,.T.);
#3535=FACE_OUTER_BOUND('',#5679,.T.);
#3536=FACE_OUTER_BOUND('',#5680,.T.);
#3537=FACE_OUTER_BOUND('',#5681,.T.);
#3538=FACE_OUTER_BOUND('',#5682,.T.);
#3539=FACE_OUTER_BOUND('',#5683,.T.);
#3540=FACE_OUTER_BOUND('',#5684,.T.);
#3541=FACE_OUTER_BOUND('',#5685,.T.);
#3542=FACE_OUTER_BOUND('',#5686,.T.);
#3543=FACE_OUTER_BOUND('',#5687,.T.);
#3544=FACE_OUTER_BOUND('',#5688,.T.);
#3545=FACE_OUTER_BOUND('',#5689,.T.);
#3546=FACE_OUTER_BOUND('',#5690,.T.);
#3547=FACE_OUTER_BOUND('',#5691,.T.);
#3548=FACE_OUTER_BOUND('',#5692,.T.);
#3549=FACE_OUTER_BOUND('',#5693,.T.);
#3550=FACE_OUTER_BOUND('',#5694,.T.);
#3551=FACE_OUTER_BOUND('',#5695,.T.);
#3552=FACE_OUTER_BOUND('',#5696,.T.);
#3553=FACE_OUTER_BOUND('',#5697,.T.);
#3554=FACE_OUTER_BOUND('',#5698,.T.);
#3555=FACE_OUTER_BOUND('',#5699,.T.);
#3556=FACE_OUTER_BOUND('',#5700,.T.);
#3557=FACE_OUTER_BOUND('',#5701,.T.);
#3558=FACE_OUTER_BOUND('',#5702,.T.);
#3559=FACE_OUTER_BOUND('',#5703,.T.);
#3560=FACE_OUTER_BOUND('',#5704,.T.);
#3561=FACE_OUTER_BOUND('',#5705,.T.);
#3562=FACE_OUTER_BOUND('',#5706,.T.);
#3563=FACE_OUTER_BOUND('',#5707,.T.);
#3564=FACE_OUTER_BOUND('',#5708,.T.);
#3565=FACE_OUTER_BOUND('',#5709,.T.);
#3566=FACE_OUTER_BOUND('',#5710,.T.);
#3567=FACE_OUTER_BOUND('',#5714,.T.);
#3568=FACE_OUTER_BOUND('',#5715,.T.);
#3569=FACE_OUTER_BOUND('',#5716,.T.);
#3570=FACE_OUTER_BOUND('',#5717,.T.);
#3571=FACE_OUTER_BOUND('',#5718,.T.);
#3572=FACE_OUTER_BOUND('',#5719,.T.);
#3573=FACE_OUTER_BOUND('',#5720,.T.);
#3574=FACE_OUTER_BOUND('',#5721,.T.);
#5424=EDGE_LOOP('',(#21801,#21802,#21803,#21804));
#5425=EDGE_LOOP('',(#21805,#21806,#21807,#21808,#21809,#21810,#21811,#21812,
#21813,#21814,#21815,#21816,#21817,#21818,#21819,#21820,#21821,#21822,#21823,
#21824,#21825,#21826,#21827,#21828,#21829,#21830,#21831,#21832,#21833,#21834,
#21835,#21836,#21837,#21838,#21839,#21840,#21841,#21842,#21843,#21844));
#5426=EDGE_LOOP('',(#21845,#21846,#21847,#21848,#21849,#21850,#21851,#21852,
#21853,#21854));
#5427=EDGE_LOOP('',(#21855,#21856,#21857,#21858,#21859,#21860,#21861,#21862,
#21863));
#5428=EDGE_LOOP('',(#21864,#21865,#21866,#21867,#21868,#21869,#21870,#21871,
#21872,#21873));
#5429=EDGE_LOOP('',(#21874,#21875,#21876,#21877,#21878));
#5430=EDGE_LOOP('',(#21879,#21880,#21881));
#5431=EDGE_LOOP('',(#21882,#21883,#21884,#21885));
#5432=EDGE_LOOP('',(#21886,#21887,#21888,#21889));
#5433=EDGE_LOOP('',(#21890,#21891,#21892,#21893,#21894));
#5434=EDGE_LOOP('',(#21895,#21896,#21897,#21898));
#5435=EDGE_LOOP('',(#21899,#21900,#21901,#21902,#21903,#21904));
#5436=EDGE_LOOP('',(#21905,#21906,#21907,#21908,#21909,#21910,#21911));
#5437=EDGE_LOOP('',(#21912,#21913,#21914,#21915,#21916));
#5438=EDGE_LOOP('',(#21917,#21918,#21919,#21920,#21921,#21922,#21923));
#5439=EDGE_LOOP('',(#21924,#21925,#21926,#21927,#21928));
#5440=EDGE_LOOP('',(#21929,#21930,#21931,#21932,#21933));
#5441=EDGE_LOOP('',(#21934,#21935,#21936,#21937,#21938,#21939));
#5442=EDGE_LOOP('',(#21940,#21941,#21942,#21943,#21944));
#5443=EDGE_LOOP('',(#21945,#21946,#21947,#21948));
#5444=EDGE_LOOP('',(#21949,#21950,#21951,#21952,#21953,#21954));
#5445=EDGE_LOOP('',(#21955,#21956,#21957,#21958,#21959));
#5446=EDGE_LOOP('',(#21960,#21961,#21962,#21963,#21964));
#5447=EDGE_LOOP('',(#21965,#21966,#21967,#21968,#21969,#21970,#21971));
#5448=EDGE_LOOP('',(#21972,#21973,#21974,#21975,#21976));
#5449=EDGE_LOOP('',(#21977,#21978,#21979,#21980,#21981,#21982,#21983));
#5450=EDGE_LOOP('',(#21984,#21985,#21986,#21987,#21988,#21989));
#5451=EDGE_LOOP('',(#21990,#21991,#21992,#21993));
#5452=EDGE_LOOP('',(#21994,#21995,#21996,#21997));
#5453=EDGE_LOOP('',(#21998,#21999,#22000,#22001));
#5454=EDGE_LOOP('',(#22002,#22003,#22004,#22005));
#5455=EDGE_LOOP('',(#22006,#22007,#22008,#22009));
#5456=EDGE_LOOP('',(#22010,#22011,#22012,#22013));
#5457=EDGE_LOOP('',(#22014,#22015,#22016,#22017));
#5458=EDGE_LOOP('',(#22018,#22019,#22020,#22021));
#5459=EDGE_LOOP('',(#22022,#22023,#22024,#22025));
#5460=EDGE_LOOP('',(#22026,#22027,#22028,#22029));
#5461=EDGE_LOOP('',(#22030,#22031,#22032,#22033));
#5462=EDGE_LOOP('',(#22034,#22035,#22036,#22037));
#5463=EDGE_LOOP('',(#22038,#22039,#22040,#22041));
#5464=EDGE_LOOP('',(#22042,#22043,#22044,#22045));
#5465=EDGE_LOOP('',(#22046,#22047,#22048,#22049));
#5466=EDGE_LOOP('',(#22050,#22051,#22052,#22053));
#5467=EDGE_LOOP('',(#22054,#22055,#22056,#22057));
#5468=EDGE_LOOP('',(#22058,#22059,#22060,#22061));
#5469=EDGE_LOOP('',(#22062,#22063,#22064,#22065));
#5470=EDGE_LOOP('',(#22066,#22067,#22068,#22069));
#5471=EDGE_LOOP('',(#22070,#22071,#22072,#22073));
#5472=EDGE_LOOP('',(#22074,#22075,#22076,#22077));
#5473=EDGE_LOOP('',(#22078,#22079,#22080,#22081));
#5474=EDGE_LOOP('',(#22082,#22083,#22084,#22085));
#5475=EDGE_LOOP('',(#22086,#22087,#22088,#22089));
#5476=EDGE_LOOP('',(#22090,#22091,#22092,#22093));
#5477=EDGE_LOOP('',(#22094,#22095,#22096,#22097));
#5478=EDGE_LOOP('',(#22098,#22099,#22100,#22101));
#5479=EDGE_LOOP('',(#22102,#22103,#22104,#22105));
#5480=EDGE_LOOP('',(#22106,#22107,#22108,#22109));
#5481=EDGE_LOOP('',(#22110,#22111,#22112,#22113));
#5482=EDGE_LOOP('',(#22114,#22115,#22116,#22117));
#5483=EDGE_LOOP('',(#22118,#22119,#22120,#22121));
#5484=EDGE_LOOP('',(#22122,#22123,#22124,#22125));
#5485=EDGE_LOOP('',(#22126,#22127,#22128,#22129));
#5486=EDGE_LOOP('',(#22130,#22131,#22132,#22133));
#5487=EDGE_LOOP('',(#22134,#22135,#22136,#22137));
#5488=EDGE_LOOP('',(#22138,#22139,#22140,#22141));
#5489=EDGE_LOOP('',(#22142,#22143,#22144,#22145));
#5490=EDGE_LOOP('',(#22146,#22147,#22148,#22149));
#5491=EDGE_LOOP('',(#22150,#22151,#22152,#22153));
#5492=EDGE_LOOP('',(#22154,#22155,#22156,#22157));
#5493=EDGE_LOOP('',(#22158,#22159,#22160,#22161));
#5494=EDGE_LOOP('',(#22162,#22163,#22164,#22165));
#5495=EDGE_LOOP('',(#22166,#22167,#22168,#22169));
#5496=EDGE_LOOP('',(#22170,#22171,#22172,#22173));
#5497=EDGE_LOOP('',(#22174,#22175,#22176,#22177));
#5498=EDGE_LOOP('',(#22178,#22179,#22180,#22181));
#5499=EDGE_LOOP('',(#22182,#22183,#22184,#22185));
#5500=EDGE_LOOP('',(#22186,#22187,#22188,#22189));
#5501=EDGE_LOOP('',(#22190,#22191,#22192,#22193));
#5502=EDGE_LOOP('',(#22194,#22195,#22196,#22197));
#5503=EDGE_LOOP('',(#22198,#22199,#22200,#22201));
#5504=EDGE_LOOP('',(#22202,#22203,#22204,#22205));
#5505=EDGE_LOOP('',(#22206,#22207,#22208,#22209));
#5506=EDGE_LOOP('',(#22210,#22211,#22212,#22213));
#5507=EDGE_LOOP('',(#22214,#22215,#22216,#22217));
#5508=EDGE_LOOP('',(#22218,#22219,#22220,#22221));
#5509=EDGE_LOOP('',(#22222,#22223,#22224,#22225));
#5510=EDGE_LOOP('',(#22226,#22227,#22228,#22229));
#5511=EDGE_LOOP('',(#22230,#22231,#22232,#22233));
#5512=EDGE_LOOP('',(#22234,#22235,#22236,#22237));
#5513=EDGE_LOOP('',(#22238,#22239,#22240,#22241));
#5514=EDGE_LOOP('',(#22242,#22243,#22244,#22245));
#5515=EDGE_LOOP('',(#22246,#22247,#22248,#22249));
#5516=EDGE_LOOP('',(#22250,#22251,#22252,#22253));
#5517=EDGE_LOOP('',(#22254,#22255,#22256,#22257));
#5518=EDGE_LOOP('',(#22258,#22259,#22260,#22261));
#5519=EDGE_LOOP('',(#22262,#22263,#22264,#22265));
#5520=EDGE_LOOP('',(#22266,#22267,#22268,#22269));
#5521=EDGE_LOOP('',(#22270,#22271,#22272,#22273));
#5522=EDGE_LOOP('',(#22274,#22275,#22276,#22277));
#5523=EDGE_LOOP('',(#22278,#22279,#22280,#22281));
#5524=EDGE_LOOP('',(#22282,#22283,#22284,#22285));
#5525=EDGE_LOOP('',(#22286,#22287,#22288,#22289));
#5526=EDGE_LOOP('',(#22290,#22291,#22292,#22293));
#5527=EDGE_LOOP('',(#22294,#22295,#22296,#22297));
#5528=EDGE_LOOP('',(#22298,#22299,#22300,#22301));
#5529=EDGE_LOOP('',(#22302,#22303,#22304,#22305));
#5530=EDGE_LOOP('',(#22306,#22307,#22308,#22309));
#5531=EDGE_LOOP('',(#22310,#22311,#22312,#22313));
#5532=EDGE_LOOP('',(#22314,#22315,#22316,#22317));
#5533=EDGE_LOOP('',(#22318,#22319,#22320,#22321));
#5534=EDGE_LOOP('',(#22322,#22323,#22324,#22325,#22326));
#5535=EDGE_LOOP('',(#22327,#22328,#22329,#22330,#22331));
#5536=EDGE_LOOP('',(#22332,#22333,#22334,#22335));
#5537=EDGE_LOOP('',(#22336,#22337,#22338,#22339));
#5538=EDGE_LOOP('',(#22340,#22341,#22342,#22343));
#5539=EDGE_LOOP('',(#22344,#22345,#22346,#22347));
#5540=EDGE_LOOP('',(#22348,#22349,#22350,#22351));
#5541=EDGE_LOOP('',(#22352,#22353,#22354,#22355,#22356));
#5542=EDGE_LOOP('',(#22357,#22358,#22359,#22360));
#5543=EDGE_LOOP('',(#22361,#22362,#22363,#22364));
#5544=EDGE_LOOP('',(#22365,#22366,#22367,#22368));
#5545=EDGE_LOOP('',(#22369,#22370,#22371,#22372));
#5546=EDGE_LOOP('',(#22373,#22374,#22375,#22376));
#5547=EDGE_LOOP('',(#22377,#22378,#22379,#22380));
#5548=EDGE_LOOP('',(#22381,#22382,#22383,#22384));
#5549=EDGE_LOOP('',(#22385,#22386,#22387,#22388));
#5550=EDGE_LOOP('',(#22389,#22390,#22391,#22392));
#5551=EDGE_LOOP('',(#22393,#22394,#22395,#22396));
#5552=EDGE_LOOP('',(#22397,#22398,#22399,#22400));
#5553=EDGE_LOOP('',(#22401,#22402,#22403,#22404));
#5554=EDGE_LOOP('',(#22405,#22406,#22407,#22408));
#5555=EDGE_LOOP('',(#22409,#22410,#22411,#22412));
#5556=EDGE_LOOP('',(#22413,#22414,#22415,#22416));
#5557=EDGE_LOOP('',(#22417,#22418,#22419,#22420));
#5558=EDGE_LOOP('',(#22421,#22422,#22423,#22424));
#5559=EDGE_LOOP('',(#22425,#22426,#22427,#22428));
#5560=EDGE_LOOP('',(#22429,#22430,#22431,#22432));
#5561=EDGE_LOOP('',(#22433,#22434,#22435,#22436,#22437,#22438));
#5562=EDGE_LOOP('',(#22439,#22440,#22441));
#5563=EDGE_LOOP('',(#22442,#22443,#22444,#22445,#22446,#22447));
#5564=EDGE_LOOP('',(#22448,#22449,#22450));
#5565=EDGE_LOOP('',(#22451,#22452,#22453,#22454));
#5566=EDGE_LOOP('',(#22455,#22456,#22457,#22458));
#5567=EDGE_LOOP('',(#22459,#22460,#22461,#22462));
#5568=EDGE_LOOP('',(#22463,#22464,#22465,#22466));
#5569=EDGE_LOOP('',(#22467,#22468,#22469,#22470));
#5570=EDGE_LOOP('',(#22471,#22472,#22473,#22474));
#5571=EDGE_LOOP('',(#22475,#22476,#22477,#22478));
#5572=EDGE_LOOP('',(#22479,#22480,#22481,#22482));
#5573=EDGE_LOOP('',(#22483,#22484,#22485,#22486));
#5574=EDGE_LOOP('',(#22487,#22488,#22489));
#5575=EDGE_LOOP('',(#22490,#22491,#22492,#22493,#22494,#22495));
#5576=EDGE_LOOP('',(#22496,#22497,#22498,#22499,#22500,#22501));
#5577=EDGE_LOOP('',(#22502,#22503,#22504));
#5578=EDGE_LOOP('',(#22505,#22506,#22507,#22508));
#5579=EDGE_LOOP('',(#22509,#22510,#22511,#22512));
#5580=EDGE_LOOP('',(#22513,#22514,#22515,#22516));
#5581=EDGE_LOOP('',(#22517,#22518,#22519,#22520));
#5582=EDGE_LOOP('',(#22521,#22522,#22523,#22524));
#5583=EDGE_LOOP('',(#22525,#22526,#22527,#22528));
#5584=EDGE_LOOP('',(#22529,#22530,#22531,#22532));
#5585=EDGE_LOOP('',(#22533,#22534,#22535,#22536));
#5586=EDGE_LOOP('',(#22537,#22538,#22539,#22540));
#5587=EDGE_LOOP('',(#22541,#22542,#22543,#22544));
#5588=EDGE_LOOP('',(#22545,#22546,#22547,#22548));
#5589=EDGE_LOOP('',(#22549,#22550,#22551,#22552));
#5590=EDGE_LOOP('',(#22553,#22554,#22555,#22556));
#5591=EDGE_LOOP('',(#22557,#22558,#22559,#22560));
#5592=EDGE_LOOP('',(#22561,#22562,#22563,#22564));
#5593=EDGE_LOOP('',(#22565,#22566,#22567,#22568));
#5594=EDGE_LOOP('',(#22569,#22570,#22571,#22572));
#5595=EDGE_LOOP('',(#22573,#22574,#22575,#22576));
#5596=EDGE_LOOP('',(#22577,#22578,#22579,#22580));
#5597=EDGE_LOOP('',(#22581,#22582,#22583,#22584));
#5598=EDGE_LOOP('',(#22585,#22586,#22587,#22588));
#5599=EDGE_LOOP('',(#22589,#22590,#22591,#22592));
#5600=EDGE_LOOP('',(#22593,#22594,#22595,#22596));
#5601=EDGE_LOOP('',(#22597,#22598,#22599,#22600));
#5602=EDGE_LOOP('',(#22601,#22602,#22603,#22604));
#5603=EDGE_LOOP('',(#22605,#22606,#22607,#22608));
#5604=EDGE_LOOP('',(#22609,#22610,#22611,#22612));
#5605=EDGE_LOOP('',(#22613,#22614,#22615,#22616));
#5606=EDGE_LOOP('',(#22617,#22618,#22619,#22620));
#5607=EDGE_LOOP('',(#22621,#22622,#22623,#22624));
#5608=EDGE_LOOP('',(#22625,#22626,#22627,#22628));
#5609=EDGE_LOOP('',(#22629,#22630,#22631,#22632));
#5610=EDGE_LOOP('',(#22633,#22634,#22635,#22636));
#5611=EDGE_LOOP('',(#22637,#22638,#22639,#22640));
#5612=EDGE_LOOP('',(#22641,#22642,#22643,#22644));
#5613=EDGE_LOOP('',(#22645,#22646,#22647,#22648));
#5614=EDGE_LOOP('',(#22649,#22650,#22651,#22652));
#5615=EDGE_LOOP('',(#22653,#22654,#22655,#22656));
#5616=EDGE_LOOP('',(#22657,#22658,#22659,#22660));
#5617=EDGE_LOOP('',(#22661,#22662,#22663,#22664));
#5618=EDGE_LOOP('',(#22665,#22666,#22667,#22668));
#5619=EDGE_LOOP('',(#22669,#22670,#22671,#22672));
#5620=EDGE_LOOP('',(#22673,#22674,#22675,#22676));
#5621=EDGE_LOOP('',(#22677,#22678,#22679,#22680));
#5622=EDGE_LOOP('',(#22681,#22682,#22683,#22684));
#5623=EDGE_LOOP('',(#22685,#22686,#22687,#22688));
#5624=EDGE_LOOP('',(#22689,#22690,#22691,#22692));
#5625=EDGE_LOOP('',(#22693,#22694,#22695,#22696));
#5626=EDGE_LOOP('',(#22697,#22698,#22699,#22700));
#5627=EDGE_LOOP('',(#22701,#22702,#22703,#22704));
#5628=EDGE_LOOP('',(#22705,#22706,#22707,#22708));
#5629=EDGE_LOOP('',(#22709,#22710,#22711,#22712));
#5630=EDGE_LOOP('',(#22713,#22714,#22715,#22716));
#5631=EDGE_LOOP('',(#22717,#22718,#22719,#22720));
#5632=EDGE_LOOP('',(#22721,#22722,#22723,#22724,#22725,#22726,#22727,#22728,
#22729,#22730,#22731,#22732,#22733,#22734,#22735,#22736,#22737,#22738,#22739,
#22740,#22741,#22742,#22743,#22744,#22745,#22746,#22747,#22748,#22749,#22750,
#22751,#22752,#22753,#22754,#22755,#22756,#22757,#22758,#22759,#22760));
#5633=EDGE_LOOP('',(#22761,#22762,#22763,#22764,#22765,#22766,#22767,#22768,
#22769,#22770,#22771,#22772,#22773,#22774,#22775,#22776,#22777,#22778,#22779,
#22780,#22781,#22782,#22783));
#5634=EDGE_LOOP('',(#22784,#22785,#22786,#22787));
#5635=EDGE_LOOP('',(#22788,#22789,#22790,#22791));
#5636=EDGE_LOOP('',(#22792,#22793,#22794,#22795));
#5637=EDGE_LOOP('',(#22796,#22797,#22798,#22799));
#5638=EDGE_LOOP('',(#22800,#22801,#22802,#22803));
#5639=EDGE_LOOP('',(#22804,#22805,#22806,#22807));
#5640=EDGE_LOOP('',(#22808,#22809,#22810,#22811));
#5641=EDGE_LOOP('',(#22812,#22813,#22814,#22815));
#5642=EDGE_LOOP('',(#22816,#22817,#22818,#22819));
#5643=EDGE_LOOP('',(#22820,#22821,#22822,#22823));
#5644=EDGE_LOOP('',(#22824,#22825,#22826,#22827));
#5645=EDGE_LOOP('',(#22828,#22829,#22830,#22831));
#5646=EDGE_LOOP('',(#22832,#22833,#22834,#22835));
#5647=EDGE_LOOP('',(#22836,#22837,#22838,#22839));
#5648=EDGE_LOOP('',(#22840,#22841,#22842,#22843));
#5649=EDGE_LOOP('',(#22844,#22845,#22846,#22847));
#5650=EDGE_LOOP('',(#22848,#22849,#22850,#22851));
#5651=EDGE_LOOP('',(#22852,#22853,#22854,#22855));
#5652=EDGE_LOOP('',(#22856,#22857,#22858,#22859,#22860,#22861));
#5653=EDGE_LOOP('',(#22862,#22863,#22864,#22865));
#5654=EDGE_LOOP('',(#22866,#22867,#22868,#22869,#22870));
#5655=EDGE_LOOP('',(#22871,#22872,#22873,#22874,#22875));
#5656=EDGE_LOOP('',(#22876,#22877,#22878,#22879));
#5657=EDGE_LOOP('',(#22880,#22881,#22882,#22883));
#5658=EDGE_LOOP('',(#22884,#22885,#22886,#22887));
#5659=EDGE_LOOP('',(#22888,#22889,#22890,#22891,#22892));
#5660=EDGE_LOOP('',(#22893,#22894,#22895,#22896,#22897));
#5661=EDGE_LOOP('',(#22898,#22899,#22900,#22901));
#5662=EDGE_LOOP('',(#22902,#22903,#22904,#22905));
#5663=EDGE_LOOP('',(#22906,#22907,#22908,#22909));
#5664=EDGE_LOOP('',(#22910,#22911,#22912,#22913));
#5665=EDGE_LOOP('',(#22914,#22915,#22916,#22917,#22918,#22919));
#5666=EDGE_LOOP('',(#22920,#22921,#22922,#22923));
#5667=EDGE_LOOP('',(#22924,#22925,#22926,#22927));
#5668=EDGE_LOOP('',(#22928,#22929,#22930,#22931));
#5669=EDGE_LOOP('',(#22932,#22933,#22934,#22935));
#5670=EDGE_LOOP('',(#22936,#22937,#22938,#22939));
#5671=EDGE_LOOP('',(#22940,#22941,#22942,#22943,#22944,#22945,#22946));
#5672=EDGE_LOOP('',(#22947,#22948,#22949,#22950,#22951,#22952,#22953));
#5673=EDGE_LOOP('',(#22954,#22955,#22956,#22957));
#5674=EDGE_LOOP('',(#22958,#22959,#22960,#22961,#22962));
#5675=EDGE_LOOP('',(#22963,#22964,#22965,#22966,#22967));
#5676=EDGE_LOOP('',(#22968,#22969,#22970,#22971,#22972,#22973,#22974));
#5677=EDGE_LOOP('',(#22975,#22976,#22977,#22978,#22979));
#5678=EDGE_LOOP('',(#22980,#22981,#22982,#22983,#22984));
#5679=EDGE_LOOP('',(#22985,#22986,#22987,#22988));
#5680=EDGE_LOOP('',(#22989,#22990,#22991,#22992));
#5681=EDGE_LOOP('',(#22993,#22994,#22995,#22996));
#5682=EDGE_LOOP('',(#22997,#22998,#22999,#23000));
#5683=EDGE_LOOP('',(#23001,#23002,#23003,#23004));
#5684=EDGE_LOOP('',(#23005,#23006,#23007,#23008));
#5685=EDGE_LOOP('',(#23009,#23010,#23011,#23012));
#5686=EDGE_LOOP('',(#23013,#23014,#23015,#23016));
#5687=EDGE_LOOP('',(#23017,#23018,#23019,#23020));
#5688=EDGE_LOOP('',(#23021,#23022,#23023,#23024));
#5689=EDGE_LOOP('',(#23025,#23026,#23027,#23028));
#5690=EDGE_LOOP('',(#23029,#23030,#23031,#23032));
#5691=EDGE_LOOP('',(#23033,#23034,#23035));
#5692=EDGE_LOOP('',(#23036,#23037,#23038,#23039));
#5693=EDGE_LOOP('',(#23040,#23041,#23042,#23043));
#5694=EDGE_LOOP('',(#23044,#23045,#23046,#23047));
#5695=EDGE_LOOP('',(#23048,#23049,#23050,#23051));
#5696=EDGE_LOOP('',(#23052,#23053,#23054,#23055,#23056));
#5697=EDGE_LOOP('',(#23057,#23058,#23059,#23060,#23061));
#5698=EDGE_LOOP('',(#23062,#23063,#23064,#23065));
#5699=EDGE_LOOP('',(#23066,#23067,#23068,#23069));
#5700=EDGE_LOOP('',(#23070,#23071,#23072,#23073,#23074));
#5701=EDGE_LOOP('',(#23075,#23076,#23077,#23078,#23079));
#5702=EDGE_LOOP('',(#23080,#23081,#23082,#23083,#23084));
#5703=EDGE_LOOP('',(#23085,#23086,#23087,#23088));
#5704=EDGE_LOOP('',(#23089,#23090,#23091,#23092));
#5705=EDGE_LOOP('',(#23093,#23094,#23095,#23096,#23097));
#5706=EDGE_LOOP('',(#23098,#23099,#23100,#23101,#23102));
#5707=EDGE_LOOP('',(#23103,#23104,#23105,#23106,#23107));
#5708=EDGE_LOOP('',(#23108,#23109,#23110,#23111));
#5709=EDGE_LOOP('',(#23112,#23113,#23114,#23115));
#5710=EDGE_LOOP('',(#23116,#23117,#23118,#23119,#23120,#23121,#23122));
#5711=EDGE_LOOP('',(#23123,#23124,#23125,#23126,#23127,#23128,#23129,#23130,
#23131,#23132,#23133,#23134,#23135,#23136));
#5712=EDGE_LOOP('',(#23137,#23138,#23139,#23140,#23141,#23142,#23143,#23144,
#23145,#23146,#23147,#23148,#23149,#23150));
#5713=EDGE_LOOP('',(#23151,#23152,#23153,#23154,#23155,#23156,#23157,#23158,
#23159,#23160,#23161,#23162,#23163,#23164));
#5714=EDGE_LOOP('',(#23165,#23166,#23167,#23168));
#5715=EDGE_LOOP('',(#23169,#23170,#23171,#23172));
#5716=EDGE_LOOP('',(#23173,#23174,#23175,#23176));
#5717=EDGE_LOOP('',(#23177,#23178,#23179,#23180));
#5718=EDGE_LOOP('',(#23181,#23182,#23183,#23184));
#5719=EDGE_LOOP('',(#23185,#23186,#23187,#23188));
#5720=EDGE_LOOP('',(#23189,#23190,#23191,#23192));
#5721=EDGE_LOOP('',(#23193,#23194,#23195,#23196,#23197,#23198,#23199,#23200,
#23201,#23202,#23203,#23204,#23205,#23206,#23207,#23208,#23209,#23210,#23211,
#23212,#23213,#23214,#23215));
#5722=EDGE_LOOP('',(#23216,#23217,#23218,#23219,#23220,#23221,#23222));
#7640=LINE('',#49134,#9480);
#7641=LINE('',#49138,#9481);
#7642=LINE('',#49143,#9482);
#7643=LINE('',#49151,#9483);
#7644=LINE('',#49155,#9484);
#7645=LINE('',#49159,#9485);
#7646=LINE('',#49167,#9486);
#7647=LINE('',#49171,#9487);
#7648=LINE('',#49175,#9488);
#7649=LINE('',#49183,#9489);
#7650=LINE('',#49191,#9490);
#7651=LINE('',#49195,#9491);
#7652=LINE('',#49199,#9492);
#7653=LINE('',#49207,#9493);
#7654=LINE('',#49211,#9494);
#7655=LINE('',#49215,#9495);
#7656=LINE('',#49273,#9496);
#7657=LINE('',#49291,#9497);
#7658=LINE('',#49298,#9498);
#7659=LINE('',#49301,#9499);
#7660=LINE('',#49386,#9500);
#7661=LINE('',#49398,#9501);
#7662=LINE('',#49460,#9502);
#7663=LINE('',#49462,#9503);
#7664=LINE('',#49464,#9504);
#7665=LINE('',#49465,#9505);
#7666=LINE('',#49485,#9506);
#7667=LINE('',#49521,#9507);
#7668=LINE('',#49524,#9508);
#7669=LINE('',#49538,#9509);
#7670=LINE('',#49539,#9510);
#7671=LINE('',#49542,#9511);
#7672=LINE('',#49624,#9512);
#7673=LINE('',#49759,#9513);
#7674=LINE('',#49822,#9514);
#7675=LINE('',#49886,#9515);
#7676=LINE('',#49951,#9516);
#7677=LINE('',#50022,#9517);
#7678=LINE('',#50066,#9518);
#7679=LINE('',#50086,#9519);
#7680=LINE('',#50120,#9520);
#7681=LINE('',#50184,#9521);
#7682=LINE('',#50294,#9522);
#7683=LINE('',#50371,#9523);
#7684=LINE('',#50568,#9524);
#7685=LINE('',#50637,#9525);
#7686=LINE('',#50875,#9526);
#7687=LINE('',#50921,#9527);
#7688=LINE('',#50927,#9528);
#7689=LINE('',#50930,#9529);
#7690=LINE('',#50940,#9530);
#7691=LINE('',#50945,#9531);
#7692=LINE('',#50948,#9532);
#7693=LINE('',#50949,#9533);
#7694=LINE('',#50956,#9534);
#7695=LINE('',#50961,#9535);
#7696=LINE('',#50964,#9536);
#7697=LINE('',#50965,#9537);
#7698=LINE('',#50972,#9538);
#7699=LINE('',#50977,#9539);
#7700=LINE('',#50980,#9540);
#7701=LINE('',#50981,#9541);
#7702=LINE('',#50988,#9542);
#7703=LINE('',#50996,#9543);
#7704=LINE('',#51004,#9544);
#7705=LINE('',#51009,#9545);
#7706=LINE('',#51012,#9546);
#7707=LINE('',#51013,#9547);
#7708=LINE('',#51020,#9548);
#7709=LINE('',#51028,#9549);
#7710=LINE('',#51036,#9550);
#7711=LINE('',#51041,#9551);
#7712=LINE('',#51044,#9552);
#7713=LINE('',#51045,#9553);
#7714=LINE('',#51052,#9554);
#7715=LINE('',#51057,#9555);
#7716=LINE('',#51060,#9556);
#7717=LINE('',#51061,#9557);
#7718=LINE('',#51068,#9558);
#7719=LINE('',#51073,#9559);
#7720=LINE('',#51076,#9560);
#7721=LINE('',#51077,#9561);
#7722=LINE('',#51084,#9562);
#7723=LINE('',#51091,#9563);
#7724=LINE('',#51100,#9564);
#7725=LINE('',#51105,#9565);
#7726=LINE('',#51108,#9566);
#7727=LINE('',#51109,#9567);
#7728=LINE('',#51116,#9568);
#7729=LINE('',#51121,#9569);
#7730=LINE('',#51124,#9570);
#7731=LINE('',#51125,#9571);
#7732=LINE('',#51132,#9572);
#7733=LINE('',#51137,#9573);
#7734=LINE('',#51140,#9574);
#7735=LINE('',#51141,#9575);
#7736=LINE('',#51148,#9576);
#7737=LINE('',#51156,#9577);
#7738=LINE('',#51164,#9578);
#7739=LINE('',#51169,#9579);
#7740=LINE('',#51172,#9580);
#7741=LINE('',#51173,#9581);
#7742=LINE('',#51180,#9582);
#7743=LINE('',#51188,#9583);
#7744=LINE('',#51196,#9584);
#7745=LINE('',#51201,#9585);
#7746=LINE('',#51204,#9586);
#7747=LINE('',#51205,#9587);
#7748=LINE('',#51212,#9588);
#7749=LINE('',#51217,#9589);
#7750=LINE('',#51220,#9590);
#7751=LINE('',#51221,#9591);
#7752=LINE('',#51229,#9592);
#7753=LINE('',#51236,#9593);
#7754=LINE('',#51239,#9594);
#7755=LINE('',#51241,#9595);
#7756=LINE('',#51245,#9596);
#7757=LINE('',#51247,#9597);
#7758=LINE('',#51249,#9598);
#7759=LINE('',#51250,#9599);
#7760=LINE('',#51265,#9600);
#7761=LINE('',#51278,#9601);
#7762=LINE('',#51331,#9602);
#7763=LINE('',#51332,#9603);
#7764=LINE('',#51335,#9604);
#7765=LINE('',#51356,#9605);
#7766=LINE('',#51458,#9606);
#7767=LINE('',#51528,#9607);
#7768=LINE('',#51532,#9608);
#7769=LINE('',#51596,#9609);
#7770=LINE('',#51666,#9610);
#7771=LINE('',#51693,#9611);
#7772=LINE('',#51820,#9612);
#7773=LINE('',#51821,#9613);
#7774=LINE('',#51822,#9614);
#7775=LINE('',#51825,#9615);
#7776=LINE('',#51827,#9616);
#7777=LINE('',#51828,#9617);
#7778=LINE('',#52044,#9618);
#7779=LINE('',#53277,#9619);
#7780=LINE('',#53285,#9620);
#7781=LINE('',#53459,#9621);
#7782=LINE('',#54081,#9622);
#7783=LINE('',#54817,#9623);
#7784=LINE('',#54825,#9624);
#7785=LINE('',#54833,#9625);
#7786=LINE('',#54849,#9626);
#7787=LINE('',#54865,#9627);
#7788=LINE('',#54873,#9628);
#7789=LINE('',#54881,#9629);
#7790=LINE('',#54897,#9630);
#7791=LINE('',#54905,#9631);
#7792=LINE('',#54913,#9632);
#7793=LINE('',#54929,#9633);
#7794=LINE('',#54945,#9634);
#7795=LINE('',#54953,#9635);
#7796=LINE('',#54963,#9636);
#7797=LINE('',#54966,#9637);
#7798=LINE('',#54970,#9638);
#7799=LINE('',#54974,#9639);
#7800=LINE('',#54978,#9640);
#7801=LINE('',#54982,#9641);
#7802=LINE('',#54987,#9642);
#7803=LINE('',#54991,#9643);
#7804=LINE('',#54995,#9644);
#7805=LINE('',#54999,#9645);
#7806=LINE('',#55003,#9646);
#7807=LINE('',#55005,#9647);
#7808=LINE('',#55009,#9648);
#7809=LINE('',#55010,#9649);
#7810=LINE('',#55013,#9650);
#7811=LINE('',#55014,#9651);
#7812=LINE('',#55018,#9652);
#7813=LINE('',#55021,#9653);
#7814=LINE('',#55022,#9654);
#7815=LINE('',#55027,#9655);
#7816=LINE('',#55029,#9656);
#7817=LINE('',#55030,#9657);
#7818=LINE('',#55036,#9658);
#7819=LINE('',#55039,#9659);
#7820=LINE('',#55040,#9660);
#7821=LINE('',#55044,#9661);
#7822=LINE('',#55047,#9662);
#7823=LINE('',#55048,#9663);
#7824=LINE('',#55052,#9664);
#7825=LINE('',#55055,#9665);
#7826=LINE('',#55056,#9666);
#7827=LINE('',#55060,#9667);
#7828=LINE('',#55063,#9668);
#7829=LINE('',#55064,#9669);
#7830=LINE('',#55068,#9670);
#7831=LINE('',#55070,#9671);
#7832=LINE('',#55084,#9672);
#7833=LINE('',#55108,#9673);
#7834=LINE('',#55122,#9674);
#7835=LINE('',#55135,#9675);
#7836=LINE('',#55136,#9676);
#7837=LINE('',#55150,#9677);
#7838=LINE('',#55158,#9678);
#7839=LINE('',#55206,#9679);
#7840=LINE('',#55284,#9680);
#7841=LINE('',#55310,#9681);
#7842=LINE('',#55364,#9682);
#7843=LINE('',#55409,#9683);
#7844=LINE('',#55552,#9684);
#7845=LINE('',#56067,#9685);
#7846=LINE('',#56157,#9686);
#7847=LINE('',#56161,#9687);
#7848=LINE('',#56188,#9688);
#7849=LINE('',#56221,#9689);
#7850=LINE('',#56329,#9690);
#7851=LINE('',#56362,#9691);
#7852=LINE('',#57611,#9692);
#7853=LINE('',#57667,#9693);
#7854=LINE('',#57687,#9694);
#7855=LINE('',#57702,#9695);
#7856=LINE('',#57717,#9696);
#7857=LINE('',#57732,#9697);
#7858=LINE('',#57752,#9698);
#7859=LINE('',#57767,#9699);
#7860=LINE('',#57782,#9700);
#7861=LINE('',#57797,#9701);
#7862=LINE('',#57812,#9702);
#7863=LINE('',#57832,#9703);
#7864=LINE('',#57847,#9704);
#7865=LINE('',#57881,#9705);
#7866=LINE('',#57882,#9706);
#7867=LINE('',#57885,#9707);
#7868=LINE('',#57889,#9708);
#7869=LINE('',#57894,#9709);
#7870=LINE('',#57898,#9710);
#7871=LINE('',#57902,#9711);
#9480=VECTOR('',#38649,1000.);
#9481=VECTOR('',#38652,1000.);
#9482=VECTOR('',#38657,1000.);
#9483=VECTOR('',#38664,1000.);
#9484=VECTOR('',#38667,1000.);
#9485=VECTOR('',#38670,1000.);
#9486=VECTOR('',#38677,1000.);
#9487=VECTOR('',#38680,1000.);
#9488=VECTOR('',#38683,1000.);
#9489=VECTOR('',#38690,1000.);
#9490=VECTOR('',#38697,1000.);
#9491=VECTOR('',#38700,1000.);
#9492=VECTOR('',#38703,1000.);
#9493=VECTOR('',#38710,1000.);
#9494=VECTOR('',#38713,1000.);
#9495=VECTOR('',#38716,1000.);
#9496=VECTOR('',#38727,1000.);
#9497=VECTOR('',#38736,1000.);
#9498=VECTOR('',#38743,1000.);
#9499=VECTOR('',#38744,1000.);
#9500=VECTOR('',#38751,10.);
#9501=VECTOR('',#38752,10.);
#9502=VECTOR('',#38761,1000.);
#9503=VECTOR('',#38762,1000.);
#9504=VECTOR('',#38763,1000.);
#9505=VECTOR('',#38764,1000.);
#9506=VECTOR('',#38765,1000.);
#9507=VECTOR('',#38766,1000.);
#9508=VECTOR('',#38769,1000.);
#9509=VECTOR('',#38774,1000.);
#9510=VECTOR('',#38775,10.);
#9511=VECTOR('',#38778,1000.);
#9512=VECTOR('',#38783,1000.);
#9513=VECTOR('',#38788,1000.);
#9514=VECTOR('',#38789,1000.);
#9515=VECTOR('',#38792,1000.);
#9516=VECTOR('',#38793,1000.);
#9517=VECTOR('',#38800,1000.);
#9518=VECTOR('',#38803,1000.);
#9519=VECTOR('',#38804,1000.);
#9520=VECTOR('',#38807,1000.);
#9521=VECTOR('',#38810,1000.);
#9522=VECTOR('',#38811,1000.);
#9523=VECTOR('',#38812,1000.);
#9524=VECTOR('',#38815,1000.);
#9525=VECTOR('',#38816,1000.);
#9526=VECTOR('',#38823,1000.);
#9527=VECTOR('',#38830,10.);
#9528=VECTOR('',#38835,1000.);
#9529=VECTOR('',#38838,1000.);
#9530=VECTOR('',#38853,1000.);
#9531=VECTOR('',#38860,1000.);
#9532=VECTOR('',#38863,1000.);
#9533=VECTOR('',#38864,1000.);
#9534=VECTOR('',#38873,1000.);
#9535=VECTOR('',#38880,1000.);
#9536=VECTOR('',#38883,1000.);
#9537=VECTOR('',#38884,1000.);
#9538=VECTOR('',#38893,1000.);
#9539=VECTOR('',#38900,1000.);
#9540=VECTOR('',#38903,1000.);
#9541=VECTOR('',#38904,1000.);
#9542=VECTOR('',#38913,1000.);
#9543=VECTOR('',#38924,1000.);
#9544=VECTOR('',#38935,1000.);
#9545=VECTOR('',#38942,1000.);
#9546=VECTOR('',#38945,1000.);
#9547=VECTOR('',#38946,1000.);
#9548=VECTOR('',#38955,1000.);
#9549=VECTOR('',#38966,1000.);
#9550=VECTOR('',#38977,1000.);
#9551=VECTOR('',#38984,1000.);
#9552=VECTOR('',#38987,1000.);
#9553=VECTOR('',#38988,1000.);
#9554=VECTOR('',#38997,1000.);
#9555=VECTOR('',#39004,1000.);
#9556=VECTOR('',#39007,1000.);
#9557=VECTOR('',#39008,1000.);
#9558=VECTOR('',#39017,1000.);
#9559=VECTOR('',#39024,1000.);
#9560=VECTOR('',#39027,1000.);
#9561=VECTOR('',#39028,1000.);
#9562=VECTOR('',#39037,1000.);
#9563=VECTOR('',#39046,1000.);
#9564=VECTOR('',#39059,1000.);
#9565=VECTOR('',#39066,1000.);
#9566=VECTOR('',#39069,1000.);
#9567=VECTOR('',#39070,1000.);
#9568=VECTOR('',#39079,1000.);
#9569=VECTOR('',#39086,1000.);
#9570=VECTOR('',#39089,1000.);
#9571=VECTOR('',#39090,1000.);
#9572=VECTOR('',#39099,1000.);
#9573=VECTOR('',#39106,1000.);
#9574=VECTOR('',#39109,1000.);
#9575=VECTOR('',#39110,1000.);
#9576=VECTOR('',#39119,1000.);
#9577=VECTOR('',#39130,1000.);
#9578=VECTOR('',#39141,1000.);
#9579=VECTOR('',#39148,1000.);
#9580=VECTOR('',#39151,1000.);
#9581=VECTOR('',#39152,1000.);
#9582=VECTOR('',#39161,1000.);
#9583=VECTOR('',#39172,1000.);
#9584=VECTOR('',#39183,1000.);
#9585=VECTOR('',#39190,1000.);
#9586=VECTOR('',#39193,1000.);
#9587=VECTOR('',#39194,1000.);
#9588=VECTOR('',#39203,1000.);
#9589=VECTOR('',#39210,1000.);
#9590=VECTOR('',#39213,1000.);
#9591=VECTOR('',#39214,1000.);
#9592=VECTOR('',#39225,1000.);
#9593=VECTOR('',#39234,1000.);
#9594=VECTOR('',#39239,1000.);
#9595=VECTOR('',#39242,1000.);
#9596=VECTOR('',#39245,1000.);
#9597=VECTOR('',#39246,1000.);
#9598=VECTOR('',#39247,1000.);
#9599=VECTOR('',#39248,1000.);
#9600=VECTOR('',#39249,10.);
#9601=VECTOR('',#39250,10.);
#9602=VECTOR('',#39253,10.);
#9603=VECTOR('',#39254,10.);
#9604=VECTOR('',#39257,10.);
#9605=VECTOR('',#39258,10.);
#9606=VECTOR('',#39261,10.);
#9607=VECTOR('',#39262,10.);
#9608=VECTOR('',#39265,10.);
#9609=VECTOR('',#39266,10.);
#9610=VECTOR('',#39267,10.);
#9611=VECTOR('',#39268,10.);
#9612=VECTOR('',#39273,1000.);
#9613=VECTOR('',#39274,10.);
#9614=VECTOR('',#39275,1000.);
#9615=VECTOR('',#39278,1000.);
#9616=VECTOR('',#39279,10.);
#9617=VECTOR('',#39280,1000.);
#9618=VECTOR('',#39293,10.);
#9619=VECTOR('',#39324,10.);
#9620=VECTOR('',#39325,10.);
#9621=VECTOR('',#39328,10.);
#9622=VECTOR('',#39355,10.);
#9623=VECTOR('',#39404,1000.);
#9624=VECTOR('',#39415,1000.);
#9625=VECTOR('',#39426,1000.);
#9626=VECTOR('',#39449,1000.);
#9627=VECTOR('',#39472,1000.);
#9628=VECTOR('',#39483,1000.);
#9629=VECTOR('',#39494,1000.);
#9630=VECTOR('',#39517,1000.);
#9631=VECTOR('',#39528,1000.);
#9632=VECTOR('',#39539,1000.);
#9633=VECTOR('',#39562,1000.);
#9634=VECTOR('',#39585,1000.);
#9635=VECTOR('',#39596,1000.);
#9636=VECTOR('',#39611,1000.);
#9637=VECTOR('',#39614,1000.);
#9638=VECTOR('',#39617,1000.);
#9639=VECTOR('',#39620,1000.);
#9640=VECTOR('',#39623,1000.);
#9641=VECTOR('',#39626,1000.);
#9642=VECTOR('',#39631,1000.);
#9643=VECTOR('',#39634,1000.);
#9644=VECTOR('',#39637,1000.);
#9645=VECTOR('',#39640,1000.);
#9646=VECTOR('',#39645,1000.);
#9647=VECTOR('',#39646,1000.);
#9648=VECTOR('',#39651,10.);
#9649=VECTOR('',#39652,1000.);
#9650=VECTOR('',#39655,10.);
#9651=VECTOR('',#39656,1000.);
#9652=VECTOR('',#39661,1000.);
#9653=VECTOR('',#39664,10.);
#9654=VECTOR('',#39665,1000.);
#9655=VECTOR('',#39672,1000.);
#9656=VECTOR('',#39673,10.);
#9657=VECTOR('',#39674,1000.);
#9658=VECTOR('',#39683,1000.);
#9659=VECTOR('',#39686,10.);
#9660=VECTOR('',#39687,1000.);
#9661=VECTOR('',#39692,1000.);
#9662=VECTOR('',#39695,1000.);
#9663=VECTOR('',#39696,10.);
#9664=VECTOR('',#39701,1000.);
#9665=VECTOR('',#39704,1000.);
#9666=VECTOR('',#39705,10.);
#9667=VECTOR('',#39710,1000.);
#9668=VECTOR('',#39713,1000.);
#9669=VECTOR('',#39714,10.);
#9670=VECTOR('',#39719,1000.);
#9671=VECTOR('',#39722,10.);
#9672=VECTOR('',#39723,10.);
#9673=VECTOR('',#39724,10.);
#9674=VECTOR('',#39725,10.);
#9675=VECTOR('',#39728,10.);
#9676=VECTOR('',#39729,10.);
#9677=VECTOR('',#39730,10.);
#9678=VECTOR('',#39731,10.);
#9679=VECTOR('',#39732,10.);
#9680=VECTOR('',#39733,10.);
#9681=VECTOR('',#39734,10.);
#9682=VECTOR('',#39735,10.);
#9683=VECTOR('',#39736,10.);
#9684=VECTOR('',#39745,10.);
#9685=VECTOR('',#39756,1000.);
#9686=VECTOR('',#39761,1000.);
#9687=VECTOR('',#39766,1000.);
#9688=VECTOR('',#39771,1000.);
#9689=VECTOR('',#39776,1000.);
#9690=VECTOR('',#39783,1000.);
#9691=VECTOR('',#39788,1000.);
#9692=VECTOR('',#39831,10.);
#9693=VECTOR('',#39832,10.);
#9694=VECTOR('',#39833,10.);
#9695=VECTOR('',#39836,10.);
#9696=VECTOR('',#39839,10.);
#9697=VECTOR('',#39842,10.);
#9698=VECTOR('',#39843,10.);
#9699=VECTOR('',#39846,10.);
#9700=VECTOR('',#39849,10.);
#9701=VECTOR('',#39852,10.);
#9702=VECTOR('',#39855,10.);
#9703=VECTOR('',#39856,10.);
#9704=VECTOR('',#39859,10.);
#9705=VECTOR('',#39884,1000.);
#9706=VECTOR('',#39885,1000.);
#9707=VECTOR('',#39888,1000.);
#9708=VECTOR('',#39893,1000.);
#9709=VECTOR('',#39900,1000.);
#9710=VECTOR('',#39905,1000.);
#9711=VECTOR('',#39910,1000.);
#11323=CIRCLE('',#34305,0.299999999999997);
#11324=CIRCLE('',#34306,0.3);
#11325=CIRCLE('',#34308,0.399999999999999);
#11326=CIRCLE('',#34309,15.8);
#11327=CIRCLE('',#34310,0.200000000000001);
#11328=CIRCLE('',#34311,0.399999999999999);
#11329=CIRCLE('',#34312,0.399999999999999);
#11330=CIRCLE('',#34313,0.200000000000001);
#11331=CIRCLE('',#34314,15.8);
#11332=CIRCLE('',#34315,0.200000000000001);
#11333=CIRCLE('',#34316,0.399999999999999);
#11334=CIRCLE('',#34317,0.399999999999999);
#11335=CIRCLE('',#34318,0.200000000000001);
#11336=CIRCLE('',#34319,15.8);
#11337=CIRCLE('',#34320,0.399999999999999);
#11338=CIRCLE('',#34321,0.399999999999999);
#11339=CIRCLE('',#34322,15.8);
#11340=CIRCLE('',#34323,0.200000000000001);
#11341=CIRCLE('',#34324,0.399999999999999);
#11342=CIRCLE('',#34325,0.399999999999999);
#11343=CIRCLE('',#34326,0.200000000000001);
#11344=CIRCLE('',#34327,15.8);
#11345=CIRCLE('',#34328,0.200000000000001);
#11346=CIRCLE('',#34329,0.4);
#11347=CIRCLE('',#34330,0.399999999999999);
#11348=CIRCLE('',#34331,0.200000000000001);
#11349=CIRCLE('',#34332,15.8);
#11350=CIRCLE('',#34333,0.399999999999999);
#11351=CIRCLE('',#34334,0.3);
#11352=CIRCLE('',#34335,0.3);
#11353=CIRCLE('',#34336,0.3);
#11354=CIRCLE('',#34337,0.3);
#11355=CIRCLE('',#34338,3.89050581799);
#11356=CIRCLE('',#34339,0.3);
#11357=CIRCLE('',#34340,4.00389099741);
#11358=CIRCLE('',#34341,4.00389099741);
#11359=CIRCLE('',#34342,0.3);
#11360=CIRCLE('',#34343,0.3);
#11361=CIRCLE('',#34344,0.3);
#11362=CIRCLE('',#34345,0.3);
#11363=CIRCLE('',#34347,0.300011835782053);
#11364=CIRCLE('',#34348,0.300012859472308);
#11365=CIRCLE('',#34357,2.21359789376355);
#11366=CIRCLE('',#34366,2.21359789376338);
#11367=CIRCLE('',#34373,15.9);
#11368=CIRCLE('',#34374,15.9);
#11369=CIRCLE('',#34376,0.0999999999999996);
#11370=CIRCLE('',#34377,0.0999999999999996);
#11371=CIRCLE('',#34379,0.1);
#11372=CIRCLE('',#34380,0.3);
#11373=CIRCLE('',#34382,0.3);
#11374=CIRCLE('',#34384,0.1);
#11375=CIRCLE('',#34387,0.1);
#11376=CIRCLE('',#34388,0.3);
#11377=CIRCLE('',#34390,0.3);
#11378=CIRCLE('',#34392,0.1);
#11379=CIRCLE('',#34395,0.0999999999999997);
#11380=CIRCLE('',#34396,0.3);
#11381=CIRCLE('',#34398,0.3);
#11382=CIRCLE('',#34400,0.1);
#11383=CIRCLE('',#34403,0.0999999999999997);
#11384=CIRCLE('',#34404,0.3);
#11385=CIRCLE('',#34406,0.3);
#11386=CIRCLE('',#34408,0.1);
#11387=CIRCLE('',#34409,15.9);
#11388=CIRCLE('',#34411,15.9);
#11389=CIRCLE('',#34413,0.0999999999999994);
#11390=CIRCLE('',#34414,0.5);
#11391=CIRCLE('',#34416,0.5);
#11392=CIRCLE('',#34418,0.0999999999999994);
#11393=CIRCLE('',#34421,0.1);
#11394=CIRCLE('',#34422,0.5);
#11395=CIRCLE('',#34424,0.5);
#11396=CIRCLE('',#34426,0.0999999999999997);
#11397=CIRCLE('',#34427,15.9);
#11398=CIRCLE('',#34429,15.9);
#11399=CIRCLE('',#34431,0.1);
#11400=CIRCLE('',#34432,0.3);
#11401=CIRCLE('',#34434,0.3);
#11402=CIRCLE('',#34436,0.0999999999999997);
#11403=CIRCLE('',#34439,0.1);
#11404=CIRCLE('',#34440,0.3);
#11405=CIRCLE('',#34442,0.3);
#11406=CIRCLE('',#34444,0.1);
#11407=CIRCLE('',#34447,0.1);
#11408=CIRCLE('',#34448,0.3);
#11409=CIRCLE('',#34450,0.3);
#11410=CIRCLE('',#34452,0.1);
#11411=CIRCLE('',#34455,0.0999999999999996);
#11412=CIRCLE('',#34456,0.3);
#11413=CIRCLE('',#34458,0.3);
#11414=CIRCLE('',#34460,15.9);
#11415=CIRCLE('',#34461,15.9);
#11416=CIRCLE('',#34463,0.0999999999999996);
#11417=CIRCLE('',#34465,0.1);
#11418=CIRCLE('',#34466,0.3);
#11419=CIRCLE('',#34468,0.3);
#11420=CIRCLE('',#34470,0.1);
#11421=CIRCLE('',#34473,0.1);
#11422=CIRCLE('',#34474,0.3);
#11423=CIRCLE('',#34476,0.3);
#11424=CIRCLE('',#34478,0.1);
#11425=CIRCLE('',#34481,0.0999999999999997);
#11426=CIRCLE('',#34482,0.3);
#11427=CIRCLE('',#34484,0.3);
#11428=CIRCLE('',#34486,0.1);
#11429=CIRCLE('',#34489,0.0999999999999997);
#11430=CIRCLE('',#34490,0.3);
#11431=CIRCLE('',#34492,0.3);
#11432=CIRCLE('',#34494,0.1);
#11433=CIRCLE('',#34495,15.9);
#11434=CIRCLE('',#34497,15.9);
#11435=CIRCLE('',#34499,0.0999999999999994);
#11436=CIRCLE('',#34500,0.5);
#11437=CIRCLE('',#34502,0.5);
#11438=CIRCLE('',#34504,0.0999999999999994);
#11439=CIRCLE('',#34507,0.1);
#11440=CIRCLE('',#34508,0.5);
#11441=CIRCLE('',#34510,0.5);
#11442=CIRCLE('',#34512,0.100000000000001);
#11443=CIRCLE('',#34513,15.9);
#11444=CIRCLE('',#34515,15.9);
#11445=CIRCLE('',#34517,0.1);
#11446=CIRCLE('',#34518,0.3);
#11447=CIRCLE('',#34520,0.3);
#11448=CIRCLE('',#34522,0.0999999999999997);
#11449=CIRCLE('',#34525,0.1);
#11450=CIRCLE('',#34526,0.3);
#11451=CIRCLE('',#34528,0.3);
#11452=CIRCLE('',#34530,0.0999999999999997);
#11453=CIRCLE('',#34533,0.3);
#11454=CIRCLE('',#34534,0.1);
#11455=CIRCLE('',#34536,0.3);
#11456=CIRCLE('',#34538,0.1);
#11457=CIRCLE('',#34539,0.3);
#11458=CIRCLE('',#34541,0.3);
#11459=CIRCLE('',#34547,0.199628863365679);
#11460=CIRCLE('',#34548,25.8578696504043);
#11461=CIRCLE('',#34549,25.2720864994101);
#11462=CIRCLE('',#34552,1.00000028469603);
#11463=CIRCLE('',#34553,1.00000044523891);
#11464=CIRCLE('',#34554,1.00003251262321);
#11465=CIRCLE('',#34555,1.00000027785337);
#11466=CIRCLE('',#34557,1.00000151494447);
#11467=CIRCLE('',#34558,1.00000061628411);
#11468=CIRCLE('',#34559,0.199580166399456);
#11469=CIRCLE('',#34560,1.00000059230394);
#11470=CIRCLE('',#34561,1.00000225038159);
#11471=CIRCLE('',#34563,1.00000028769429);
#11472=CIRCLE('',#34564,1.00000056588799);
#11473=CIRCLE('',#34565,1.00094397097147);
#11474=CIRCLE('',#34566,1.00000104682485);
#11475=CIRCLE('',#34567,1.00000115828043);
#11476=CIRCLE('',#34568,1.0000112573725);
#11477=CIRCLE('',#34569,1.00001575325937);
#11478=CIRCLE('',#34570,1.0000246775636);
#11479=CIRCLE('',#34571,0.999999920339783);
#11480=CIRCLE('',#34572,1.00000014419189);
#11481=CIRCLE('',#34574,1.0000008808516);
#11482=CIRCLE('',#34576,1.00000035796375);
#11483=CIRCLE('',#34577,0.99999967643586);
#11484=CIRCLE('',#34578,1.00000028469559);
#11485=CIRCLE('',#34579,1.00000027785327);
#11486=CIRCLE('',#34580,1.0000022192481);
#11487=CIRCLE('',#34581,1.00000044523891);
#11488=CIRCLE('',#34582,1.00000088028536);
#11489=CIRCLE('',#34584,1.00000078095249);
#11490=CIRCLE('',#34585,1.00000035796383);
#11491=CIRCLE('',#34587,1.00000014499945);
#11492=CIRCLE('',#34588,1.00000027111426);
#11493=CIRCLE('',#34589,1.00002467755638);
#11494=CIRCLE('',#34590,1.00001261620148);
#11495=CIRCLE('',#34591,1.00001153699998);
#11496=CIRCLE('',#34592,1.00000072628758);
#11497=CIRCLE('',#34593,1.00000103074381);
#11498=CIRCLE('',#34594,1.00094348029171);
#11499=CIRCLE('',#34595,1.00000030121054);
#11500=CIRCLE('',#34596,1.00000056588799);
#11501=CIRCLE('',#34597,1.00000061628416);
#11502=CIRCLE('',#34598,1.00000151494756);
#11503=CIRCLE('',#34599,1.00000225038157);
#11504=CIRCLE('',#34600,1.00000062699678);
#11505=CIRCLE('',#34603,0.0999999999999996);
#11506=CIRCLE('',#34604,15.8);
#11507=CIRCLE('',#34605,0.0999999999999996);
#11508=CIRCLE('',#34607,0.1);
#11509=CIRCLE('',#34608,0.200000000000001);
#11510=CIRCLE('',#34610,0.1);
#11511=CIRCLE('',#34612,0.1);
#11512=CIRCLE('',#34613,0.399999999999999);
#11513=CIRCLE('',#34615,0.1);
#11514=CIRCLE('',#34617,0.0999999999999997);
#11515=CIRCLE('',#34618,0.399999999999999);
#11516=CIRCLE('',#34620,0.1);
#11517=CIRCLE('',#34622,0.0999999999999997);
#11518=CIRCLE('',#34623,0.200000000000001);
#11519=CIRCLE('',#34625,0.1);
#11520=CIRCLE('',#34626,15.8);
#11521=CIRCLE('',#34628,0.0999999999999994);
#11522=CIRCLE('',#34629,0.399999999999999);
#11523=CIRCLE('',#34631,0.0999999999999994);
#11524=CIRCLE('',#34633,0.1);
#11525=CIRCLE('',#34634,0.399999999999999);
#11526=CIRCLE('',#34636,0.0999999999999997);
#11527=CIRCLE('',#34637,15.8);
#11528=CIRCLE('',#34639,0.1);
#11529=CIRCLE('',#34640,0.200000000000001);
#11530=CIRCLE('',#34642,0.0999999999999994);
#11531=CIRCLE('',#34644,0.1);
#11532=CIRCLE('',#34645,0.399999999999999);
#11533=CIRCLE('',#34647,0.1);
#11534=CIRCLE('',#34649,0.1);
#11535=CIRCLE('',#34650,0.399999999999999);
#11536=CIRCLE('',#34652,0.1);
#11537=CIRCLE('',#34654,0.0999999999999996);
#11538=CIRCLE('',#34655,0.200000000000001);
#11539=CIRCLE('',#34657,0.0999999999999996);
#11540=CIRCLE('',#34658,15.8);
#11541=CIRCLE('',#34660,0.1);
#11542=CIRCLE('',#34661,0.200000000000001);
#11543=CIRCLE('',#34663,0.1);
#11544=CIRCLE('',#34665,0.1);
#11545=CIRCLE('',#34666,0.399999999999999);
#11546=CIRCLE('',#34668,0.1);
#11547=CIRCLE('',#34670,0.0999999999999997);
#11548=CIRCLE('',#34671,0.399999999999999);
#11549=CIRCLE('',#34673,0.1);
#11550=CIRCLE('',#34675,0.0999999999999997);
#11551=CIRCLE('',#34676,0.200000000000001);
#11552=CIRCLE('',#34678,0.1);
#11553=CIRCLE('',#34679,15.8);
#11554=CIRCLE('',#34681,0.0999999999999994);
#11555=CIRCLE('',#34682,0.399999999999999);
#11556=CIRCLE('',#34684,0.0999999999999994);
#11557=CIRCLE('',#34686,0.1);
#11558=CIRCLE('',#34687,0.399999999999999);
#11559=CIRCLE('',#34689,0.100000000000001);
#11560=CIRCLE('',#34690,15.8);
#11561=CIRCLE('',#34692,0.1);
#11562=CIRCLE('',#34693,0.200000000000001);
#11563=CIRCLE('',#34695,0.0999999999999997);
#11564=CIRCLE('',#34697,0.1);
#11565=CIRCLE('',#34698,0.399999999999999);
#11566=CIRCLE('',#34700,0.0999999999999994);
#11567=CIRCLE('',#34702,0.200000000000001);
#11568=CIRCLE('',#34703,0.1);
#11569=CIRCLE('',#34705,0.1);
#11570=CIRCLE('',#34706,0.4);
#11571=CIRCLE('',#34709,1.5);
#11572=CIRCLE('',#34710,1.5);
#11573=CIRCLE('',#34711,14.4);
#11574=CIRCLE('',#34712,1.5);
#11575=CIRCLE('',#34713,1.5);
#11576=CIRCLE('',#34714,1.5);
#11577=CIRCLE('',#34715,1.5);
#11578=CIRCLE('',#34716,14.4);
#11579=CIRCLE('',#34717,1.5);
#11580=CIRCLE('',#34718,1.5);
#11581=CIRCLE('',#34720,14.4);
#11582=CIRCLE('',#34724,1.5);
#11583=CIRCLE('',#34727,1.5);
#11584=CIRCLE('',#34730,1.5);
#11585=CIRCLE('',#34732,1.5);
#11586=CIRCLE('',#34735,14.4);
#11587=CIRCLE('',#34738,1.5);
#11588=CIRCLE('',#34741,1.5);
#11589=CIRCLE('',#34744,1.5);
#11590=CIRCLE('',#34747,25.2720864994101);
#11591=CIRCLE('',#34749,1.5);
#11592=CIRCLE('',#34750,25.8578696504043);
#11593=CIRCLE('',#34751,0.300021606146326);
#11594=CIRCLE('',#34752,0.300022261835106);
#11595=CIRCLE('',#34753,0.300005681511778);
#11596=CIRCLE('',#34759,0.300000000000001);
#11597=CIRCLE('',#34771,0.300006142570235);
#11598=CIRCLE('',#34775,0.300000544869244);
#11599=CIRCLE('',#34776,0.300000585046962);
#11600=CIRCLE('',#34777,0.300165537902904);
#11601=CIRCLE('',#34778,0.300000598082167);
#11602=CIRCLE('',#34779,0.300000584963546);
#11603=CIRCLE('',#34783,0.300006218981457);
#11604=CIRCLE('',#34784,0.3);
#11605=CIRCLE('',#34786,0.300012869270441);
#11606=CIRCLE('',#34787,0.300007072562979);
#11607=CIRCLE('',#34788,0.300022294497527);
#11608=CIRCLE('',#34789,0.300021607322509);
#11609=CIRCLE('',#34790,0.999998074024125);
#11610=CIRCLE('',#34791,24.7051161323679);
#11611=CIRCLE('',#34792,24.8400616948579);
#11612=CIRCLE('',#34794,24.7051633159733);
#11613=CIRCLE('',#34795,24.7051633159701);
#11614=CIRCLE('',#34797,24.8400616948579);
#11615=CIRCLE('',#34798,24.7051161323679);
#11616=CIRCLE('',#34799,0.999998074024125);
#11617=CIRCLE('',#34801,5.);
#11618=CIRCLE('',#34802,16.1875296363);
#11619=CIRCLE('',#34803,26.2647265892);
#11620=CIRCLE('',#34804,12.2773059952);
#11621=CIRCLE('',#34805,12.2773059952);
#11622=CIRCLE('',#34806,26.2647265892);
#11623=CIRCLE('',#34807,16.1875296363);
#11624=CIRCLE('',#34809,16.1875296363);
#11625=CIRCLE('',#34811,26.2647265891997);
#11626=CIRCLE('',#34813,12.2773059952);
#11627=CIRCLE('',#34815,12.2773059952);
#11628=CIRCLE('',#34817,26.2647265892);
#11629=CIRCLE('',#34819,16.1875296363);
#11630=CIRCLE('',#34821,4.99999999999993);
#13631=VERTEX_POINT('',#49132);
#13632=VERTEX_POINT('',#49133);
#13633=VERTEX_POINT('',#49135);
#13634=VERTEX_POINT('',#49137);
#13635=VERTEX_POINT('',#49141);
#13636=VERTEX_POINT('',#49142);
#13637=VERTEX_POINT('',#49144);
#13638=VERTEX_POINT('',#49146);
#13639=VERTEX_POINT('',#49148);
#13640=VERTEX_POINT('',#49150);
#13641=VERTEX_POINT('',#49152);
#13642=VERTEX_POINT('',#49154);
#13643=VERTEX_POINT('',#49156);
#13644=VERTEX_POINT('',#49158);
#13645=VERTEX_POINT('',#49160);
#13646=VERTEX_POINT('',#49162);
#13647=VERTEX_POINT('',#49164);
#13648=VERTEX_POINT('',#49166);
#13649=VERTEX_POINT('',#49168);
#13650=VERTEX_POINT('',#49170);
#13651=VERTEX_POINT('',#49172);
#13652=VERTEX_POINT('',#49174);
#13653=VERTEX_POINT('',#49176);
#13654=VERTEX_POINT('',#49178);
#13655=VERTEX_POINT('',#49180);
#13656=VERTEX_POINT('',#49182);
#13657=VERTEX_POINT('',#49184);
#13658=VERTEX_POINT('',#49186);
#13659=VERTEX_POINT('',#49188);
#13660=VERTEX_POINT('',#49190);
#13661=VERTEX_POINT('',#49192);
#13662=VERTEX_POINT('',#49194);
#13663=VERTEX_POINT('',#49196);
#13664=VERTEX_POINT('',#49198);
#13665=VERTEX_POINT('',#49200);
#13666=VERTEX_POINT('',#49202);
#13667=VERTEX_POINT('',#49204);
#13668=VERTEX_POINT('',#49206);
#13669=VERTEX_POINT('',#49208);
#13670=VERTEX_POINT('',#49210);
#13671=VERTEX_POINT('',#49212);
#13672=VERTEX_POINT('',#49214);
#13673=VERTEX_POINT('',#49216);
#13674=VERTEX_POINT('',#49218);
#13675=VERTEX_POINT('',#49221);
#13676=VERTEX_POINT('',#49222);
#13677=VERTEX_POINT('',#49224);
#13678=VERTEX_POINT('',#49232);
#13679=VERTEX_POINT('',#49239);
#13680=VERTEX_POINT('',#49251);
#13681=VERTEX_POINT('',#49258);
#13682=VERTEX_POINT('',#49270);
#13683=VERTEX_POINT('',#49272);
#13684=VERTEX_POINT('',#49274);
#13685=VERTEX_POINT('',#49284);
#13686=VERTEX_POINT('',#49285);
#13687=VERTEX_POINT('',#49287);
#13688=VERTEX_POINT('',#49289);
#13689=VERTEX_POINT('',#49292);
#13690=VERTEX_POINT('',#49294);
#13691=VERTEX_POINT('',#49296);
#13692=VERTEX_POINT('',#49299);
#13693=VERTEX_POINT('',#49300);
#13694=VERTEX_POINT('',#49302);
#13695=VERTEX_POINT('',#49304);
#13696=VERTEX_POINT('',#49323);
#13697=VERTEX_POINT('',#49330);
#13698=VERTEX_POINT('',#49346);
#13699=VERTEX_POINT('',#49353);
#13700=VERTEX_POINT('',#49358);
#13701=VERTEX_POINT('',#49360);
#13702=VERTEX_POINT('',#49384);
#13703=VERTEX_POINT('',#49385);
#13704=VERTEX_POINT('',#49387);
#13705=VERTEX_POINT('',#49397);
#13706=VERTEX_POINT('',#49399);
#13707=VERTEX_POINT('',#49454);
#13708=VERTEX_POINT('',#49458);
#13709=VERTEX_POINT('',#49459);
#13710=VERTEX_POINT('',#49461);
#13711=VERTEX_POINT('',#49463);
#13712=VERTEX_POINT('',#49484);
#13713=VERTEX_POINT('',#49486);
#13714=VERTEX_POINT('',#49523);
#13715=VERTEX_POINT('',#49525);
#13716=VERTEX_POINT('',#49537);
#13717=VERTEX_POINT('',#49541);
#13718=VERTEX_POINT('',#49543);
#13719=VERTEX_POINT('',#49545);
#13720=VERTEX_POINT('',#49623);
#13721=VERTEX_POINT('',#49625);
#13722=VERTEX_POINT('',#49669);
#13723=VERTEX_POINT('',#49671);
#13724=VERTEX_POINT('',#49758);
#13725=VERTEX_POINT('',#49760);
#13726=VERTEX_POINT('',#49821);
#13727=VERTEX_POINT('',#49823);
#13728=VERTEX_POINT('',#49830);
#13729=VERTEX_POINT('',#49843);
#13730=VERTEX_POINT('',#49885);
#13731=VERTEX_POINT('',#49887);
#13732=VERTEX_POINT('',#49950);
#13733=VERTEX_POINT('',#49952);
#13734=VERTEX_POINT('',#49976);
#13735=VERTEX_POINT('',#49978);
#13736=VERTEX_POINT('',#50021);
#13737=VERTEX_POINT('',#50023);
#13738=VERTEX_POINT('',#50025);
#13739=VERTEX_POINT('',#50085);
#13740=VERTEX_POINT('',#50119);
#13741=VERTEX_POINT('',#50121);
#13742=VERTEX_POINT('',#50126);
#13743=VERTEX_POINT('',#50183);
#13744=VERTEX_POINT('',#50185);
#13745=VERTEX_POINT('',#50293);
#13746=VERTEX_POINT('',#50295);
#13747=VERTEX_POINT('',#50370);
#13748=VERTEX_POINT('',#50372);
#13749=VERTEX_POINT('',#50374);
#13750=VERTEX_POINT('',#50403);
#13751=VERTEX_POINT('',#50567);
#13752=VERTEX_POINT('',#50569);
#13753=VERTEX_POINT('',#50636);
#13754=VERTEX_POINT('',#50638);
#13755=VERTEX_POINT('',#50640);
#13756=VERTEX_POINT('',#50783);
#13757=VERTEX_POINT('',#50874);
#13758=VERTEX_POINT('',#50876);
#13759=VERTEX_POINT('',#50878);
#13760=VERTEX_POINT('',#50923);
#13761=VERTEX_POINT('',#50924);
#13762=VERTEX_POINT('',#50926);
#13763=VERTEX_POINT('',#50928);
#13764=VERTEX_POINT('',#50935);
#13765=VERTEX_POINT('',#50939);
#13766=VERTEX_POINT('',#50943);
#13767=VERTEX_POINT('',#50947);
#13768=VERTEX_POINT('',#50951);
#13769=VERTEX_POINT('',#50955);
#13770=VERTEX_POINT('',#50959);
#13771=VERTEX_POINT('',#50963);
#13772=VERTEX_POINT('',#50967);
#13773=VERTEX_POINT('',#50971);
#13774=VERTEX_POINT('',#50975);
#13775=VERTEX_POINT('',#50979);
#13776=VERTEX_POINT('',#50983);
#13777=VERTEX_POINT('',#50987);
#13778=VERTEX_POINT('',#50991);
#13779=VERTEX_POINT('',#50995);
#13780=VERTEX_POINT('',#50999);
#13781=VERTEX_POINT('',#51003);
#13782=VERTEX_POINT('',#51007);
#13783=VERTEX_POINT('',#51011);
#13784=VERTEX_POINT('',#51015);
#13785=VERTEX_POINT('',#51019);
#13786=VERTEX_POINT('',#51023);
#13787=VERTEX_POINT('',#51027);
#13788=VERTEX_POINT('',#51031);
#13789=VERTEX_POINT('',#51035);
#13790=VERTEX_POINT('',#51039);
#13791=VERTEX_POINT('',#51043);
#13792=VERTEX_POINT('',#51047);
#13793=VERTEX_POINT('',#51051);
#13794=VERTEX_POINT('',#51055);
#13795=VERTEX_POINT('',#51059);
#13796=VERTEX_POINT('',#51063);
#13797=VERTEX_POINT('',#51067);
#13798=VERTEX_POINT('',#51071);
#13799=VERTEX_POINT('',#51075);
#13800=VERTEX_POINT('',#51079);
#13801=VERTEX_POINT('',#51083);
#13802=VERTEX_POINT('',#51087);
#13803=VERTEX_POINT('',#51089);
#13804=VERTEX_POINT('',#51095);
#13805=VERTEX_POINT('',#51099);
#13806=VERTEX_POINT('',#51103);
#13807=VERTEX_POINT('',#51107);
#13808=VERTEX_POINT('',#51111);
#13809=VERTEX_POINT('',#51115);
#13810=VERTEX_POINT('',#51119);
#13811=VERTEX_POINT('',#51123);
#13812=VERTEX_POINT('',#51127);
#13813=VERTEX_POINT('',#51131);
#13814=VERTEX_POINT('',#51135);
#13815=VERTEX_POINT('',#51139);
#13816=VERTEX_POINT('',#51143);
#13817=VERTEX_POINT('',#51147);
#13818=VERTEX_POINT('',#51151);
#13819=VERTEX_POINT('',#51155);
#13820=VERTEX_POINT('',#51159);
#13821=VERTEX_POINT('',#51163);
#13822=VERTEX_POINT('',#51167);
#13823=VERTEX_POINT('',#51171);
#13824=VERTEX_POINT('',#51175);
#13825=VERTEX_POINT('',#51179);
#13826=VERTEX_POINT('',#51183);
#13827=VERTEX_POINT('',#51187);
#13828=VERTEX_POINT('',#51191);
#13829=VERTEX_POINT('',#51195);
#13830=VERTEX_POINT('',#51199);
#13831=VERTEX_POINT('',#51203);
#13832=VERTEX_POINT('',#51207);
#13833=VERTEX_POINT('',#51211);
#13834=VERTEX_POINT('',#51215);
#13835=VERTEX_POINT('',#51219);
#13836=VERTEX_POINT('',#51223);
#13837=VERTEX_POINT('',#51227);
#13838=VERTEX_POINT('',#51231);
#13839=VERTEX_POINT('',#51235);
#13840=VERTEX_POINT('',#51243);
#13841=VERTEX_POINT('',#51244);
#13842=VERTEX_POINT('',#51246);
#13843=VERTEX_POINT('',#51248);
#13844=VERTEX_POINT('',#51263);
#13845=VERTEX_POINT('',#51264);
#13846=VERTEX_POINT('',#51266);
#13847=VERTEX_POINT('',#51277);
#13848=VERTEX_POINT('',#51329);
#13849=VERTEX_POINT('',#51330);
#13850=VERTEX_POINT('',#51333);
#13851=VERTEX_POINT('',#51348);
#13852=VERTEX_POINT('',#51355);
#13853=VERTEX_POINT('',#51357);
#13854=VERTEX_POINT('',#51392);
#13855=VERTEX_POINT('',#51457);
#13856=VERTEX_POINT('',#51526);
#13857=VERTEX_POINT('',#51527);
#13858=VERTEX_POINT('',#51529);
#13859=VERTEX_POINT('',#51531);
#13860=VERTEX_POINT('',#51594);
#13861=VERTEX_POINT('',#51595);
#13862=VERTEX_POINT('',#51597);
#13863=VERTEX_POINT('',#51665);
#13864=VERTEX_POINT('',#51691);
#13865=VERTEX_POINT('',#51692);
#13866=VERTEX_POINT('',#51760);
#13867=VERTEX_POINT('',#51818);
#13868=VERTEX_POINT('',#51819);
#13869=VERTEX_POINT('',#51824);
#13870=VERTEX_POINT('',#51826);
#13871=VERTEX_POINT('',#51865);
#13872=VERTEX_POINT('',#51867);
#13873=VERTEX_POINT('',#51954);
#13874=VERTEX_POINT('',#51956);
#13875=VERTEX_POINT('',#52042);
#13876=VERTEX_POINT('',#52081);
#13877=VERTEX_POINT('',#52083);
#13878=VERTEX_POINT('',#52140);
#13879=VERTEX_POINT('',#52288);
#13880=VERTEX_POINT('',#52290);
#13881=VERTEX_POINT('',#52479);
#13882=VERTEX_POINT('',#52560);
#13883=VERTEX_POINT('',#52726);
#13884=VERTEX_POINT('',#52792);
#13885=VERTEX_POINT('',#52942);
#13886=VERTEX_POINT('',#53005);
#13887=VERTEX_POINT('',#53098);
#13888=VERTEX_POINT('',#53236);
#13889=VERTEX_POINT('',#53276);
#13890=VERTEX_POINT('',#53278);
#13891=VERTEX_POINT('',#53328);
#13892=VERTEX_POINT('',#53456);
#13893=VERTEX_POINT('',#53458);
#13894=VERTEX_POINT('',#53575);
#13895=VERTEX_POINT('',#53724);
#13896=VERTEX_POINT('',#53726);
#13897=VERTEX_POINT('',#53838);
#13898=VERTEX_POINT('',#53882);
#13899=VERTEX_POINT('',#54080);
#13900=VERTEX_POINT('',#54106);
#13901=VERTEX_POINT('',#54805);
#13902=VERTEX_POINT('',#54807);
#13903=VERTEX_POINT('',#54811);
#13904=VERTEX_POINT('',#54815);
#13905=VERTEX_POINT('',#54819);
#13906=VERTEX_POINT('',#54823);
#13907=VERTEX_POINT('',#54827);
#13908=VERTEX_POINT('',#54831);
#13909=VERTEX_POINT('',#54835);
#13910=VERTEX_POINT('',#54839);
#13911=VERTEX_POINT('',#54843);
#13912=VERTEX_POINT('',#54847);
#13913=VERTEX_POINT('',#54851);
#13914=VERTEX_POINT('',#54855);
#13915=VERTEX_POINT('',#54859);
#13916=VERTEX_POINT('',#54863);
#13917=VERTEX_POINT('',#54867);
#13918=VERTEX_POINT('',#54871);
#13919=VERTEX_POINT('',#54875);
#13920=VERTEX_POINT('',#54879);
#13921=VERTEX_POINT('',#54883);
#13922=VERTEX_POINT('',#54887);
#13923=VERTEX_POINT('',#54891);
#13924=VERTEX_POINT('',#54895);
#13925=VERTEX_POINT('',#54899);
#13926=VERTEX_POINT('',#54903);
#13927=VERTEX_POINT('',#54907);
#13928=VERTEX_POINT('',#54911);
#13929=VERTEX_POINT('',#54915);
#13930=VERTEX_POINT('',#54919);
#13931=VERTEX_POINT('',#54923);
#13932=VERTEX_POINT('',#54927);
#13933=VERTEX_POINT('',#54931);
#13934=VERTEX_POINT('',#54935);
#13935=VERTEX_POINT('',#54939);
#13936=VERTEX_POINT('',#54943);
#13937=VERTEX_POINT('',#54947);
#13938=VERTEX_POINT('',#54951);
#13939=VERTEX_POINT('',#54955);
#13940=VERTEX_POINT('',#54959);
#13941=VERTEX_POINT('',#54965);
#13942=VERTEX_POINT('',#54967);
#13943=VERTEX_POINT('',#54969);
#13944=VERTEX_POINT('',#54971);
#13945=VERTEX_POINT('',#54973);
#13946=VERTEX_POINT('',#54975);
#13947=VERTEX_POINT('',#54977);
#13948=VERTEX_POINT('',#54979);
#13949=VERTEX_POINT('',#54981);
#13950=VERTEX_POINT('',#54984);
#13951=VERTEX_POINT('',#54986);
#13952=VERTEX_POINT('',#54988);
#13953=VERTEX_POINT('',#54990);
#13954=VERTEX_POINT('',#54992);
#13955=VERTEX_POINT('',#54994);
#13956=VERTEX_POINT('',#54996);
#13957=VERTEX_POINT('',#54998);
#13958=VERTEX_POINT('',#55002);
#13959=VERTEX_POINT('',#55004);
#13960=VERTEX_POINT('',#55008);
#13961=VERTEX_POINT('',#55012);
#13962=VERTEX_POINT('',#55016);
#13963=VERTEX_POINT('',#55020);
#13964=VERTEX_POINT('',#55026);
#13965=VERTEX_POINT('',#55028);
#13966=VERTEX_POINT('',#55034);
#13967=VERTEX_POINT('',#55038);
#13968=VERTEX_POINT('',#55042);
#13969=VERTEX_POINT('',#55046);
#13970=VERTEX_POINT('',#55050);
#13971=VERTEX_POINT('',#55054);
#13972=VERTEX_POINT('',#55058);
#13973=VERTEX_POINT('',#55062);
#13974=VERTEX_POINT('',#55066);
#13975=VERTEX_POINT('',#55083);
#13976=VERTEX_POINT('',#55085);
#13977=VERTEX_POINT('',#55121);
#13978=VERTEX_POINT('',#55134);
#13979=VERTEX_POINT('',#55149);
#13980=VERTEX_POINT('',#55151);
#13981=VERTEX_POINT('',#55205);
#13982=VERTEX_POINT('',#55283);
#13983=VERTEX_POINT('',#55309);
#13984=VERTEX_POINT('',#55363);
#13985=VERTEX_POINT('',#55408);
#13986=VERTEX_POINT('',#55529);
#13987=VERTEX_POINT('',#55629);
#13988=VERTEX_POINT('',#55630);
#13989=VERTEX_POINT('',#55737);
#13990=VERTEX_POINT('',#55739);
#13991=VERTEX_POINT('',#55849);
#13992=VERTEX_POINT('',#55850);
#13993=VERTEX_POINT('',#55931);
#13994=VERTEX_POINT('',#55932);
#13995=VERTEX_POINT('',#56069);
#13996=VERTEX_POINT('',#56119);
#13997=VERTEX_POINT('',#56139);
#13998=VERTEX_POINT('',#56155);
#13999=VERTEX_POINT('',#56159);
#14000=VERTEX_POINT('',#56163);
#14001=VERTEX_POINT('',#56165);
#14002=VERTEX_POINT('',#56190);
#14003=VERTEX_POINT('',#56192);
#14004=VERTEX_POINT('',#56223);
#14005=VERTEX_POINT('',#56225);
#14006=VERTEX_POINT('',#56235);
#14007=VERTEX_POINT('',#56327);
#14008=VERTEX_POINT('',#56331);
#14009=VERTEX_POINT('',#56360);
#14010=VERTEX_POINT('',#56364);
#14011=VERTEX_POINT('',#56424);
#14012=VERTEX_POINT('',#56468);
#14013=VERTEX_POINT('',#56522);
#14014=VERTEX_POINT('',#56579);
#14015=VERTEX_POINT('',#56620);
#14016=VERTEX_POINT('',#56680);
#14017=VERTEX_POINT('',#56745);
#14018=VERTEX_POINT('',#56874);
#14019=VERTEX_POINT('',#56934);
#14020=VERTEX_POINT('',#56994);
#14021=VERTEX_POINT('',#57033);
#14022=VERTEX_POINT('',#57075);
#14023=VERTEX_POINT('',#57146);
#14024=VERTEX_POINT('',#57218);
#14025=VERTEX_POINT('',#57323);
#14026=VERTEX_POINT('',#57582);
#14027=VERTEX_POINT('',#57596);
#14028=VERTEX_POINT('',#57601);
#14029=VERTEX_POINT('',#57666);
#14030=VERTEX_POINT('',#57686);
#14031=VERTEX_POINT('',#57701);
#14032=VERTEX_POINT('',#57716);
#14033=VERTEX_POINT('',#57731);
#14034=VERTEX_POINT('',#57751);
#14035=VERTEX_POINT('',#57766);
#14036=VERTEX_POINT('',#57781);
#14037=VERTEX_POINT('',#57796);
#14038=VERTEX_POINT('',#57811);
#14039=VERTEX_POINT('',#57831);
#14040=VERTEX_POINT('',#57846);
#14041=VERTEX_POINT('',#57863);
#14042=VERTEX_POINT('',#57864);
#14043=VERTEX_POINT('',#57866);
#14044=VERTEX_POINT('',#57868);
#14045=VERTEX_POINT('',#57870);
#14046=VERTEX_POINT('',#57872);
#14047=VERTEX_POINT('',#57874);
#14048=VERTEX_POINT('',#57878);
#14049=VERTEX_POINT('',#57879);
#14050=VERTEX_POINT('',#57884);
#14051=VERTEX_POINT('',#57888);
#14052=VERTEX_POINT('',#57892);
#14053=VERTEX_POINT('',#57896);
#14054=VERTEX_POINT('',#57900);
#16672=EDGE_CURVE('',#13631,#13632,#7640,.T.);
#16673=EDGE_CURVE('',#13631,#13633,#11323,.T.);
#16674=EDGE_CURVE('',#13633,#13634,#7641,.T.);
#16675=EDGE_CURVE('',#13632,#13634,#11324,.T.);
#16676=EDGE_CURVE('',#13635,#13636,#7642,.T.);
#16677=EDGE_CURVE('',#13636,#13637,#11325,.T.);
#16678=EDGE_CURVE('',#13637,#13638,#11326,.T.);
#16679=EDGE_CURVE('',#13638,#13639,#11327,.T.);
#16680=EDGE_CURVE('',#13639,#13640,#7643,.T.);
#16681=EDGE_CURVE('',#13640,#13641,#11328,.T.);
#16682=EDGE_CURVE('',#13641,#13642,#7644,.T.);
#16683=EDGE_CURVE('',#13642,#13643,#11329,.T.);
#16684=EDGE_CURVE('',#13643,#13644,#7645,.T.);
#16685=EDGE_CURVE('',#13644,#13645,#11330,.T.);
#16686=EDGE_CURVE('',#13645,#13646,#11331,.T.);
#16687=EDGE_CURVE('',#13646,#13647,#11332,.T.);
#16688=EDGE_CURVE('',#13647,#13648,#7646,.T.);
#16689=EDGE_CURVE('',#13648,#13649,#11333,.T.);
#16690=EDGE_CURVE('',#13649,#13650,#7647,.T.);
#16691=EDGE_CURVE('',#13650,#13651,#11334,.T.);
#16692=EDGE_CURVE('',#13651,#13652,#7648,.T.);
#16693=EDGE_CURVE('',#13652,#13653,#11335,.T.);
#16694=EDGE_CURVE('',#13653,#13654,#11336,.T.);
#16695=EDGE_CURVE('',#13654,#13655,#11337,.T.);
#16696=EDGE_CURVE('',#13655,#13656,#7649,.T.);
#16697=EDGE_CURVE('',#13656,#13657,#11338,.T.);
#16698=EDGE_CURVE('',#13657,#13658,#11339,.T.);
#16699=EDGE_CURVE('',#13658,#13659,#11340,.T.);
#16700=EDGE_CURVE('',#13659,#13660,#7650,.T.);
#16701=EDGE_CURVE('',#13660,#13661,#11341,.T.);
#16702=EDGE_CURVE('',#13661,#13662,#7651,.T.);
#16703=EDGE_CURVE('',#13662,#13663,#11342,.T.);
#16704=EDGE_CURVE('',#13663,#13664,#7652,.T.);
#16705=EDGE_CURVE('',#13664,#13665,#11343,.T.);
#16706=EDGE_CURVE('',#13665,#13666,#11344,.T.);
#16707=EDGE_CURVE('',#13666,#13667,#11345,.T.);
#16708=EDGE_CURVE('',#13667,#13668,#7653,.T.);
#16709=EDGE_CURVE('',#13668,#13669,#11346,.T.);
#16710=EDGE_CURVE('',#13669,#13670,#7654,.T.);
#16711=EDGE_CURVE('',#13670,#13671,#11347,.T.);
#16712=EDGE_CURVE('',#13671,#13672,#7655,.T.);
#16713=EDGE_CURVE('',#13672,#13673,#11348,.T.);
#16714=EDGE_CURVE('',#13673,#13674,#11349,.T.);
#16715=EDGE_CURVE('',#13674,#13635,#11350,.T.);
#16716=EDGE_CURVE('',#13675,#13676,#11351,.T.);
#16717=EDGE_CURVE('',#13677,#13676,#1332,.T.);
#16718=EDGE_CURVE('',#13678,#13677,#1333,.T.);
#16719=EDGE_CURVE('',#13679,#13678,#1334,.T.);
#16720=EDGE_CURVE('',#13679,#13680,#1335,.T.);
#16721=EDGE_CURVE('',#13681,#13680,#1336,.T.);
#16722=EDGE_CURVE('',#13681,#13682,#11352,.T.);
#16723=EDGE_CURVE('',#13683,#13682,#7656,.T.);
#16724=EDGE_CURVE('',#13683,#13684,#11353,.T.);
#16725=EDGE_CURVE('',#13675,#13684,#1337,.T.);
#16726=EDGE_CURVE('',#13685,#13686,#11354,.T.);
#16727=EDGE_CURVE('',#13687,#13686,#11355,.T.);
#16728=EDGE_CURVE('',#13688,#13687,#11356,.T.);
#16729=EDGE_CURVE('',#13688,#13632,#7657,.T.);
#16730=EDGE_CURVE('',#13689,#13634,#11357,.T.);
#16731=EDGE_CURVE('',#13689,#13690,#11358,.T.);
#16732=EDGE_CURVE('',#13691,#13690,#11359,.T.);
#16733=EDGE_CURVE('',#13685,#13691,#7658,.T.);
#16734=EDGE_CURVE('',#13692,#13693,#7659,.T.);
#16735=EDGE_CURVE('',#13694,#13693,#11360,.T.);
#16736=EDGE_CURVE('',#13694,#13695,#1338,.T.);
#16737=EDGE_CURVE('',#13696,#13695,#1339,.T.);
#16738=EDGE_CURVE('',#13696,#13697,#1340,.T.);
#16739=EDGE_CURVE('',#13697,#13698,#1341,.T.);
#16740=EDGE_CURVE('',#13698,#13699,#1342,.T.);
#16741=EDGE_CURVE('',#13700,#13699,#11361,.T.);
#16742=EDGE_CURVE('',#13700,#13701,#1343,.T.);
#16743=EDGE_CURVE('',#13692,#13701,#11362,.T.);
#16744=EDGE_CURVE('',#13702,#13703,#7660,.T.);
#16745=EDGE_CURVE('',#13703,#13704,#1344,.T.);
#16746=EDGE_CURVE('',#13705,#13704,#7661,.T.);
#16747=EDGE_CURVE('',#13706,#13705,#1345,.T.);
#16748=EDGE_CURVE('',#13702,#13706,#1346,.T.);
#16749=EDGE_CURVE('',#13631,#13707,#11363,.T.);
#16750=EDGE_CURVE('',#13633,#13707,#11364,.T.);
#16751=EDGE_CURVE('',#13708,#13709,#7662,.T.);
#16752=EDGE_CURVE('',#13709,#13710,#7663,.T.);
#16753=EDGE_CURVE('',#13711,#13710,#7664,.T.);
#16754=EDGE_CURVE('',#13708,#13711,#7665,.T.);
#16755=EDGE_CURVE('',#13684,#13712,#7666,.T.);
#16756=EDGE_CURVE('',#13713,#13712,#1347,.T.);
#16757=EDGE_CURVE('',#13675,#13713,#7667,.T.);
#16758=EDGE_CURVE('',#13683,#13714,#7668,.T.);
#16759=EDGE_CURVE('',#13715,#13714,#1348,.T.);
#16760=EDGE_CURVE('',#13712,#13715,#449,.T.);
#16761=EDGE_CURVE('',#13682,#13716,#7669,.T.);
#16762=EDGE_CURVE('',#13714,#13716,#7670,.T.);
#16763=EDGE_CURVE('',#13681,#13717,#7671,.T.);
#16764=EDGE_CURVE('',#13718,#13717,#450,.T.);
#16765=EDGE_CURVE('',#13719,#13718,#1349,.T.);
#16766=EDGE_CURVE('',#13716,#13719,#451,.T.);
#16767=EDGE_CURVE('',#13680,#13720,#7672,.T.);
#16768=EDGE_CURVE('',#13721,#13720,#1350,.T.);
#16769=EDGE_CURVE('',#13722,#13721,#452,.T.);
#16770=EDGE_CURVE('',#13723,#13722,#1351,.T.);
#16771=EDGE_CURVE('',#13717,#13723,#11365,.T.);
#16772=EDGE_CURVE('',#13679,#13724,#7673,.T.);
#16773=EDGE_CURVE('',#13725,#13724,#1352,.T.);
#16774=EDGE_CURVE('',#13720,#13725,#1353,.T.);
#16775=EDGE_CURVE('',#13678,#13726,#7674,.T.);
#16776=EDGE_CURVE('',#13727,#13726,#1354,.T.);
#16777=EDGE_CURVE('',#13728,#13727,#1355,.T.);
#16778=EDGE_CURVE('',#13729,#13728,#1356,.T.);
#16779=EDGE_CURVE('',#13724,#13729,#453,.T.);
#16780=EDGE_CURVE('',#13677,#13730,#7675,.T.);
#16781=EDGE_CURVE('',#13730,#13731,#1357,.T.);
#16782=EDGE_CURVE('',#13726,#13731,#1358,.T.);
#16783=EDGE_CURVE('',#13676,#13732,#7676,.T.);
#16784=EDGE_CURVE('',#13733,#13732,#1359,.T.);
#16785=EDGE_CURVE('',#13733,#13730,#1360,.T.);
#16786=EDGE_CURVE('',#13734,#13713,#454,.T.);
#16787=EDGE_CURVE('',#13735,#13734,#1361,.T.);
#16788=EDGE_CURVE('',#13732,#13735,#1362,.T.);
#16789=EDGE_CURVE('',#13701,#13736,#7677,.T.);
#16790=EDGE_CURVE('',#13736,#13737,#455,.T.);
#16791=EDGE_CURVE('',#13737,#13738,#1363,.T.);
#16792=EDGE_CURVE('',#13692,#13738,#7678,.T.);
#16793=EDGE_CURVE('',#13700,#13739,#7679,.T.);
#16794=EDGE_CURVE('',#13739,#13736,#1364,.T.);
#16795=EDGE_CURVE('',#13699,#13740,#7680,.T.);
#16796=EDGE_CURVE('',#13740,#13741,#1365,.T.);
#16797=EDGE_CURVE('',#13741,#13742,#1366,.T.);
#16798=EDGE_CURVE('',#13742,#13739,#456,.T.);
#16799=EDGE_CURVE('',#13698,#13743,#7681,.T.);
#16800=EDGE_CURVE('',#13744,#13743,#1367,.T.);
#16801=EDGE_CURVE('',#13744,#13740,#1368,.T.);
#16802=EDGE_CURVE('',#13697,#13745,#7682,.T.);
#16803=EDGE_CURVE('',#13745,#13746,#1369,.T.);
#16804=EDGE_CURVE('',#13743,#13746,#1370,.T.);
#16805=EDGE_CURVE('',#13696,#13747,#7683,.T.);
#16806=EDGE_CURVE('',#13747,#13748,#457,.T.);
#16807=EDGE_CURVE('',#13748,#13749,#1371,.T.);
#16808=EDGE_CURVE('',#13749,#13750,#1372,.T.);
#16809=EDGE_CURVE('',#13750,#13745,#1373,.T.);
#16810=EDGE_CURVE('',#13695,#13751,#7684,.T.);
#16811=EDGE_CURVE('',#13751,#13752,#1374,.T.);
#16812=EDGE_CURVE('',#13752,#13747,#1375,.T.);
#16813=EDGE_CURVE('',#13694,#13753,#7685,.T.);
#16814=EDGE_CURVE('',#13753,#13754,#11366,.T.);
#16815=EDGE_CURVE('',#13754,#13755,#1376,.T.);
#16816=EDGE_CURVE('',#13755,#13756,#458,.T.);
#16817=EDGE_CURVE('',#13756,#13751,#1377,.T.);
#16818=EDGE_CURVE('',#13693,#13757,#7686,.T.);
#16819=EDGE_CURVE('',#13757,#13758,#459,.T.);
#16820=EDGE_CURVE('',#13758,#13759,#1378,.T.);
#16821=EDGE_CURVE('',#13759,#13753,#460,.T.);
#16822=EDGE_CURVE('',#13738,#13757,#7687,.T.);
#16823=EDGE_CURVE('',#13760,#13761,#11367,.T.);
#16824=EDGE_CURVE('',#13761,#13762,#7688,.T.);
#16825=EDGE_CURVE('',#13763,#13762,#11368,.T.);
#16826=EDGE_CURVE('',#13760,#13763,#7689,.T.);
#16827=EDGE_CURVE('',#13665,#13763,#11369,.T.);
#16828=EDGE_CURVE('',#13666,#13762,#11370,.T.);
#16829=EDGE_CURVE('',#13664,#13764,#11371,.T.);
#16830=EDGE_CURVE('',#13764,#13763,#11372,.T.);
#16831=EDGE_CURVE('',#13765,#13764,#7690,.T.);
#16832=EDGE_CURVE('',#13765,#13760,#11373,.T.);
#16833=EDGE_CURVE('',#13663,#13766,#11374,.T.);
#16834=EDGE_CURVE('',#13766,#13764,#7691,.T.);
#16835=EDGE_CURVE('',#13766,#13767,#7692,.T.);
#16836=EDGE_CURVE('',#13767,#13765,#7693,.T.);
#16837=EDGE_CURVE('',#13662,#13768,#11375,.T.);
#16838=EDGE_CURVE('',#13768,#13766,#11376,.T.);
#16839=EDGE_CURVE('',#13768,#13769,#7694,.T.);
#16840=EDGE_CURVE('',#13769,#13767,#11377,.T.);
#16841=EDGE_CURVE('',#13661,#13770,#11378,.T.);
#16842=EDGE_CURVE('',#13770,#13768,#7695,.T.);
#16843=EDGE_CURVE('',#13770,#13771,#7696,.T.);
#16844=EDGE_CURVE('',#13771,#13769,#7697,.T.);
#16845=EDGE_CURVE('',#13660,#13772,#11379,.T.);
#16846=EDGE_CURVE('',#13772,#13770,#11380,.T.);
#16847=EDGE_CURVE('',#13772,#13773,#7698,.T.);
#16848=EDGE_CURVE('',#13773,#13771,#11381,.T.);
#16849=EDGE_CURVE('',#13659,#13774,#11382,.T.);
#16850=EDGE_CURVE('',#13774,#13772,#7699,.T.);
#16851=EDGE_CURVE('',#13775,#13774,#7700,.T.);
#16852=EDGE_CURVE('',#13775,#13773,#7701,.T.);
#16853=EDGE_CURVE('',#13658,#13776,#11383,.T.);
#16854=EDGE_CURVE('',#13776,#13774,#11384,.T.);
#16855=EDGE_CURVE('',#13777,#13776,#7702,.T.);
#16856=EDGE_CURVE('',#13777,#13775,#11385,.T.);
#16857=EDGE_CURVE('',#13657,#13778,#11386,.T.);
#16858=EDGE_CURVE('',#13778,#13776,#11387,.T.);
#16859=EDGE_CURVE('',#13779,#13778,#7703,.T.);
#16860=EDGE_CURVE('',#13779,#13777,#11388,.T.);
#16861=EDGE_CURVE('',#13656,#13780,#11389,.T.);
#16862=EDGE_CURVE('',#13780,#13778,#11390,.T.);
#16863=EDGE_CURVE('',#13781,#13780,#7704,.T.);
#16864=EDGE_CURVE('',#13781,#13779,#11391,.T.);
#16865=EDGE_CURVE('',#13655,#13782,#11392,.T.);
#16866=EDGE_CURVE('',#13782,#13780,#7705,.T.);
#16867=EDGE_CURVE('',#13783,#13782,#7706,.T.);
#16868=EDGE_CURVE('',#13783,#13781,#7707,.T.);
#16869=EDGE_CURVE('',#13654,#13784,#11393,.T.);
#16870=EDGE_CURVE('',#13784,#13782,#11394,.T.);
#16871=EDGE_CURVE('',#13785,#13784,#7708,.T.);
#16872=EDGE_CURVE('',#13785,#13783,#11395,.T.);
#16873=EDGE_CURVE('',#13653,#13786,#11396,.T.);
#16874=EDGE_CURVE('',#13786,#13784,#11397,.T.);
#16875=EDGE_CURVE('',#13787,#13786,#7709,.T.);
#16876=EDGE_CURVE('',#13787,#13785,#11398,.T.);
#16877=EDGE_CURVE('',#13652,#13788,#11399,.T.);
#16878=EDGE_CURVE('',#13788,#13786,#11400,.T.);
#16879=EDGE_CURVE('',#13789,#13788,#7710,.T.);
#16880=EDGE_CURVE('',#13789,#13787,#11401,.T.);
#16881=EDGE_CURVE('',#13651,#13790,#11402,.T.);
#16882=EDGE_CURVE('',#13790,#13788,#7711,.T.);
#16883=EDGE_CURVE('',#13790,#13791,#7712,.T.);
#16884=EDGE_CURVE('',#13791,#13789,#7713,.T.);
#16885=EDGE_CURVE('',#13650,#13792,#11403,.T.);
#16886=EDGE_CURVE('',#13792,#13790,#11404,.T.);
#16887=EDGE_CURVE('',#13792,#13793,#7714,.T.);
#16888=EDGE_CURVE('',#13793,#13791,#11405,.T.);
#16889=EDGE_CURVE('',#13649,#13794,#11406,.T.);
#16890=EDGE_CURVE('',#13794,#13792,#7715,.T.);
#16891=EDGE_CURVE('',#13794,#13795,#7716,.T.);
#16892=EDGE_CURVE('',#13795,#13793,#7717,.T.);
#16893=EDGE_CURVE('',#13648,#13796,#11407,.T.);
#16894=EDGE_CURVE('',#13796,#13794,#11408,.T.);
#16895=EDGE_CURVE('',#13796,#13797,#7718,.T.);
#16896=EDGE_CURVE('',#13797,#13795,#11409,.T.);
#16897=EDGE_CURVE('',#13647,#13798,#11410,.T.);
#16898=EDGE_CURVE('',#13798,#13796,#7719,.T.);
#16899=EDGE_CURVE('',#13799,#13798,#7720,.T.);
#16900=EDGE_CURVE('',#13799,#13797,#7721,.T.);
#16901=EDGE_CURVE('',#13646,#13800,#11411,.T.);
#16902=EDGE_CURVE('',#13800,#13798,#11412,.T.);
#16903=EDGE_CURVE('',#13801,#13800,#7722,.T.);
#16904=EDGE_CURVE('',#13801,#13799,#11413,.T.);
#16905=EDGE_CURVE('',#13802,#13801,#11414,.T.);
#16906=EDGE_CURVE('',#13803,#13800,#11415,.T.);
#16907=EDGE_CURVE('',#13802,#13803,#7723,.T.);
#16908=EDGE_CURVE('',#13645,#13803,#11416,.T.);
#16909=EDGE_CURVE('',#13644,#13804,#11417,.T.);
#16910=EDGE_CURVE('',#13804,#13803,#11418,.T.);
#16911=EDGE_CURVE('',#13805,#13804,#7724,.T.);
#16912=EDGE_CURVE('',#13805,#13802,#11419,.T.);
#16913=EDGE_CURVE('',#13643,#13806,#11420,.T.);
#16914=EDGE_CURVE('',#13806,#13804,#7725,.T.);
#16915=EDGE_CURVE('',#13806,#13807,#7726,.T.);
#16916=EDGE_CURVE('',#13807,#13805,#7727,.T.);
#16917=EDGE_CURVE('',#13642,#13808,#11421,.T.);
#16918=EDGE_CURVE('',#13808,#13806,#11422,.T.);
#16919=EDGE_CURVE('',#13808,#13809,#7728,.T.);
#16920=EDGE_CURVE('',#13809,#13807,#11423,.T.);
#16921=EDGE_CURVE('',#13641,#13810,#11424,.T.);
#16922=EDGE_CURVE('',#13810,#13808,#7729,.T.);
#16923=EDGE_CURVE('',#13810,#13811,#7730,.T.);
#16924=EDGE_CURVE('',#13811,#13809,#7731,.T.);
#16925=EDGE_CURVE('',#13640,#13812,#11425,.T.);
#16926=EDGE_CURVE('',#13812,#13810,#11426,.T.);
#16927=EDGE_CURVE('',#13812,#13813,#7732,.T.);
#16928=EDGE_CURVE('',#13813,#13811,#11427,.T.);
#16929=EDGE_CURVE('',#13639,#13814,#11428,.T.);
#16930=EDGE_CURVE('',#13814,#13812,#7733,.T.);
#16931=EDGE_CURVE('',#13815,#13814,#7734,.T.);
#16932=EDGE_CURVE('',#13815,#13813,#7735,.T.);
#16933=EDGE_CURVE('',#13638,#13816,#11429,.T.);
#16934=EDGE_CURVE('',#13816,#13814,#11430,.T.);
#16935=EDGE_CURVE('',#13817,#13816,#7736,.T.);
#16936=EDGE_CURVE('',#13817,#13815,#11431,.T.);
#16937=EDGE_CURVE('',#13637,#13818,#11432,.T.);
#16938=EDGE_CURVE('',#13818,#13816,#11433,.T.);
#16939=EDGE_CURVE('',#13819,#13818,#7737,.T.);
#16940=EDGE_CURVE('',#13819,#13817,#11434,.T.);
#16941=EDGE_CURVE('',#13636,#13820,#11435,.T.);
#16942=EDGE_CURVE('',#13820,#13818,#11436,.T.);
#16943=EDGE_CURVE('',#13821,#13820,#7738,.T.);
#16944=EDGE_CURVE('',#13821,#13819,#11437,.T.);
#16945=EDGE_CURVE('',#13635,#13822,#11438,.T.);
#16946=EDGE_CURVE('',#13822,#13820,#7739,.T.);
#16947=EDGE_CURVE('',#13823,#13822,#7740,.T.);
#16948=EDGE_CURVE('',#13823,#13821,#7741,.T.);
#16949=EDGE_CURVE('',#13674,#13824,#11439,.T.);
#16950=EDGE_CURVE('',#13824,#13822,#11440,.T.);
#16951=EDGE_CURVE('',#13825,#13824,#7742,.T.);
#16952=EDGE_CURVE('',#13825,#13823,#11441,.T.);
#16953=EDGE_CURVE('',#13673,#13826,#11442,.T.);
#16954=EDGE_CURVE('',#13826,#13824,#11443,.T.);
#16955=EDGE_CURVE('',#13827,#13826,#7743,.T.);
#16956=EDGE_CURVE('',#13827,#13825,#11444,.T.);
#16957=EDGE_CURVE('',#13672,#13828,#11445,.T.);
#16958=EDGE_CURVE('',#13828,#13826,#11446,.T.);
#16959=EDGE_CURVE('',#13829,#13828,#7744,.T.);
#16960=EDGE_CURVE('',#13829,#13827,#11447,.T.);
#16961=EDGE_CURVE('',#13671,#13830,#11448,.T.);
#16962=EDGE_CURVE('',#13830,#13828,#7745,.T.);
#16963=EDGE_CURVE('',#13830,#13831,#7746,.T.);
#16964=EDGE_CURVE('',#13831,#13829,#7747,.T.);
#16965=EDGE_CURVE('',#13670,#13832,#11449,.T.);
#16966=EDGE_CURVE('',#13832,#13830,#11450,.T.);
#16967=EDGE_CURVE('',#13832,#13833,#7748,.T.);
#16968=EDGE_CURVE('',#13833,#13831,#11451,.T.);
#16969=EDGE_CURVE('',#13669,#13834,#11452,.T.);
#16970=EDGE_CURVE('',#13834,#13832,#7749,.T.);
#16971=EDGE_CURVE('',#13834,#13835,#7750,.T.);
#16972=EDGE_CURVE('',#13835,#13833,#7751,.T.);
#16973=EDGE_CURVE('',#13762,#13836,#11453,.T.);
#16974=EDGE_CURVE('',#13667,#13836,#11454,.T.);
#16975=EDGE_CURVE('',#13761,#13837,#11455,.T.);
#16976=EDGE_CURVE('',#13837,#13836,#7752,.T.);
#16977=EDGE_CURVE('',#13668,#13838,#11456,.T.);
#16978=EDGE_CURVE('',#13838,#13834,#11457,.T.);
#16979=EDGE_CURVE('',#13838,#13839,#7753,.T.);
#16980=EDGE_CURVE('',#13839,#13835,#11458,.T.);
#16981=EDGE_CURVE('',#13836,#13838,#7754,.T.);
#16982=EDGE_CURVE('',#13837,#13839,#7755,.T.);
#16983=EDGE_CURVE('',#13840,#13841,#7756,.T.);
#16984=EDGE_CURVE('',#13842,#13841,#7757,.T.);
#16985=EDGE_CURVE('',#13843,#13842,#7758,.T.);
#16986=EDGE_CURVE('',#13840,#13843,#7759,.T.);
#16987=EDGE_CURVE('',#13844,#13845,#7760,.T.);
#16988=EDGE_CURVE('',#13846,#13845,#1379,.T.);
#16989=EDGE_CURVE('',#13847,#13846,#7761,.T.);
#16990=EDGE_CURVE('',#13844,#13847,#1380,.T.);
#16991=EDGE_CURVE('',#13848,#13849,#7762,.T.);
#16992=EDGE_CURVE('',#13849,#13845,#7763,.T.);
#16993=EDGE_CURVE('',#13850,#13844,#461,.T.);
#16994=EDGE_CURVE('',#13848,#13850,#7764,.T.);
#16995=EDGE_CURVE('',#13846,#13851,#1381,.T.);
#16996=EDGE_CURVE('',#13852,#13851,#7765,.T.);
#16997=EDGE_CURVE('',#13853,#13852,#1382,.T.);
#16998=EDGE_CURVE('',#13847,#13853,#11459,.T.);
#16999=EDGE_CURVE('',#13851,#13854,#1383,.T.);
#17000=EDGE_CURVE('',#13855,#13854,#7766,.T.);
#17001=EDGE_CURVE('',#13852,#13855,#1384,.T.);
#17002=EDGE_CURVE('',#13854,#13703,#1385,.T.);
#17003=EDGE_CURVE('',#13855,#13702,#1386,.T.);
#17004=EDGE_CURVE('',#13856,#13857,#7767,.T.);
#17005=EDGE_CURVE('',#13858,#13857,#11460,.T.);
#17006=EDGE_CURVE('',#13859,#13858,#7768,.T.);
#17007=EDGE_CURVE('',#13856,#13859,#1387,.T.);
#17008=EDGE_CURVE('',#13860,#13861,#7769,.T.);
#17009=EDGE_CURVE('',#13861,#13862,#1388,.T.);
#17010=EDGE_CURVE('',#13863,#13862,#7770,.T.);
#17011=EDGE_CURVE('',#13860,#13863,#1389,.T.);
#17012=EDGE_CURVE('',#13864,#13865,#7771,.T.);
#17013=EDGE_CURVE('',#13865,#13861,#11461,.T.);
#17014=EDGE_CURVE('',#13864,#13860,#1390,.T.);
#17015=EDGE_CURVE('',#13865,#13704,#1391,.T.);
#17016=EDGE_CURVE('',#13866,#13864,#1392,.T.);
#17017=EDGE_CURVE('',#13705,#13866,#1393,.T.);
#17018=EDGE_CURVE('',#13867,#13868,#7772,.T.);
#17019=EDGE_CURVE('',#13868,#13710,#7773,.T.);
#17020=EDGE_CURVE('',#13867,#13709,#7774,.T.);
#17021=EDGE_CURVE('',#13869,#13843,#7775,.T.);
#17022=EDGE_CURVE('',#13842,#13870,#7776,.T.);
#17023=EDGE_CURVE('',#13869,#13870,#7777,.T.);
#17024=EDGE_CURVE('',#13712,#13871,#11462,.T.);
#17025=EDGE_CURVE('',#13872,#13871,#1394,.T.);
#17026=EDGE_CURVE('',#13713,#13872,#11463,.T.);
#17027=EDGE_CURVE('',#13714,#13873,#11464,.T.);
#17028=EDGE_CURVE('',#13874,#13873,#1395,.T.);
#17029=EDGE_CURVE('',#13715,#13874,#11465,.T.);
#17030=EDGE_CURVE('',#13871,#13874,#1396,.T.);
#17031=EDGE_CURVE('',#13716,#13875,#11466,.T.);
#17032=EDGE_CURVE('',#13873,#13875,#7778,.T.);
#17033=EDGE_CURVE('',#13717,#13876,#11467,.T.);
#17034=EDGE_CURVE('',#13877,#13876,#11468,.T.);
#17035=EDGE_CURVE('',#13718,#13877,#11469,.T.);
#17036=EDGE_CURVE('',#13878,#13877,#1397,.T.);
#17037=EDGE_CURVE('',#13719,#13878,#11470,.T.);
#17038=EDGE_CURVE('',#13875,#13878,#462,.T.);
#17039=EDGE_CURVE('',#13722,#13879,#11471,.T.);
#17040=EDGE_CURVE('',#13880,#13879,#1398,.T.);
#17041=EDGE_CURVE('',#13723,#13880,#11472,.T.);
#17042=EDGE_CURVE('',#13721,#13881,#11473,.T.);
#17043=EDGE_CURVE('',#13879,#13881,#1399,.T.);
#17044=EDGE_CURVE('',#13720,#13882,#11474,.T.);
#17045=EDGE_CURVE('',#13881,#13882,#1400,.T.);
#17046=EDGE_CURVE('',#13876,#13880,#1401,.T.);
#17047=EDGE_CURVE('',#13725,#13883,#11475,.T.);
#17048=EDGE_CURVE('',#13882,#13883,#1402,.T.);
#17049=EDGE_CURVE('',#13724,#13884,#11476,.T.);
#17050=EDGE_CURVE('',#13883,#13884,#1403,.T.);
#17051=EDGE_CURVE('',#13729,#13885,#11477,.T.);
#17052=EDGE_CURVE('',#13884,#13885,#1404,.T.);
#17053=EDGE_CURVE('',#13728,#13886,#11478,.T.);
#17054=EDGE_CURVE('',#13885,#13886,#1405,.T.);
#17055=EDGE_CURVE('',#13727,#13887,#11479,.T.);
#17056=EDGE_CURVE('',#13886,#13887,#1406,.T.);
#17057=EDGE_CURVE('',#13726,#13888,#11480,.T.);
#17058=EDGE_CURVE('',#13887,#13888,#1407,.T.);
#17059=EDGE_CURVE('',#13888,#13731,#1408,.T.);
#17060=EDGE_CURVE('',#13730,#13889,#7779,.T.);
#17061=EDGE_CURVE('',#13890,#13889,#1409,.T.);
#17062=EDGE_CURVE('',#13887,#13890,#7780,.T.);
#17063=EDGE_CURVE('',#13733,#13891,#1410,.T.);
#17064=EDGE_CURVE('',#13891,#13892,#463,.T.);
#17065=EDGE_CURVE('',#13892,#13893,#7781,.T.);
#17066=EDGE_CURVE('',#13889,#13893,#1411,.T.);
#17067=EDGE_CURVE('',#13732,#13891,#11481,.T.);
#17068=EDGE_CURVE('',#13894,#13872,#464,.T.);
#17069=EDGE_CURVE('',#13734,#13894,#11482,.T.);
#17070=EDGE_CURVE('',#13892,#13894,#1412,.T.);
#17071=EDGE_CURVE('',#13735,#13892,#11483,.T.);
#17072=EDGE_CURVE('',#13736,#13895,#11484,.T.);
#17073=EDGE_CURVE('',#13895,#13896,#1413,.T.);
#17074=EDGE_CURVE('',#13737,#13896,#11485,.T.);
#17075=EDGE_CURVE('',#13896,#13848,#1414,.T.);
#17076=EDGE_CURVE('',#13738,#13848,#11486,.T.);
#17077=EDGE_CURVE('',#13739,#13897,#11487,.T.);
#17078=EDGE_CURVE('',#13897,#13895,#1415,.T.);
#17079=EDGE_CURVE('',#13740,#13898,#11488,.T.);
#17080=EDGE_CURVE('',#13898,#13856,#465,.T.);
#17081=EDGE_CURVE('',#13741,#13856,#11489,.T.);
#17082=EDGE_CURVE('',#13742,#13859,#11490,.T.);
#17083=EDGE_CURVE('',#13859,#13897,#466,.T.);
#17084=EDGE_CURVE('',#13744,#13898,#1416,.T.);
#17085=EDGE_CURVE('',#13743,#13899,#7782,.T.);
#17086=EDGE_CURVE('',#13899,#13857,#1417,.T.);
#17087=EDGE_CURVE('',#13862,#13899,#1418,.T.);
#17088=EDGE_CURVE('',#13900,#13746,#1419,.T.);
#17089=EDGE_CURVE('',#13863,#13900,#1420,.T.);
#17090=EDGE_CURVE('',#13745,#13900,#11491,.T.);
#17091=EDGE_CURVE('',#13750,#13863,#11492,.T.);
#17092=EDGE_CURVE('',#13749,#13860,#11493,.T.);
#17093=EDGE_CURVE('',#13748,#13864,#11494,.T.);
#17094=EDGE_CURVE('',#13747,#13866,#11495,.T.);
#17095=EDGE_CURVE('',#13752,#13705,#11496,.T.);
#17096=EDGE_CURVE('',#13751,#13706,#11497,.T.);
#17097=EDGE_CURVE('',#13756,#13702,#11498,.T.);
#17098=EDGE_CURVE('',#13755,#13855,#11499,.T.);
#17099=EDGE_CURVE('',#13754,#13852,#11500,.T.);
#17100=EDGE_CURVE('',#13753,#13853,#11501,.T.);
#17101=EDGE_CURVE('',#13757,#13850,#11502,.T.);
#17102=EDGE_CURVE('',#13758,#13844,#11503,.T.);
#17103=EDGE_CURVE('',#13759,#13847,#11504,.T.);
#17104=EDGE_CURVE('',#13760,#13901,#11505,.T.);
#17105=EDGE_CURVE('',#13901,#13902,#11506,.T.);
#17106=EDGE_CURVE('',#13761,#13902,#11507,.T.);
#17107=EDGE_CURVE('',#13765,#13903,#11508,.T.);
#17108=EDGE_CURVE('',#13903,#13901,#11509,.T.);
#17109=EDGE_CURVE('',#13767,#13904,#11510,.T.);
#17110=EDGE_CURVE('',#13904,#13903,#7783,.T.);
#17111=EDGE_CURVE('',#13769,#13905,#11511,.T.);
#17112=EDGE_CURVE('',#13905,#13904,#11512,.T.);
#17113=EDGE_CURVE('',#13771,#13906,#11513,.T.);
#17114=EDGE_CURVE('',#13906,#13905,#7784,.T.);
#17115=EDGE_CURVE('',#13773,#13907,#11514,.T.);
#17116=EDGE_CURVE('',#13907,#13906,#11515,.T.);
#17117=EDGE_CURVE('',#13775,#13908,#11516,.T.);
#17118=EDGE_CURVE('',#13908,#13907,#7785,.T.);
#17119=EDGE_CURVE('',#13777,#13909,#11517,.T.);
#17120=EDGE_CURVE('',#13909,#13908,#11518,.T.);
#17121=EDGE_CURVE('',#13779,#13910,#11519,.T.);
#17122=EDGE_CURVE('',#13910,#13909,#11520,.T.);
#17123=EDGE_CURVE('',#13781,#13911,#11521,.T.);
#17124=EDGE_CURVE('',#13911,#13910,#11522,.T.);
#17125=EDGE_CURVE('',#13783,#13912,#11523,.T.);
#17126=EDGE_CURVE('',#13912,#13911,#7786,.T.);
#17127=EDGE_CURVE('',#13785,#13913,#11524,.T.);
#17128=EDGE_CURVE('',#13913,#13912,#11525,.T.);
#17129=EDGE_CURVE('',#13787,#13914,#11526,.T.);
#17130=EDGE_CURVE('',#13914,#13913,#11527,.T.);
#17131=EDGE_CURVE('',#13789,#13915,#11528,.T.);
#17132=EDGE_CURVE('',#13915,#13914,#11529,.T.);
#17133=EDGE_CURVE('',#13791,#13916,#11530,.T.);
#17134=EDGE_CURVE('',#13916,#13915,#7787,.T.);
#17135=EDGE_CURVE('',#13793,#13917,#11531,.T.);
#17136=EDGE_CURVE('',#13917,#13916,#11532,.T.);
#17137=EDGE_CURVE('',#13795,#13918,#11533,.T.);
#17138=EDGE_CURVE('',#13918,#13917,#7788,.T.);
#17139=EDGE_CURVE('',#13797,#13919,#11534,.T.);
#17140=EDGE_CURVE('',#13919,#13918,#11535,.T.);
#17141=EDGE_CURVE('',#13799,#13920,#11536,.T.);
#17142=EDGE_CURVE('',#13920,#13919,#7789,.T.);
#17143=EDGE_CURVE('',#13801,#13921,#11537,.T.);
#17144=EDGE_CURVE('',#13921,#13920,#11538,.T.);
#17145=EDGE_CURVE('',#13802,#13922,#11539,.T.);
#17146=EDGE_CURVE('',#13922,#13921,#11540,.T.);
#17147=EDGE_CURVE('',#13805,#13923,#11541,.T.);
#17148=EDGE_CURVE('',#13923,#13922,#11542,.T.);
#17149=EDGE_CURVE('',#13807,#13924,#11543,.T.);
#17150=EDGE_CURVE('',#13924,#13923,#7790,.T.);
#17151=EDGE_CURVE('',#13809,#13925,#11544,.T.);
#17152=EDGE_CURVE('',#13925,#13924,#11545,.T.);
#17153=EDGE_CURVE('',#13811,#13926,#11546,.T.);
#17154=EDGE_CURVE('',#13926,#13925,#7791,.T.);
#17155=EDGE_CURVE('',#13813,#13927,#11547,.T.);
#17156=EDGE_CURVE('',#13927,#13926,#11548,.T.);
#17157=EDGE_CURVE('',#13815,#13928,#11549,.T.);
#17158=EDGE_CURVE('',#13928,#13927,#7792,.T.);
#17159=EDGE_CURVE('',#13817,#13929,#11550,.T.);
#17160=EDGE_CURVE('',#13929,#13928,#11551,.T.);
#17161=EDGE_CURVE('',#13819,#13930,#11552,.T.);
#17162=EDGE_CURVE('',#13930,#13929,#11553,.T.);
#17163=EDGE_CURVE('',#13821,#13931,#11554,.T.);
#17164=EDGE_CURVE('',#13931,#13930,#11555,.T.);
#17165=EDGE_CURVE('',#13823,#13932,#11556,.T.);
#17166=EDGE_CURVE('',#13932,#13931,#7793,.T.);
#17167=EDGE_CURVE('',#13825,#13933,#11557,.T.);
#17168=EDGE_CURVE('',#13933,#13932,#11558,.T.);
#17169=EDGE_CURVE('',#13827,#13934,#11559,.T.);
#17170=EDGE_CURVE('',#13934,#13933,#11560,.T.);
#17171=EDGE_CURVE('',#13829,#13935,#11561,.T.);
#17172=EDGE_CURVE('',#13935,#13934,#11562,.T.);
#17173=EDGE_CURVE('',#13831,#13936,#11563,.T.);
#17174=EDGE_CURVE('',#13936,#13935,#7794,.T.);
#17175=EDGE_CURVE('',#13833,#13937,#11564,.T.);
#17176=EDGE_CURVE('',#13937,#13936,#11565,.T.);
#17177=EDGE_CURVE('',#13835,#13938,#11566,.T.);
#17178=EDGE_CURVE('',#13938,#13937,#7795,.T.);
#17179=EDGE_CURVE('',#13902,#13939,#11567,.T.);
#17180=EDGE_CURVE('',#13837,#13939,#11568,.T.);
#17181=EDGE_CURVE('',#13839,#13940,#11569,.T.);
#17182=EDGE_CURVE('',#13940,#13938,#11570,.T.);
#17183=EDGE_CURVE('',#13939,#13940,#7796,.T.);
#17184=EDGE_CURVE('',#13941,#13708,#7797,.T.);
#17185=EDGE_CURVE('',#13942,#13941,#11571,.T.);
#17186=EDGE_CURVE('',#13942,#13943,#7798,.T.);
#17187=EDGE_CURVE('',#13944,#13943,#11572,.T.);
#17188=EDGE_CURVE('',#13944,#13945,#7799,.T.);
#17189=EDGE_CURVE('',#13946,#13945,#11573,.T.);
#17190=EDGE_CURVE('',#13947,#13946,#7800,.T.);
#17191=EDGE_CURVE('',#13948,#13947,#11574,.T.);
#17192=EDGE_CURVE('',#13949,#13948,#7801,.T.);
#17193=EDGE_CURVE('',#13840,#13949,#11575,.T.);
#17194=EDGE_CURVE('',#13950,#13869,#11576,.T.);
#17195=EDGE_CURVE('',#13950,#13951,#7802,.T.);
#17196=EDGE_CURVE('',#13952,#13951,#11577,.T.);
#17197=EDGE_CURVE('',#13952,#13953,#7803,.T.);
#17198=EDGE_CURVE('',#13953,#13954,#11578,.T.);
#17199=EDGE_CURVE('',#13955,#13954,#7804,.T.);
#17200=EDGE_CURVE('',#13956,#13955,#11579,.T.);
#17201=EDGE_CURVE('',#13957,#13956,#7805,.T.);
#17202=EDGE_CURVE('',#13867,#13957,#11580,.T.);
#17203=EDGE_CURVE('',#13954,#13958,#7806,.T.);
#17204=EDGE_CURVE('',#13953,#13959,#7807,.T.);
#17205=EDGE_CURVE('',#13959,#13958,#11581,.T.);
#17206=EDGE_CURVE('',#13960,#13711,#7808,.T.);
#17207=EDGE_CURVE('',#13941,#13960,#7809,.T.);
#17208=EDGE_CURVE('',#13961,#13958,#7810,.T.);
#17209=EDGE_CURVE('',#13955,#13961,#7811,.T.);
#17210=EDGE_CURVE('',#13961,#13962,#11582,.T.);
#17211=EDGE_CURVE('',#13956,#13962,#7812,.T.);
#17212=EDGE_CURVE('',#13963,#13962,#7813,.T.);
#17213=EDGE_CURVE('',#13957,#13963,#7814,.T.);
#17214=EDGE_CURVE('',#13963,#13868,#11583,.T.);
#17215=EDGE_CURVE('',#13942,#13964,#7815,.T.);
#17216=EDGE_CURVE('',#13964,#13965,#7816,.T.);
#17217=EDGE_CURVE('',#13943,#13965,#7817,.T.);
#17218=EDGE_CURVE('',#13960,#13964,#11584,.T.);
#17219=EDGE_CURVE('',#13965,#13966,#11585,.T.);
#17220=EDGE_CURVE('',#13944,#13966,#7818,.T.);
#17221=EDGE_CURVE('',#13966,#13967,#7819,.T.);
#17222=EDGE_CURVE('',#13945,#13967,#7820,.T.);
#17223=EDGE_CURVE('',#13967,#13968,#11586,.T.);
#17224=EDGE_CURVE('',#13946,#13968,#7821,.T.);
#17225=EDGE_CURVE('',#13952,#13969,#7822,.T.);
#17226=EDGE_CURVE('',#13969,#13959,#7823,.T.);
#17227=EDGE_CURVE('',#13970,#13969,#11587,.T.);
#17228=EDGE_CURVE('',#13951,#13970,#7824,.T.);
#17229=EDGE_CURVE('',#13950,#13971,#7825,.T.);
#17230=EDGE_CURVE('',#13971,#13970,#7826,.T.);
#17231=EDGE_CURVE('',#13972,#13841,#11588,.T.);
#17232=EDGE_CURVE('',#13949,#13972,#7827,.T.);
#17233=EDGE_CURVE('',#13948,#13973,#7828,.T.);
#17234=EDGE_CURVE('',#13972,#13973,#7829,.T.);
#17235=EDGE_CURVE('',#13974,#13973,#11589,.T.);
#17236=EDGE_CURVE('',#13947,#13974,#7830,.T.);
#17237=EDGE_CURVE('',#13974,#13968,#7831,.T.);
#17238=EDGE_CURVE('',#13874,#13975,#7832,.T.);
#17239=EDGE_CURVE('',#13976,#13975,#1421,.T.);
#17240=EDGE_CURVE('',#13894,#13976,#7833,.T.);
#17241=EDGE_CURVE('',#13873,#13977,#7834,.T.);
#17242=EDGE_CURVE('',#13977,#13975,#1422,.T.);
#17243=EDGE_CURVE('',#13878,#13978,#7835,.T.);
#17244=EDGE_CURVE('',#13977,#13978,#7836,.T.);
#17245=EDGE_CURVE('',#13880,#13979,#7837,.T.);
#17246=EDGE_CURVE('',#13980,#13979,#1423,.T.);
#17247=EDGE_CURVE('',#13877,#13980,#7838,.T.);
#17248=EDGE_CURVE('',#13980,#13978,#1424,.T.);
#17249=EDGE_CURVE('',#13879,#13981,#7839,.T.);
#17250=EDGE_CURVE('',#13979,#13981,#1425,.T.);
#17251=EDGE_CURVE('',#13881,#13982,#7840,.T.);
#17252=EDGE_CURVE('',#13981,#13982,#1426,.T.);
#17253=EDGE_CURVE('',#13883,#13983,#7841,.T.);
#17254=EDGE_CURVE('',#13982,#13983,#1427,.T.);
#17255=EDGE_CURVE('',#13885,#13984,#7842,.T.);
#17256=EDGE_CURVE('',#13984,#13983,#1428,.T.);
#17257=EDGE_CURVE('',#13886,#13985,#7843,.T.);
#17258=EDGE_CURVE('',#13984,#13985,#11590,.T.);
#17259=EDGE_CURVE('',#13985,#13890,#1429,.T.);
#17260=EDGE_CURVE('',#13870,#13971,#11591,.T.);
#17261=EDGE_CURVE('',#13976,#13893,#11592,.T.);
#17262=EDGE_CURVE('',#13858,#13986,#1430,.T.);
#17263=EDGE_CURVE('',#13896,#13986,#7844,.T.);
#17264=EDGE_CURVE('',#13849,#13986,#1431,.T.);
#17265=EDGE_CURVE('',#13987,#13988,#1432,.T.);
#17266=EDGE_CURVE('',#13987,#13989,#11593,.T.);
#17267=EDGE_CURVE('',#13989,#13990,#1433,.T.);
#17268=EDGE_CURVE('',#13990,#13988,#1434,.T.);
#17269=EDGE_CURVE('',#13991,#13992,#11594,.T.);
#17270=EDGE_CURVE('',#13992,#13989,#1435,.T.);
#17271=EDGE_CURVE('',#13991,#13987,#1436,.T.);
#17272=EDGE_CURVE('',#13993,#13994,#11595,.T.);
#17273=EDGE_CURVE('',#13994,#13992,#1437,.T.);
#17274=EDGE_CURVE('',#13993,#13991,#1438,.T.);
#17275=EDGE_CURVE('',#13707,#13994,#1439,.T.);
#17276=EDGE_CURVE('',#13633,#13993,#467,.T.);
#17277=EDGE_CURVE('',#13689,#13988,#7845,.T.);
#17278=EDGE_CURVE('',#13995,#13988,#1440,.T.);
#17279=EDGE_CURVE('',#13996,#13995,#1441,.T.);
#17280=EDGE_CURVE('',#13997,#13996,#1442,.T.);
#17281=EDGE_CURVE('',#13998,#13997,#468,.T.);
#17282=EDGE_CURVE('',#13998,#13690,#7846,.T.);
#17283=EDGE_CURVE('',#13999,#13998,#11596,.T.);
#17284=EDGE_CURVE('',#13999,#13691,#7847,.T.);
#17285=EDGE_CURVE('',#14000,#13999,#469,.T.);
#17286=EDGE_CURVE('',#14001,#14000,#1443,.T.);
#17287=EDGE_CURVE('',#13685,#14001,#7848,.T.);
#17288=EDGE_CURVE('',#14002,#14001,#470,.T.);
#17289=EDGE_CURVE('',#14003,#14002,#1444,.T.);
#17290=EDGE_CURVE('',#13686,#14003,#7849,.T.);
#17291=EDGE_CURVE('',#14004,#14003,#471,.T.);
#17292=EDGE_CURVE('',#14005,#14004,#1445,.T.);
#17293=EDGE_CURVE('',#14005,#14006,#1446,.T.);
#17294=EDGE_CURVE('',#14006,#14007,#472,.T.);
#17295=EDGE_CURVE('',#13687,#14007,#7850,.T.);
#17296=EDGE_CURVE('',#14007,#14008,#1447,.T.);
#17297=EDGE_CURVE('',#14008,#14009,#473,.T.);
#17298=EDGE_CURVE('',#13688,#14009,#7851,.T.);
#17299=EDGE_CURVE('',#14009,#14010,#1448,.T.);
#17300=EDGE_CURVE('',#14010,#13631,#474,.T.);
#17301=EDGE_CURVE('',#14010,#14011,#11597,.T.);
#17302=EDGE_CURVE('',#14011,#13707,#1449,.T.);
#17303=EDGE_CURVE('',#14009,#14012,#475,.T.);
#17304=EDGE_CURVE('',#14012,#14011,#1450,.T.);
#17305=EDGE_CURVE('',#14008,#14013,#476,.T.);
#17306=EDGE_CURVE('',#14013,#14012,#477,.T.);
#17307=EDGE_CURVE('',#14007,#14014,#11598,.T.);
#17308=EDGE_CURVE('',#14014,#14013,#1451,.T.);
#17309=EDGE_CURVE('',#14006,#14015,#11599,.T.);
#17310=EDGE_CURVE('',#14015,#14014,#1452,.T.);
#17311=EDGE_CURVE('',#14016,#14015,#1453,.T.);
#17312=EDGE_CURVE('',#14005,#14016,#11600,.T.);
#17313=EDGE_CURVE('',#14004,#14017,#11601,.T.);
#17314=EDGE_CURVE('',#14016,#14017,#1454,.T.);
#17315=EDGE_CURVE('',#14003,#14018,#11602,.T.);
#17316=EDGE_CURVE('',#14017,#14018,#1455,.T.);
#17317=EDGE_CURVE('',#14002,#14019,#478,.T.);
#17318=EDGE_CURVE('',#14018,#14019,#1456,.T.);
#17319=EDGE_CURVE('',#14001,#14020,#479,.T.);
#17320=EDGE_CURVE('',#14019,#14020,#480,.T.);
#17321=EDGE_CURVE('',#14000,#14021,#11603,.T.);
#17322=EDGE_CURVE('',#14020,#14021,#1457,.T.);
#17323=EDGE_CURVE('',#13999,#14022,#11604,.T.);
#17324=EDGE_CURVE('',#14021,#14022,#1458,.T.);
#17325=EDGE_CURVE('',#13998,#14022,#11605,.T.);
#17326=EDGE_CURVE('',#13997,#14023,#11606,.T.);
#17327=EDGE_CURVE('',#14022,#14023,#1459,.T.);
#17328=EDGE_CURVE('',#13996,#14024,#11607,.T.);
#17329=EDGE_CURVE('',#14023,#14024,#1460,.T.);
#17330=EDGE_CURVE('',#13995,#14025,#11608,.T.);
#17331=EDGE_CURVE('',#14024,#14025,#1461,.T.);
#17332=EDGE_CURVE('',#14025,#13990,#1462,.T.);
#17333=EDGE_CURVE('',#13990,#14026,#1463,.T.);
#17334=EDGE_CURVE('',#14026,#14027,#1464,.T.);
#17335=EDGE_CURVE('',#14027,#14028,#1465,.T.);
#17336=EDGE_CURVE('',#14025,#14028,#7852,.T.);
#17337=EDGE_CURVE('',#13989,#14029,#7853,.T.);
#17338=EDGE_CURVE('',#14027,#14029,#1466,.T.);
#17339=EDGE_CURVE('',#13992,#14030,#7854,.T.);
#17340=EDGE_CURVE('',#14029,#14030,#11609,.T.);
#17341=EDGE_CURVE('',#13994,#14031,#7855,.T.);
#17342=EDGE_CURVE('',#14030,#14031,#11610,.T.);
#17343=EDGE_CURVE('',#14011,#14032,#7856,.T.);
#17344=EDGE_CURVE('',#14032,#14031,#11611,.T.);
#17345=EDGE_CURVE('',#14013,#14033,#7857,.T.);
#17346=EDGE_CURVE('',#14033,#14032,#1467,.T.);
#17347=EDGE_CURVE('',#14015,#14034,#7858,.T.);
#17348=EDGE_CURVE('',#14033,#14034,#481,.T.);
#17349=EDGE_CURVE('',#14016,#14035,#7859,.T.);
#17350=EDGE_CURVE('',#14034,#14035,#11612,.T.);
#17351=EDGE_CURVE('',#14017,#14036,#7860,.T.);
#17352=EDGE_CURVE('',#14036,#14035,#11613,.T.);
#17353=EDGE_CURVE('',#14019,#14037,#7861,.T.);
#17354=EDGE_CURVE('',#14037,#14036,#482,.T.);
#17355=EDGE_CURVE('',#14021,#14038,#7862,.T.);
#17356=EDGE_CURVE('',#14037,#14038,#1468,.T.);
#17357=EDGE_CURVE('',#14023,#14039,#7863,.T.);
#17358=EDGE_CURVE('',#14038,#14039,#11614,.T.);
#17359=EDGE_CURVE('',#14024,#14040,#7864,.T.);
#17360=EDGE_CURVE('',#14040,#14039,#11615,.T.);
#17361=EDGE_CURVE('',#14028,#14040,#11616,.T.);
#17362=EDGE_CURVE('',#14041,#14042,#11617,.T.);
#17363=EDGE_CURVE('',#14043,#14041,#11618,.T.);
#17364=EDGE_CURVE('',#14044,#14043,#11619,.T.);
#17365=EDGE_CURVE('',#14045,#14044,#11620,.T.);
#17366=EDGE_CURVE('',#14045,#14046,#11621,.T.);
#17367=EDGE_CURVE('',#14046,#14047,#11622,.T.);
#17368=EDGE_CURVE('',#14047,#14042,#11623,.T.);
#17369=EDGE_CURVE('',#14048,#14049,#11624,.T.);
#17370=EDGE_CURVE('',#14043,#14048,#7865,.T.);
#17371=EDGE_CURVE('',#14041,#14049,#7866,.T.);
#17372=EDGE_CURVE('',#14044,#14050,#7867,.T.);
#17373=EDGE_CURVE('',#14050,#14048,#11625,.T.);
#17374=EDGE_CURVE('',#14045,#14051,#7868,.T.);
#17375=EDGE_CURVE('',#14051,#14050,#11626,.T.);
#17376=EDGE_CURVE('',#14051,#14052,#11627,.T.);
#17377=EDGE_CURVE('',#14046,#14052,#7869,.T.);
#17378=EDGE_CURVE('',#14052,#14053,#11628,.T.);
#17379=EDGE_CURVE('',#14047,#14053,#7870,.T.);
#17380=EDGE_CURVE('',#14053,#14054,#11629,.T.);
#17381=EDGE_CURVE('',#14042,#14054,#7871,.T.);
#17382=EDGE_CURVE('',#14054,#14049,#11630,.T.);
#21801=ORIENTED_EDGE('',*,*,#16672,.F.);
#21802=ORIENTED_EDGE('',*,*,#16673,.T.);
#21803=ORIENTED_EDGE('',*,*,#16674,.T.);
#21804=ORIENTED_EDGE('',*,*,#16675,.F.);
#21805=ORIENTED_EDGE('',*,*,#16676,.T.);
#21806=ORIENTED_EDGE('',*,*,#16677,.T.);
#21807=ORIENTED_EDGE('',*,*,#16678,.T.);
#21808=ORIENTED_EDGE('',*,*,#16679,.T.);
#21809=ORIENTED_EDGE('',*,*,#16680,.T.);
#21810=ORIENTED_EDGE('',*,*,#16681,.T.);
#21811=ORIENTED_EDGE('',*,*,#16682,.T.);
#21812=ORIENTED_EDGE('',*,*,#16683,.T.);
#21813=ORIENTED_EDGE('',*,*,#16684,.T.);
#21814=ORIENTED_EDGE('',*,*,#16685,.T.);
#21815=ORIENTED_EDGE('',*,*,#16686,.T.);
#21816=ORIENTED_EDGE('',*,*,#16687,.T.);
#21817=ORIENTED_EDGE('',*,*,#16688,.T.);
#21818=ORIENTED_EDGE('',*,*,#16689,.T.);
#21819=ORIENTED_EDGE('',*,*,#16690,.T.);
#21820=ORIENTED_EDGE('',*,*,#16691,.T.);
#21821=ORIENTED_EDGE('',*,*,#16692,.T.);
#21822=ORIENTED_EDGE('',*,*,#16693,.T.);
#21823=ORIENTED_EDGE('',*,*,#16694,.T.);
#21824=ORIENTED_EDGE('',*,*,#16695,.T.);
#21825=ORIENTED_EDGE('',*,*,#16696,.T.);
#21826=ORIENTED_EDGE('',*,*,#16697,.T.);
#21827=ORIENTED_EDGE('',*,*,#16698,.T.);
#21828=ORIENTED_EDGE('',*,*,#16699,.T.);
#21829=ORIENTED_EDGE('',*,*,#16700,.T.);
#21830=ORIENTED_EDGE('',*,*,#16701,.T.);
#21831=ORIENTED_EDGE('',*,*,#16702,.T.);
#21832=ORIENTED_EDGE('',*,*,#16703,.T.);
#21833=ORIENTED_EDGE('',*,*,#16704,.T.);
#21834=ORIENTED_EDGE('',*,*,#16705,.T.);
#21835=ORIENTED_EDGE('',*,*,#16706,.T.);
#21836=ORIENTED_EDGE('',*,*,#16707,.T.);
#21837=ORIENTED_EDGE('',*,*,#16708,.T.);
#21838=ORIENTED_EDGE('',*,*,#16709,.T.);
#21839=ORIENTED_EDGE('',*,*,#16710,.T.);
#21840=ORIENTED_EDGE('',*,*,#16711,.T.);
#21841=ORIENTED_EDGE('',*,*,#16712,.T.);
#21842=ORIENTED_EDGE('',*,*,#16713,.T.);
#21843=ORIENTED_EDGE('',*,*,#16714,.T.);
#21844=ORIENTED_EDGE('',*,*,#16715,.T.);
#21845=ORIENTED_EDGE('',*,*,#16716,.T.);
#21846=ORIENTED_EDGE('',*,*,#16717,.F.);
#21847=ORIENTED_EDGE('',*,*,#16718,.F.);
#21848=ORIENTED_EDGE('',*,*,#16719,.F.);
#21849=ORIENTED_EDGE('',*,*,#16720,.T.);
#21850=ORIENTED_EDGE('',*,*,#16721,.F.);
#21851=ORIENTED_EDGE('',*,*,#16722,.T.);
#21852=ORIENTED_EDGE('',*,*,#16723,.F.);
#21853=ORIENTED_EDGE('',*,*,#16724,.T.);
#21854=ORIENTED_EDGE('',*,*,#16725,.F.);
#21855=ORIENTED_EDGE('',*,*,#16726,.T.);
#21856=ORIENTED_EDGE('',*,*,#16727,.F.);
#21857=ORIENTED_EDGE('',*,*,#16728,.F.);
#21858=ORIENTED_EDGE('',*,*,#16729,.T.);
#21859=ORIENTED_EDGE('',*,*,#16675,.T.);
#21860=ORIENTED_EDGE('',*,*,#16730,.F.);
#21861=ORIENTED_EDGE('',*,*,#16731,.T.);
#21862=ORIENTED_EDGE('',*,*,#16732,.F.);
#21863=ORIENTED_EDGE('',*,*,#16733,.F.);
#21864=ORIENTED_EDGE('',*,*,#16734,.T.);
#21865=ORIENTED_EDGE('',*,*,#16735,.F.);
#21866=ORIENTED_EDGE('',*,*,#16736,.T.);
#21867=ORIENTED_EDGE('',*,*,#16737,.F.);
#21868=ORIENTED_EDGE('',*,*,#16738,.T.);
#21869=ORIENTED_EDGE('',*,*,#16739,.T.);
#21870=ORIENTED_EDGE('',*,*,#16740,.T.);
#21871=ORIENTED_EDGE('',*,*,#16741,.F.);
#21872=ORIENTED_EDGE('',*,*,#16742,.T.);
#21873=ORIENTED_EDGE('',*,*,#16743,.F.);
#21874=ORIENTED_EDGE('',*,*,#16744,.T.);
#21875=ORIENTED_EDGE('',*,*,#16745,.T.);
#21876=ORIENTED_EDGE('',*,*,#16746,.F.);
#21877=ORIENTED_EDGE('',*,*,#16747,.F.);
#21878=ORIENTED_EDGE('',*,*,#16748,.F.);
#21879=ORIENTED_EDGE('',*,*,#16749,.T.);
#21880=ORIENTED_EDGE('',*,*,#16750,.F.);
#21881=ORIENTED_EDGE('',*,*,#16673,.F.);
#21882=ORIENTED_EDGE('',*,*,#16751,.T.);
#21883=ORIENTED_EDGE('',*,*,#16752,.T.);
#21884=ORIENTED_EDGE('',*,*,#16753,.F.);
#21885=ORIENTED_EDGE('',*,*,#16754,.F.);
#21886=ORIENTED_EDGE('',*,*,#16755,.T.);
#21887=ORIENTED_EDGE('',*,*,#16756,.F.);
#21888=ORIENTED_EDGE('',*,*,#16757,.F.);
#21889=ORIENTED_EDGE('',*,*,#16725,.T.);
#21890=ORIENTED_EDGE('',*,*,#16758,.T.);
#21891=ORIENTED_EDGE('',*,*,#16759,.F.);
#21892=ORIENTED_EDGE('',*,*,#16760,.F.);
#21893=ORIENTED_EDGE('',*,*,#16755,.F.);
#21894=ORIENTED_EDGE('',*,*,#16724,.F.);
#21895=ORIENTED_EDGE('',*,*,#16761,.T.);
#21896=ORIENTED_EDGE('',*,*,#16762,.F.);
#21897=ORIENTED_EDGE('',*,*,#16758,.F.);
#21898=ORIENTED_EDGE('',*,*,#16723,.T.);
#21899=ORIENTED_EDGE('',*,*,#16763,.T.);
#21900=ORIENTED_EDGE('',*,*,#16764,.F.);
#21901=ORIENTED_EDGE('',*,*,#16765,.F.);
#21902=ORIENTED_EDGE('',*,*,#16766,.F.);
#21903=ORIENTED_EDGE('',*,*,#16761,.F.);
#21904=ORIENTED_EDGE('',*,*,#16722,.F.);
#21905=ORIENTED_EDGE('',*,*,#16767,.T.);
#21906=ORIENTED_EDGE('',*,*,#16768,.F.);
#21907=ORIENTED_EDGE('',*,*,#16769,.F.);
#21908=ORIENTED_EDGE('',*,*,#16770,.F.);
#21909=ORIENTED_EDGE('',*,*,#16771,.F.);
#21910=ORIENTED_EDGE('',*,*,#16763,.F.);
#21911=ORIENTED_EDGE('',*,*,#16721,.T.);
#21912=ORIENTED_EDGE('',*,*,#16720,.F.);
#21913=ORIENTED_EDGE('',*,*,#16772,.T.);
#21914=ORIENTED_EDGE('',*,*,#16773,.F.);
#21915=ORIENTED_EDGE('',*,*,#16774,.F.);
#21916=ORIENTED_EDGE('',*,*,#16767,.F.);
#21917=ORIENTED_EDGE('',*,*,#16775,.T.);
#21918=ORIENTED_EDGE('',*,*,#16776,.F.);
#21919=ORIENTED_EDGE('',*,*,#16777,.F.);
#21920=ORIENTED_EDGE('',*,*,#16778,.F.);
#21921=ORIENTED_EDGE('',*,*,#16779,.F.);
#21922=ORIENTED_EDGE('',*,*,#16772,.F.);
#21923=ORIENTED_EDGE('',*,*,#16719,.T.);
#21924=ORIENTED_EDGE('',*,*,#16780,.T.);
#21925=ORIENTED_EDGE('',*,*,#16781,.T.);
#21926=ORIENTED_EDGE('',*,*,#16782,.F.);
#21927=ORIENTED_EDGE('',*,*,#16775,.F.);
#21928=ORIENTED_EDGE('',*,*,#16718,.T.);
#21929=ORIENTED_EDGE('',*,*,#16783,.T.);
#21930=ORIENTED_EDGE('',*,*,#16784,.F.);
#21931=ORIENTED_EDGE('',*,*,#16785,.T.);
#21932=ORIENTED_EDGE('',*,*,#16780,.F.);
#21933=ORIENTED_EDGE('',*,*,#16717,.T.);
#21934=ORIENTED_EDGE('',*,*,#16757,.T.);
#21935=ORIENTED_EDGE('',*,*,#16786,.F.);
#21936=ORIENTED_EDGE('',*,*,#16787,.F.);
#21937=ORIENTED_EDGE('',*,*,#16788,.F.);
#21938=ORIENTED_EDGE('',*,*,#16783,.F.);
#21939=ORIENTED_EDGE('',*,*,#16716,.F.);
#21940=ORIENTED_EDGE('',*,*,#16743,.T.);
#21941=ORIENTED_EDGE('',*,*,#16789,.T.);
#21942=ORIENTED_EDGE('',*,*,#16790,.T.);
#21943=ORIENTED_EDGE('',*,*,#16791,.T.);
#21944=ORIENTED_EDGE('',*,*,#16792,.F.);
#21945=ORIENTED_EDGE('',*,*,#16742,.F.);
#21946=ORIENTED_EDGE('',*,*,#16793,.T.);
#21947=ORIENTED_EDGE('',*,*,#16794,.T.);
#21948=ORIENTED_EDGE('',*,*,#16789,.F.);
#21949=ORIENTED_EDGE('',*,*,#16741,.T.);
#21950=ORIENTED_EDGE('',*,*,#16795,.T.);
#21951=ORIENTED_EDGE('',*,*,#16796,.T.);
#21952=ORIENTED_EDGE('',*,*,#16797,.T.);
#21953=ORIENTED_EDGE('',*,*,#16798,.T.);
#21954=ORIENTED_EDGE('',*,*,#16793,.F.);
#21955=ORIENTED_EDGE('',*,*,#16740,.F.);
#21956=ORIENTED_EDGE('',*,*,#16799,.T.);
#21957=ORIENTED_EDGE('',*,*,#16800,.F.);
#21958=ORIENTED_EDGE('',*,*,#16801,.T.);
#21959=ORIENTED_EDGE('',*,*,#16795,.F.);
#21960=ORIENTED_EDGE('',*,*,#16739,.F.);
#21961=ORIENTED_EDGE('',*,*,#16802,.T.);
#21962=ORIENTED_EDGE('',*,*,#16803,.T.);
#21963=ORIENTED_EDGE('',*,*,#16804,.F.);
#21964=ORIENTED_EDGE('',*,*,#16799,.F.);
#21965=ORIENTED_EDGE('',*,*,#16738,.F.);
#21966=ORIENTED_EDGE('',*,*,#16805,.T.);
#21967=ORIENTED_EDGE('',*,*,#16806,.T.);
#21968=ORIENTED_EDGE('',*,*,#16807,.T.);
#21969=ORIENTED_EDGE('',*,*,#16808,.T.);
#21970=ORIENTED_EDGE('',*,*,#16809,.T.);
#21971=ORIENTED_EDGE('',*,*,#16802,.F.);
#21972=ORIENTED_EDGE('',*,*,#16810,.T.);
#21973=ORIENTED_EDGE('',*,*,#16811,.T.);
#21974=ORIENTED_EDGE('',*,*,#16812,.T.);
#21975=ORIENTED_EDGE('',*,*,#16805,.F.);
#21976=ORIENTED_EDGE('',*,*,#16737,.T.);
#21977=ORIENTED_EDGE('',*,*,#16736,.F.);
#21978=ORIENTED_EDGE('',*,*,#16813,.T.);
#21979=ORIENTED_EDGE('',*,*,#16814,.T.);
#21980=ORIENTED_EDGE('',*,*,#16815,.T.);
#21981=ORIENTED_EDGE('',*,*,#16816,.T.);
#21982=ORIENTED_EDGE('',*,*,#16817,.T.);
#21983=ORIENTED_EDGE('',*,*,#16810,.F.);
#21984=ORIENTED_EDGE('',*,*,#16735,.T.);
#21985=ORIENTED_EDGE('',*,*,#16818,.T.);
#21986=ORIENTED_EDGE('',*,*,#16819,.T.);
#21987=ORIENTED_EDGE('',*,*,#16820,.T.);
#21988=ORIENTED_EDGE('',*,*,#16821,.T.);
#21989=ORIENTED_EDGE('',*,*,#16813,.F.);
#21990=ORIENTED_EDGE('',*,*,#16734,.F.);
#21991=ORIENTED_EDGE('',*,*,#16792,.T.);
#21992=ORIENTED_EDGE('',*,*,#16822,.T.);
#21993=ORIENTED_EDGE('',*,*,#16818,.F.);
#21994=ORIENTED_EDGE('',*,*,#16823,.T.);
#21995=ORIENTED_EDGE('',*,*,#16824,.T.);
#21996=ORIENTED_EDGE('',*,*,#16825,.F.);
#21997=ORIENTED_EDGE('',*,*,#16826,.F.);
#21998=ORIENTED_EDGE('',*,*,#16827,.T.);
#21999=ORIENTED_EDGE('',*,*,#16825,.T.);
#22000=ORIENTED_EDGE('',*,*,#16828,.F.);
#22001=ORIENTED_EDGE('',*,*,#16706,.F.);
#22002=ORIENTED_EDGE('',*,*,#16829,.T.);
#22003=ORIENTED_EDGE('',*,*,#16830,.T.);
#22004=ORIENTED_EDGE('',*,*,#16827,.F.);
#22005=ORIENTED_EDGE('',*,*,#16705,.F.);
#22006=ORIENTED_EDGE('',*,*,#16831,.F.);
#22007=ORIENTED_EDGE('',*,*,#16832,.T.);
#22008=ORIENTED_EDGE('',*,*,#16826,.T.);
#22009=ORIENTED_EDGE('',*,*,#16830,.F.);
#22010=ORIENTED_EDGE('',*,*,#16833,.T.);
#22011=ORIENTED_EDGE('',*,*,#16834,.T.);
#22012=ORIENTED_EDGE('',*,*,#16829,.F.);
#22013=ORIENTED_EDGE('',*,*,#16704,.F.);
#22014=ORIENTED_EDGE('',*,*,#16835,.T.);
#22015=ORIENTED_EDGE('',*,*,#16836,.T.);
#22016=ORIENTED_EDGE('',*,*,#16831,.T.);
#22017=ORIENTED_EDGE('',*,*,#16834,.F.);
#22018=ORIENTED_EDGE('',*,*,#16837,.T.);
#22019=ORIENTED_EDGE('',*,*,#16838,.T.);
#22020=ORIENTED_EDGE('',*,*,#16833,.F.);
#22021=ORIENTED_EDGE('',*,*,#16703,.F.);
#22022=ORIENTED_EDGE('',*,*,#16838,.F.);
#22023=ORIENTED_EDGE('',*,*,#16839,.T.);
#22024=ORIENTED_EDGE('',*,*,#16840,.T.);
#22025=ORIENTED_EDGE('',*,*,#16835,.F.);
#22026=ORIENTED_EDGE('',*,*,#16841,.T.);
#22027=ORIENTED_EDGE('',*,*,#16842,.T.);
#22028=ORIENTED_EDGE('',*,*,#16837,.F.);
#22029=ORIENTED_EDGE('',*,*,#16702,.F.);
#22030=ORIENTED_EDGE('',*,*,#16843,.T.);
#22031=ORIENTED_EDGE('',*,*,#16844,.T.);
#22032=ORIENTED_EDGE('',*,*,#16839,.F.);
#22033=ORIENTED_EDGE('',*,*,#16842,.F.);
#22034=ORIENTED_EDGE('',*,*,#16845,.T.);
#22035=ORIENTED_EDGE('',*,*,#16846,.T.);
#22036=ORIENTED_EDGE('',*,*,#16841,.F.);
#22037=ORIENTED_EDGE('',*,*,#16701,.F.);
#22038=ORIENTED_EDGE('',*,*,#16846,.F.);
#22039=ORIENTED_EDGE('',*,*,#16847,.T.);
#22040=ORIENTED_EDGE('',*,*,#16848,.T.);
#22041=ORIENTED_EDGE('',*,*,#16843,.F.);
#22042=ORIENTED_EDGE('',*,*,#16849,.T.);
#22043=ORIENTED_EDGE('',*,*,#16850,.T.);
#22044=ORIENTED_EDGE('',*,*,#16845,.F.);
#22045=ORIENTED_EDGE('',*,*,#16700,.F.);
#22046=ORIENTED_EDGE('',*,*,#16850,.F.);
#22047=ORIENTED_EDGE('',*,*,#16851,.F.);
#22048=ORIENTED_EDGE('',*,*,#16852,.T.);
#22049=ORIENTED_EDGE('',*,*,#16847,.F.);
#22050=ORIENTED_EDGE('',*,*,#16853,.T.);
#22051=ORIENTED_EDGE('',*,*,#16854,.T.);
#22052=ORIENTED_EDGE('',*,*,#16849,.F.);
#22053=ORIENTED_EDGE('',*,*,#16699,.F.);
#22054=ORIENTED_EDGE('',*,*,#16855,.F.);
#22055=ORIENTED_EDGE('',*,*,#16856,.T.);
#22056=ORIENTED_EDGE('',*,*,#16851,.T.);
#22057=ORIENTED_EDGE('',*,*,#16854,.F.);
#22058=ORIENTED_EDGE('',*,*,#16857,.T.);
#22059=ORIENTED_EDGE('',*,*,#16858,.T.);
#22060=ORIENTED_EDGE('',*,*,#16853,.F.);
#22061=ORIENTED_EDGE('',*,*,#16698,.F.);
#22062=ORIENTED_EDGE('',*,*,#16859,.F.);
#22063=ORIENTED_EDGE('',*,*,#16860,.T.);
#22064=ORIENTED_EDGE('',*,*,#16855,.T.);
#22065=ORIENTED_EDGE('',*,*,#16858,.F.);
#22066=ORIENTED_EDGE('',*,*,#16861,.T.);
#22067=ORIENTED_EDGE('',*,*,#16862,.T.);
#22068=ORIENTED_EDGE('',*,*,#16857,.F.);
#22069=ORIENTED_EDGE('',*,*,#16697,.F.);
#22070=ORIENTED_EDGE('',*,*,#16863,.F.);
#22071=ORIENTED_EDGE('',*,*,#16864,.T.);
#22072=ORIENTED_EDGE('',*,*,#16859,.T.);
#22073=ORIENTED_EDGE('',*,*,#16862,.F.);
#22074=ORIENTED_EDGE('',*,*,#16865,.T.);
#22075=ORIENTED_EDGE('',*,*,#16866,.T.);
#22076=ORIENTED_EDGE('',*,*,#16861,.F.);
#22077=ORIENTED_EDGE('',*,*,#16696,.F.);
#22078=ORIENTED_EDGE('',*,*,#16866,.F.);
#22079=ORIENTED_EDGE('',*,*,#16867,.F.);
#22080=ORIENTED_EDGE('',*,*,#16868,.T.);
#22081=ORIENTED_EDGE('',*,*,#16863,.T.);
#22082=ORIENTED_EDGE('',*,*,#16869,.T.);
#22083=ORIENTED_EDGE('',*,*,#16870,.T.);
#22084=ORIENTED_EDGE('',*,*,#16865,.F.);
#22085=ORIENTED_EDGE('',*,*,#16695,.F.);
#22086=ORIENTED_EDGE('',*,*,#16871,.F.);
#22087=ORIENTED_EDGE('',*,*,#16872,.T.);
#22088=ORIENTED_EDGE('',*,*,#16867,.T.);
#22089=ORIENTED_EDGE('',*,*,#16870,.F.);
#22090=ORIENTED_EDGE('',*,*,#16873,.T.);
#22091=ORIENTED_EDGE('',*,*,#16874,.T.);
#22092=ORIENTED_EDGE('',*,*,#16869,.F.);
#22093=ORIENTED_EDGE('',*,*,#16694,.F.);
#22094=ORIENTED_EDGE('',*,*,#16875,.F.);
#22095=ORIENTED_EDGE('',*,*,#16876,.T.);
#22096=ORIENTED_EDGE('',*,*,#16871,.T.);
#22097=ORIENTED_EDGE('',*,*,#16874,.F.);
#22098=ORIENTED_EDGE('',*,*,#16877,.T.);
#22099=ORIENTED_EDGE('',*,*,#16878,.T.);
#22100=ORIENTED_EDGE('',*,*,#16873,.F.);
#22101=ORIENTED_EDGE('',*,*,#16693,.F.);
#22102=ORIENTED_EDGE('',*,*,#16879,.F.);
#22103=ORIENTED_EDGE('',*,*,#16880,.T.);
#22104=ORIENTED_EDGE('',*,*,#16875,.T.);
#22105=ORIENTED_EDGE('',*,*,#16878,.F.);
#22106=ORIENTED_EDGE('',*,*,#16881,.T.);
#22107=ORIENTED_EDGE('',*,*,#16882,.T.);
#22108=ORIENTED_EDGE('',*,*,#16877,.F.);
#22109=ORIENTED_EDGE('',*,*,#16692,.F.);
#22110=ORIENTED_EDGE('',*,*,#16883,.T.);
#22111=ORIENTED_EDGE('',*,*,#16884,.T.);
#22112=ORIENTED_EDGE('',*,*,#16879,.T.);
#22113=ORIENTED_EDGE('',*,*,#16882,.F.);
#22114=ORIENTED_EDGE('',*,*,#16885,.T.);
#22115=ORIENTED_EDGE('',*,*,#16886,.T.);
#22116=ORIENTED_EDGE('',*,*,#16881,.F.);
#22117=ORIENTED_EDGE('',*,*,#16691,.F.);
#22118=ORIENTED_EDGE('',*,*,#16886,.F.);
#22119=ORIENTED_EDGE('',*,*,#16887,.T.);
#22120=ORIENTED_EDGE('',*,*,#16888,.T.);
#22121=ORIENTED_EDGE('',*,*,#16883,.F.);
#22122=ORIENTED_EDGE('',*,*,#16889,.T.);
#22123=ORIENTED_EDGE('',*,*,#16890,.T.);
#22124=ORIENTED_EDGE('',*,*,#16885,.F.);
#22125=ORIENTED_EDGE('',*,*,#16690,.F.);
#22126=ORIENTED_EDGE('',*,*,#16890,.F.);
#22127=ORIENTED_EDGE('',*,*,#16891,.T.);
#22128=ORIENTED_EDGE('',*,*,#16892,.T.);
#22129=ORIENTED_EDGE('',*,*,#16887,.F.);
#22130=ORIENTED_EDGE('',*,*,#16893,.T.);
#22131=ORIENTED_EDGE('',*,*,#16894,.T.);
#22132=ORIENTED_EDGE('',*,*,#16889,.F.);
#22133=ORIENTED_EDGE('',*,*,#16689,.F.);
#22134=ORIENTED_EDGE('',*,*,#16894,.F.);
#22135=ORIENTED_EDGE('',*,*,#16895,.T.);
#22136=ORIENTED_EDGE('',*,*,#16896,.T.);
#22137=ORIENTED_EDGE('',*,*,#16891,.F.);
#22138=ORIENTED_EDGE('',*,*,#16897,.T.);
#22139=ORIENTED_EDGE('',*,*,#16898,.T.);
#22140=ORIENTED_EDGE('',*,*,#16893,.F.);
#22141=ORIENTED_EDGE('',*,*,#16688,.F.);
#22142=ORIENTED_EDGE('',*,*,#16898,.F.);
#22143=ORIENTED_EDGE('',*,*,#16899,.F.);
#22144=ORIENTED_EDGE('',*,*,#16900,.T.);
#22145=ORIENTED_EDGE('',*,*,#16895,.F.);
#22146=ORIENTED_EDGE('',*,*,#16901,.T.);
#22147=ORIENTED_EDGE('',*,*,#16902,.T.);
#22148=ORIENTED_EDGE('',*,*,#16897,.F.);
#22149=ORIENTED_EDGE('',*,*,#16687,.F.);
#22150=ORIENTED_EDGE('',*,*,#16903,.F.);
#22151=ORIENTED_EDGE('',*,*,#16904,.T.);
#22152=ORIENTED_EDGE('',*,*,#16899,.T.);
#22153=ORIENTED_EDGE('',*,*,#16902,.F.);
#22154=ORIENTED_EDGE('',*,*,#16905,.T.);
#22155=ORIENTED_EDGE('',*,*,#16903,.T.);
#22156=ORIENTED_EDGE('',*,*,#16906,.F.);
#22157=ORIENTED_EDGE('',*,*,#16907,.F.);
#22158=ORIENTED_EDGE('',*,*,#16908,.T.);
#22159=ORIENTED_EDGE('',*,*,#16906,.T.);
#22160=ORIENTED_EDGE('',*,*,#16901,.F.);
#22161=ORIENTED_EDGE('',*,*,#16686,.F.);
#22162=ORIENTED_EDGE('',*,*,#16909,.T.);
#22163=ORIENTED_EDGE('',*,*,#16910,.T.);
#22164=ORIENTED_EDGE('',*,*,#16908,.F.);
#22165=ORIENTED_EDGE('',*,*,#16685,.F.);
#22166=ORIENTED_EDGE('',*,*,#16911,.F.);
#22167=ORIENTED_EDGE('',*,*,#16912,.T.);
#22168=ORIENTED_EDGE('',*,*,#16907,.T.);
#22169=ORIENTED_EDGE('',*,*,#16910,.F.);
#22170=ORIENTED_EDGE('',*,*,#16913,.T.);
#22171=ORIENTED_EDGE('',*,*,#16914,.T.);
#22172=ORIENTED_EDGE('',*,*,#16909,.F.);
#22173=ORIENTED_EDGE('',*,*,#16684,.F.);
#22174=ORIENTED_EDGE('',*,*,#16915,.T.);
#22175=ORIENTED_EDGE('',*,*,#16916,.T.);
#22176=ORIENTED_EDGE('',*,*,#16911,.T.);
#22177=ORIENTED_EDGE('',*,*,#16914,.F.);
#22178=ORIENTED_EDGE('',*,*,#16917,.T.);
#22179=ORIENTED_EDGE('',*,*,#16918,.T.);
#22180=ORIENTED_EDGE('',*,*,#16913,.F.);
#22181=ORIENTED_EDGE('',*,*,#16683,.F.);
#22182=ORIENTED_EDGE('',*,*,#16918,.F.);
#22183=ORIENTED_EDGE('',*,*,#16919,.T.);
#22184=ORIENTED_EDGE('',*,*,#16920,.T.);
#22185=ORIENTED_EDGE('',*,*,#16915,.F.);
#22186=ORIENTED_EDGE('',*,*,#16921,.T.);
#22187=ORIENTED_EDGE('',*,*,#16922,.T.);
#22188=ORIENTED_EDGE('',*,*,#16917,.F.);
#22189=ORIENTED_EDGE('',*,*,#16682,.F.);
#22190=ORIENTED_EDGE('',*,*,#16923,.T.);
#22191=ORIENTED_EDGE('',*,*,#16924,.T.);
#22192=ORIENTED_EDGE('',*,*,#16919,.F.);
#22193=ORIENTED_EDGE('',*,*,#16922,.F.);
#22194=ORIENTED_EDGE('',*,*,#16925,.T.);
#22195=ORIENTED_EDGE('',*,*,#16926,.T.);
#22196=ORIENTED_EDGE('',*,*,#16921,.F.);
#22197=ORIENTED_EDGE('',*,*,#16681,.F.);
#22198=ORIENTED_EDGE('',*,*,#16926,.F.);
#22199=ORIENTED_EDGE('',*,*,#16927,.T.);
#22200=ORIENTED_EDGE('',*,*,#16928,.T.);
#22201=ORIENTED_EDGE('',*,*,#16923,.F.);
#22202=ORIENTED_EDGE('',*,*,#16929,.T.);
#22203=ORIENTED_EDGE('',*,*,#16930,.T.);
#22204=ORIENTED_EDGE('',*,*,#16925,.F.);
#22205=ORIENTED_EDGE('',*,*,#16680,.F.);
#22206=ORIENTED_EDGE('',*,*,#16930,.F.);
#22207=ORIENTED_EDGE('',*,*,#16931,.F.);
#22208=ORIENTED_EDGE('',*,*,#16932,.T.);
#22209=ORIENTED_EDGE('',*,*,#16927,.F.);
#22210=ORIENTED_EDGE('',*,*,#16933,.T.);
#22211=ORIENTED_EDGE('',*,*,#16934,.T.);
#22212=ORIENTED_EDGE('',*,*,#16929,.F.);
#22213=ORIENTED_EDGE('',*,*,#16679,.F.);
#22214=ORIENTED_EDGE('',*,*,#16935,.F.);
#22215=ORIENTED_EDGE('',*,*,#16936,.T.);
#22216=ORIENTED_EDGE('',*,*,#16931,.T.);
#22217=ORIENTED_EDGE('',*,*,#16934,.F.);
#22218=ORIENTED_EDGE('',*,*,#16937,.T.);
#22219=ORIENTED_EDGE('',*,*,#16938,.T.);
#22220=ORIENTED_EDGE('',*,*,#16933,.F.);
#22221=ORIENTED_EDGE('',*,*,#16678,.F.);
#22222=ORIENTED_EDGE('',*,*,#16939,.F.);
#22223=ORIENTED_EDGE('',*,*,#16940,.T.);
#22224=ORIENTED_EDGE('',*,*,#16935,.T.);
#22225=ORIENTED_EDGE('',*,*,#16938,.F.);
#22226=ORIENTED_EDGE('',*,*,#16941,.T.);
#22227=ORIENTED_EDGE('',*,*,#16942,.T.);
#22228=ORIENTED_EDGE('',*,*,#16937,.F.);
#22229=ORIENTED_EDGE('',*,*,#16677,.F.);
#22230=ORIENTED_EDGE('',*,*,#16943,.F.);
#22231=ORIENTED_EDGE('',*,*,#16944,.T.);
#22232=ORIENTED_EDGE('',*,*,#16939,.T.);
#22233=ORIENTED_EDGE('',*,*,#16942,.F.);
#22234=ORIENTED_EDGE('',*,*,#16945,.T.);
#22235=ORIENTED_EDGE('',*,*,#16946,.T.);
#22236=ORIENTED_EDGE('',*,*,#16941,.F.);
#22237=ORIENTED_EDGE('',*,*,#16676,.F.);
#22238=ORIENTED_EDGE('',*,*,#16947,.F.);
#22239=ORIENTED_EDGE('',*,*,#16948,.T.);
#22240=ORIENTED_EDGE('',*,*,#16943,.T.);
#22241=ORIENTED_EDGE('',*,*,#16946,.F.);
#22242=ORIENTED_EDGE('',*,*,#16949,.T.);
#22243=ORIENTED_EDGE('',*,*,#16950,.T.);
#22244=ORIENTED_EDGE('',*,*,#16945,.F.);
#22245=ORIENTED_EDGE('',*,*,#16715,.F.);
#22246=ORIENTED_EDGE('',*,*,#16951,.F.);
#22247=ORIENTED_EDGE('',*,*,#16952,.T.);
#22248=ORIENTED_EDGE('',*,*,#16947,.T.);
#22249=ORIENTED_EDGE('',*,*,#16950,.F.);
#22250=ORIENTED_EDGE('',*,*,#16953,.T.);
#22251=ORIENTED_EDGE('',*,*,#16954,.T.);
#22252=ORIENTED_EDGE('',*,*,#16949,.F.);
#22253=ORIENTED_EDGE('',*,*,#16714,.F.);
#22254=ORIENTED_EDGE('',*,*,#16955,.F.);
#22255=ORIENTED_EDGE('',*,*,#16956,.T.);
#22256=ORIENTED_EDGE('',*,*,#16951,.T.);
#22257=ORIENTED_EDGE('',*,*,#16954,.F.);
#22258=ORIENTED_EDGE('',*,*,#16957,.T.);
#22259=ORIENTED_EDGE('',*,*,#16958,.T.);
#22260=ORIENTED_EDGE('',*,*,#16953,.F.);
#22261=ORIENTED_EDGE('',*,*,#16713,.F.);
#22262=ORIENTED_EDGE('',*,*,#16959,.F.);
#22263=ORIENTED_EDGE('',*,*,#16960,.T.);
#22264=ORIENTED_EDGE('',*,*,#16955,.T.);
#22265=ORIENTED_EDGE('',*,*,#16958,.F.);
#22266=ORIENTED_EDGE('',*,*,#16961,.T.);
#22267=ORIENTED_EDGE('',*,*,#16962,.T.);
#22268=ORIENTED_EDGE('',*,*,#16957,.F.);
#22269=ORIENTED_EDGE('',*,*,#16712,.F.);
#22270=ORIENTED_EDGE('',*,*,#16963,.T.);
#22271=ORIENTED_EDGE('',*,*,#16964,.T.);
#22272=ORIENTED_EDGE('',*,*,#16959,.T.);
#22273=ORIENTED_EDGE('',*,*,#16962,.F.);
#22274=ORIENTED_EDGE('',*,*,#16965,.T.);
#22275=ORIENTED_EDGE('',*,*,#16966,.T.);
#22276=ORIENTED_EDGE('',*,*,#16961,.F.);
#22277=ORIENTED_EDGE('',*,*,#16711,.F.);
#22278=ORIENTED_EDGE('',*,*,#16966,.F.);
#22279=ORIENTED_EDGE('',*,*,#16967,.T.);
#22280=ORIENTED_EDGE('',*,*,#16968,.T.);
#22281=ORIENTED_EDGE('',*,*,#16963,.F.);
#22282=ORIENTED_EDGE('',*,*,#16969,.T.);
#22283=ORIENTED_EDGE('',*,*,#16970,.T.);
#22284=ORIENTED_EDGE('',*,*,#16965,.F.);
#22285=ORIENTED_EDGE('',*,*,#16710,.F.);
#22286=ORIENTED_EDGE('',*,*,#16970,.F.);
#22287=ORIENTED_EDGE('',*,*,#16971,.T.);
#22288=ORIENTED_EDGE('',*,*,#16972,.T.);
#22289=ORIENTED_EDGE('',*,*,#16967,.F.);
#22290=ORIENTED_EDGE('',*,*,#16828,.T.);
#22291=ORIENTED_EDGE('',*,*,#16973,.T.);
#22292=ORIENTED_EDGE('',*,*,#16974,.F.);
#22293=ORIENTED_EDGE('',*,*,#16707,.F.);
#22294=ORIENTED_EDGE('',*,*,#16824,.F.);
#22295=ORIENTED_EDGE('',*,*,#16975,.T.);
#22296=ORIENTED_EDGE('',*,*,#16976,.T.);
#22297=ORIENTED_EDGE('',*,*,#16973,.F.);
#22298=ORIENTED_EDGE('',*,*,#16977,.T.);
#22299=ORIENTED_EDGE('',*,*,#16978,.T.);
#22300=ORIENTED_EDGE('',*,*,#16969,.F.);
#22301=ORIENTED_EDGE('',*,*,#16709,.F.);
#22302=ORIENTED_EDGE('',*,*,#16978,.F.);
#22303=ORIENTED_EDGE('',*,*,#16979,.T.);
#22304=ORIENTED_EDGE('',*,*,#16980,.T.);
#22305=ORIENTED_EDGE('',*,*,#16971,.F.);
#22306=ORIENTED_EDGE('',*,*,#16974,.T.);
#22307=ORIENTED_EDGE('',*,*,#16981,.T.);
#22308=ORIENTED_EDGE('',*,*,#16977,.F.);
#22309=ORIENTED_EDGE('',*,*,#16708,.F.);
#22310=ORIENTED_EDGE('',*,*,#16981,.F.);
#22311=ORIENTED_EDGE('',*,*,#16976,.F.);
#22312=ORIENTED_EDGE('',*,*,#16982,.T.);
#22313=ORIENTED_EDGE('',*,*,#16979,.F.);
#22314=ORIENTED_EDGE('',*,*,#16983,.T.);
#22315=ORIENTED_EDGE('',*,*,#16984,.F.);
#22316=ORIENTED_EDGE('',*,*,#16985,.F.);
#22317=ORIENTED_EDGE('',*,*,#16986,.F.);
#22318=ORIENTED_EDGE('',*,*,#16987,.T.);
#22319=ORIENTED_EDGE('',*,*,#16988,.F.);
#22320=ORIENTED_EDGE('',*,*,#16989,.F.);
#22321=ORIENTED_EDGE('',*,*,#16990,.F.);
#22322=ORIENTED_EDGE('',*,*,#16991,.T.);
#22323=ORIENTED_EDGE('',*,*,#16992,.T.);
#22324=ORIENTED_EDGE('',*,*,#16987,.F.);
#22325=ORIENTED_EDGE('',*,*,#16993,.F.);
#22326=ORIENTED_EDGE('',*,*,#16994,.F.);
#22327=ORIENTED_EDGE('',*,*,#16989,.T.);
#22328=ORIENTED_EDGE('',*,*,#16995,.T.);
#22329=ORIENTED_EDGE('',*,*,#16996,.F.);
#22330=ORIENTED_EDGE('',*,*,#16997,.F.);
#22331=ORIENTED_EDGE('',*,*,#16998,.F.);
#22332=ORIENTED_EDGE('',*,*,#16996,.T.);
#22333=ORIENTED_EDGE('',*,*,#16999,.T.);
#22334=ORIENTED_EDGE('',*,*,#17000,.F.);
#22335=ORIENTED_EDGE('',*,*,#17001,.F.);
#22336=ORIENTED_EDGE('',*,*,#17000,.T.);
#22337=ORIENTED_EDGE('',*,*,#17002,.T.);
#22338=ORIENTED_EDGE('',*,*,#16744,.F.);
#22339=ORIENTED_EDGE('',*,*,#17003,.F.);
#22340=ORIENTED_EDGE('',*,*,#17004,.T.);
#22341=ORIENTED_EDGE('',*,*,#17005,.F.);
#22342=ORIENTED_EDGE('',*,*,#17006,.F.);
#22343=ORIENTED_EDGE('',*,*,#17007,.F.);
#22344=ORIENTED_EDGE('',*,*,#17008,.T.);
#22345=ORIENTED_EDGE('',*,*,#17009,.T.);
#22346=ORIENTED_EDGE('',*,*,#17010,.F.);
#22347=ORIENTED_EDGE('',*,*,#17011,.F.);
#22348=ORIENTED_EDGE('',*,*,#17012,.T.);
#22349=ORIENTED_EDGE('',*,*,#17013,.T.);
#22350=ORIENTED_EDGE('',*,*,#17008,.F.);
#22351=ORIENTED_EDGE('',*,*,#17014,.F.);
#22352=ORIENTED_EDGE('',*,*,#16746,.T.);
#22353=ORIENTED_EDGE('',*,*,#17015,.F.);
#22354=ORIENTED_EDGE('',*,*,#17012,.F.);
#22355=ORIENTED_EDGE('',*,*,#17016,.F.);
#22356=ORIENTED_EDGE('',*,*,#17017,.F.);
#22357=ORIENTED_EDGE('',*,*,#17018,.T.);
#22358=ORIENTED_EDGE('',*,*,#17019,.T.);
#22359=ORIENTED_EDGE('',*,*,#16752,.F.);
#22360=ORIENTED_EDGE('',*,*,#17020,.F.);
#22361=ORIENTED_EDGE('',*,*,#17021,.T.);
#22362=ORIENTED_EDGE('',*,*,#16985,.T.);
#22363=ORIENTED_EDGE('',*,*,#17022,.T.);
#22364=ORIENTED_EDGE('',*,*,#17023,.F.);
#22365=ORIENTED_EDGE('',*,*,#16756,.T.);
#22366=ORIENTED_EDGE('',*,*,#17024,.T.);
#22367=ORIENTED_EDGE('',*,*,#17025,.F.);
#22368=ORIENTED_EDGE('',*,*,#17026,.F.);
#22369=ORIENTED_EDGE('',*,*,#16759,.T.);
#22370=ORIENTED_EDGE('',*,*,#17027,.T.);
#22371=ORIENTED_EDGE('',*,*,#17028,.F.);
#22372=ORIENTED_EDGE('',*,*,#17029,.F.);
#22373=ORIENTED_EDGE('',*,*,#16760,.T.);
#22374=ORIENTED_EDGE('',*,*,#17029,.T.);
#22375=ORIENTED_EDGE('',*,*,#17030,.F.);
#22376=ORIENTED_EDGE('',*,*,#17024,.F.);
#22377=ORIENTED_EDGE('',*,*,#16762,.T.);
#22378=ORIENTED_EDGE('',*,*,#17031,.T.);
#22379=ORIENTED_EDGE('',*,*,#17032,.F.);
#22380=ORIENTED_EDGE('',*,*,#17027,.F.);
#22381=ORIENTED_EDGE('',*,*,#16764,.T.);
#22382=ORIENTED_EDGE('',*,*,#17033,.T.);
#22383=ORIENTED_EDGE('',*,*,#17034,.F.);
#22384=ORIENTED_EDGE('',*,*,#17035,.F.);
#22385=ORIENTED_EDGE('',*,*,#16765,.T.);
#22386=ORIENTED_EDGE('',*,*,#17035,.T.);
#22387=ORIENTED_EDGE('',*,*,#17036,.F.);
#22388=ORIENTED_EDGE('',*,*,#17037,.F.);
#22389=ORIENTED_EDGE('',*,*,#16766,.T.);
#22390=ORIENTED_EDGE('',*,*,#17037,.T.);
#22391=ORIENTED_EDGE('',*,*,#17038,.F.);
#22392=ORIENTED_EDGE('',*,*,#17031,.F.);
#22393=ORIENTED_EDGE('',*,*,#16770,.T.);
#22394=ORIENTED_EDGE('',*,*,#17039,.T.);
#22395=ORIENTED_EDGE('',*,*,#17040,.F.);
#22396=ORIENTED_EDGE('',*,*,#17041,.F.);
#22397=ORIENTED_EDGE('',*,*,#16769,.T.);
#22398=ORIENTED_EDGE('',*,*,#17042,.T.);
#22399=ORIENTED_EDGE('',*,*,#17043,.F.);
#22400=ORIENTED_EDGE('',*,*,#17039,.F.);
#22401=ORIENTED_EDGE('',*,*,#16768,.T.);
#22402=ORIENTED_EDGE('',*,*,#17044,.T.);
#22403=ORIENTED_EDGE('',*,*,#17045,.F.);
#22404=ORIENTED_EDGE('',*,*,#17042,.F.);
#22405=ORIENTED_EDGE('',*,*,#16771,.T.);
#22406=ORIENTED_EDGE('',*,*,#17041,.T.);
#22407=ORIENTED_EDGE('',*,*,#17046,.F.);
#22408=ORIENTED_EDGE('',*,*,#17033,.F.);
#22409=ORIENTED_EDGE('',*,*,#16774,.T.);
#22410=ORIENTED_EDGE('',*,*,#17047,.T.);
#22411=ORIENTED_EDGE('',*,*,#17048,.F.);
#22412=ORIENTED_EDGE('',*,*,#17044,.F.);
#22413=ORIENTED_EDGE('',*,*,#16773,.T.);
#22414=ORIENTED_EDGE('',*,*,#17049,.T.);
#22415=ORIENTED_EDGE('',*,*,#17050,.F.);
#22416=ORIENTED_EDGE('',*,*,#17047,.F.);
#22417=ORIENTED_EDGE('',*,*,#16779,.T.);
#22418=ORIENTED_EDGE('',*,*,#17051,.T.);
#22419=ORIENTED_EDGE('',*,*,#17052,.F.);
#22420=ORIENTED_EDGE('',*,*,#17049,.F.);
#22421=ORIENTED_EDGE('',*,*,#16778,.T.);
#22422=ORIENTED_EDGE('',*,*,#17053,.T.);
#22423=ORIENTED_EDGE('',*,*,#17054,.F.);
#22424=ORIENTED_EDGE('',*,*,#17051,.F.);
#22425=ORIENTED_EDGE('',*,*,#16777,.T.);
#22426=ORIENTED_EDGE('',*,*,#17055,.T.);
#22427=ORIENTED_EDGE('',*,*,#17056,.F.);
#22428=ORIENTED_EDGE('',*,*,#17053,.F.);
#22429=ORIENTED_EDGE('',*,*,#16776,.T.);
#22430=ORIENTED_EDGE('',*,*,#17057,.T.);
#22431=ORIENTED_EDGE('',*,*,#17058,.F.);
#22432=ORIENTED_EDGE('',*,*,#17055,.F.);
#22433=ORIENTED_EDGE('',*,*,#17058,.T.);
#22434=ORIENTED_EDGE('',*,*,#17059,.T.);
#22435=ORIENTED_EDGE('',*,*,#16781,.F.);
#22436=ORIENTED_EDGE('',*,*,#17060,.T.);
#22437=ORIENTED_EDGE('',*,*,#17061,.F.);
#22438=ORIENTED_EDGE('',*,*,#17062,.F.);
#22439=ORIENTED_EDGE('',*,*,#16782,.T.);
#22440=ORIENTED_EDGE('',*,*,#17059,.F.);
#22441=ORIENTED_EDGE('',*,*,#17057,.F.);
#22442=ORIENTED_EDGE('',*,*,#17063,.T.);
#22443=ORIENTED_EDGE('',*,*,#17064,.T.);
#22444=ORIENTED_EDGE('',*,*,#17065,.T.);
#22445=ORIENTED_EDGE('',*,*,#17066,.F.);
#22446=ORIENTED_EDGE('',*,*,#17060,.F.);
#22447=ORIENTED_EDGE('',*,*,#16785,.F.);
#22448=ORIENTED_EDGE('',*,*,#16784,.T.);
#22449=ORIENTED_EDGE('',*,*,#17067,.T.);
#22450=ORIENTED_EDGE('',*,*,#17063,.F.);
#22451=ORIENTED_EDGE('',*,*,#16786,.T.);
#22452=ORIENTED_EDGE('',*,*,#17026,.T.);
#22453=ORIENTED_EDGE('',*,*,#17068,.F.);
#22454=ORIENTED_EDGE('',*,*,#17069,.F.);
#22455=ORIENTED_EDGE('',*,*,#16787,.T.);
#22456=ORIENTED_EDGE('',*,*,#17069,.T.);
#22457=ORIENTED_EDGE('',*,*,#17070,.F.);
#22458=ORIENTED_EDGE('',*,*,#17071,.F.);
#22459=ORIENTED_EDGE('',*,*,#16788,.T.);
#22460=ORIENTED_EDGE('',*,*,#17071,.T.);
#22461=ORIENTED_EDGE('',*,*,#17064,.F.);
#22462=ORIENTED_EDGE('',*,*,#17067,.F.);
#22463=ORIENTED_EDGE('',*,*,#17072,.T.);
#22464=ORIENTED_EDGE('',*,*,#17073,.T.);
#22465=ORIENTED_EDGE('',*,*,#17074,.F.);
#22466=ORIENTED_EDGE('',*,*,#16790,.F.);
#22467=ORIENTED_EDGE('',*,*,#17074,.T.);
#22468=ORIENTED_EDGE('',*,*,#17075,.T.);
#22469=ORIENTED_EDGE('',*,*,#17076,.F.);
#22470=ORIENTED_EDGE('',*,*,#16791,.F.);
#22471=ORIENTED_EDGE('',*,*,#17077,.T.);
#22472=ORIENTED_EDGE('',*,*,#17078,.T.);
#22473=ORIENTED_EDGE('',*,*,#17072,.F.);
#22474=ORIENTED_EDGE('',*,*,#16794,.F.);
#22475=ORIENTED_EDGE('',*,*,#17079,.T.);
#22476=ORIENTED_EDGE('',*,*,#17080,.T.);
#22477=ORIENTED_EDGE('',*,*,#17081,.F.);
#22478=ORIENTED_EDGE('',*,*,#16796,.F.);
#22479=ORIENTED_EDGE('',*,*,#17081,.T.);
#22480=ORIENTED_EDGE('',*,*,#17007,.T.);
#22481=ORIENTED_EDGE('',*,*,#17082,.F.);
#22482=ORIENTED_EDGE('',*,*,#16797,.F.);
#22483=ORIENTED_EDGE('',*,*,#17082,.T.);
#22484=ORIENTED_EDGE('',*,*,#17083,.T.);
#22485=ORIENTED_EDGE('',*,*,#17077,.F.);
#22486=ORIENTED_EDGE('',*,*,#16798,.F.);
#22487=ORIENTED_EDGE('',*,*,#17084,.T.);
#22488=ORIENTED_EDGE('',*,*,#17079,.F.);
#22489=ORIENTED_EDGE('',*,*,#16801,.F.);
#22490=ORIENTED_EDGE('',*,*,#16800,.T.);
#22491=ORIENTED_EDGE('',*,*,#17085,.T.);
#22492=ORIENTED_EDGE('',*,*,#17086,.T.);
#22493=ORIENTED_EDGE('',*,*,#17004,.F.);
#22494=ORIENTED_EDGE('',*,*,#17080,.F.);
#22495=ORIENTED_EDGE('',*,*,#17084,.F.);
#22496=ORIENTED_EDGE('',*,*,#17010,.T.);
#22497=ORIENTED_EDGE('',*,*,#17087,.T.);
#22498=ORIENTED_EDGE('',*,*,#17085,.F.);
#22499=ORIENTED_EDGE('',*,*,#16804,.T.);
#22500=ORIENTED_EDGE('',*,*,#17088,.F.);
#22501=ORIENTED_EDGE('',*,*,#17089,.F.);
#22502=ORIENTED_EDGE('',*,*,#17090,.T.);
#22503=ORIENTED_EDGE('',*,*,#17088,.T.);
#22504=ORIENTED_EDGE('',*,*,#16803,.F.);
#22505=ORIENTED_EDGE('',*,*,#17091,.T.);
#22506=ORIENTED_EDGE('',*,*,#17089,.T.);
#22507=ORIENTED_EDGE('',*,*,#17090,.F.);
#22508=ORIENTED_EDGE('',*,*,#16809,.F.);
#22509=ORIENTED_EDGE('',*,*,#17092,.T.);
#22510=ORIENTED_EDGE('',*,*,#17011,.T.);
#22511=ORIENTED_EDGE('',*,*,#17091,.F.);
#22512=ORIENTED_EDGE('',*,*,#16808,.F.);
#22513=ORIENTED_EDGE('',*,*,#17093,.T.);
#22514=ORIENTED_EDGE('',*,*,#17014,.T.);
#22515=ORIENTED_EDGE('',*,*,#17092,.F.);
#22516=ORIENTED_EDGE('',*,*,#16807,.F.);
#22517=ORIENTED_EDGE('',*,*,#17094,.T.);
#22518=ORIENTED_EDGE('',*,*,#17016,.T.);
#22519=ORIENTED_EDGE('',*,*,#17093,.F.);
#22520=ORIENTED_EDGE('',*,*,#16806,.F.);
#22521=ORIENTED_EDGE('',*,*,#17095,.T.);
#22522=ORIENTED_EDGE('',*,*,#17017,.T.);
#22523=ORIENTED_EDGE('',*,*,#17094,.F.);
#22524=ORIENTED_EDGE('',*,*,#16812,.F.);
#22525=ORIENTED_EDGE('',*,*,#17096,.T.);
#22526=ORIENTED_EDGE('',*,*,#16747,.T.);
#22527=ORIENTED_EDGE('',*,*,#17095,.F.);
#22528=ORIENTED_EDGE('',*,*,#16811,.F.);
#22529=ORIENTED_EDGE('',*,*,#17097,.T.);
#22530=ORIENTED_EDGE('',*,*,#16748,.T.);
#22531=ORIENTED_EDGE('',*,*,#17096,.F.);
#22532=ORIENTED_EDGE('',*,*,#16817,.F.);
#22533=ORIENTED_EDGE('',*,*,#17098,.T.);
#22534=ORIENTED_EDGE('',*,*,#17003,.T.);
#22535=ORIENTED_EDGE('',*,*,#17097,.F.);
#22536=ORIENTED_EDGE('',*,*,#16816,.F.);
#22537=ORIENTED_EDGE('',*,*,#17099,.T.);
#22538=ORIENTED_EDGE('',*,*,#17001,.T.);
#22539=ORIENTED_EDGE('',*,*,#17098,.F.);
#22540=ORIENTED_EDGE('',*,*,#16815,.F.);
#22541=ORIENTED_EDGE('',*,*,#17100,.T.);
#22542=ORIENTED_EDGE('',*,*,#16997,.T.);
#22543=ORIENTED_EDGE('',*,*,#17099,.F.);
#22544=ORIENTED_EDGE('',*,*,#16814,.F.);
#22545=ORIENTED_EDGE('',*,*,#17101,.T.);
#22546=ORIENTED_EDGE('',*,*,#16993,.T.);
#22547=ORIENTED_EDGE('',*,*,#17102,.F.);
#22548=ORIENTED_EDGE('',*,*,#16819,.F.);
#22549=ORIENTED_EDGE('',*,*,#17102,.T.);
#22550=ORIENTED_EDGE('',*,*,#16990,.T.);
#22551=ORIENTED_EDGE('',*,*,#17103,.F.);
#22552=ORIENTED_EDGE('',*,*,#16820,.F.);
#22553=ORIENTED_EDGE('',*,*,#17103,.T.);
#22554=ORIENTED_EDGE('',*,*,#16998,.T.);
#22555=ORIENTED_EDGE('',*,*,#17100,.F.);
#22556=ORIENTED_EDGE('',*,*,#16821,.F.);
#22557=ORIENTED_EDGE('',*,*,#17076,.T.);
#22558=ORIENTED_EDGE('',*,*,#16994,.T.);
#22559=ORIENTED_EDGE('',*,*,#17101,.F.);
#22560=ORIENTED_EDGE('',*,*,#16822,.F.);
#22561=ORIENTED_EDGE('',*,*,#17104,.T.);
#22562=ORIENTED_EDGE('',*,*,#17105,.T.);
#22563=ORIENTED_EDGE('',*,*,#17106,.F.);
#22564=ORIENTED_EDGE('',*,*,#16823,.F.);
#22565=ORIENTED_EDGE('',*,*,#17107,.T.);
#22566=ORIENTED_EDGE('',*,*,#17108,.T.);
#22567=ORIENTED_EDGE('',*,*,#17104,.F.);
#22568=ORIENTED_EDGE('',*,*,#16832,.F.);
#22569=ORIENTED_EDGE('',*,*,#17109,.T.);
#22570=ORIENTED_EDGE('',*,*,#17110,.T.);
#22571=ORIENTED_EDGE('',*,*,#17107,.F.);
#22572=ORIENTED_EDGE('',*,*,#16836,.F.);
#22573=ORIENTED_EDGE('',*,*,#17111,.T.);
#22574=ORIENTED_EDGE('',*,*,#17112,.T.);
#22575=ORIENTED_EDGE('',*,*,#17109,.F.);
#22576=ORIENTED_EDGE('',*,*,#16840,.F.);
#22577=ORIENTED_EDGE('',*,*,#17113,.T.);
#22578=ORIENTED_EDGE('',*,*,#17114,.T.);
#22579=ORIENTED_EDGE('',*,*,#17111,.F.);
#22580=ORIENTED_EDGE('',*,*,#16844,.F.);
#22581=ORIENTED_EDGE('',*,*,#17115,.T.);
#22582=ORIENTED_EDGE('',*,*,#17116,.T.);
#22583=ORIENTED_EDGE('',*,*,#17113,.F.);
#22584=ORIENTED_EDGE('',*,*,#16848,.F.);
#22585=ORIENTED_EDGE('',*,*,#17117,.T.);
#22586=ORIENTED_EDGE('',*,*,#17118,.T.);
#22587=ORIENTED_EDGE('',*,*,#17115,.F.);
#22588=ORIENTED_EDGE('',*,*,#16852,.F.);
#22589=ORIENTED_EDGE('',*,*,#17119,.T.);
#22590=ORIENTED_EDGE('',*,*,#17120,.T.);
#22591=ORIENTED_EDGE('',*,*,#17117,.F.);
#22592=ORIENTED_EDGE('',*,*,#16856,.F.);
#22593=ORIENTED_EDGE('',*,*,#17121,.T.);
#22594=ORIENTED_EDGE('',*,*,#17122,.T.);
#22595=ORIENTED_EDGE('',*,*,#17119,.F.);
#22596=ORIENTED_EDGE('',*,*,#16860,.F.);
#22597=ORIENTED_EDGE('',*,*,#17123,.T.);
#22598=ORIENTED_EDGE('',*,*,#17124,.T.);
#22599=ORIENTED_EDGE('',*,*,#17121,.F.);
#22600=ORIENTED_EDGE('',*,*,#16864,.F.);
#22601=ORIENTED_EDGE('',*,*,#17125,.T.);
#22602=ORIENTED_EDGE('',*,*,#17126,.T.);
#22603=ORIENTED_EDGE('',*,*,#17123,.F.);
#22604=ORIENTED_EDGE('',*,*,#16868,.F.);
#22605=ORIENTED_EDGE('',*,*,#17127,.T.);
#22606=ORIENTED_EDGE('',*,*,#17128,.T.);
#22607=ORIENTED_EDGE('',*,*,#17125,.F.);
#22608=ORIENTED_EDGE('',*,*,#16872,.F.);
#22609=ORIENTED_EDGE('',*,*,#17129,.T.);
#22610=ORIENTED_EDGE('',*,*,#17130,.T.);
#22611=ORIENTED_EDGE('',*,*,#17127,.F.);
#22612=ORIENTED_EDGE('',*,*,#16876,.F.);
#22613=ORIENTED_EDGE('',*,*,#17131,.T.);
#22614=ORIENTED_EDGE('',*,*,#17132,.T.);
#22615=ORIENTED_EDGE('',*,*,#17129,.F.);
#22616=ORIENTED_EDGE('',*,*,#16880,.F.);
#22617=ORIENTED_EDGE('',*,*,#17133,.T.);
#22618=ORIENTED_EDGE('',*,*,#17134,.T.);
#22619=ORIENTED_EDGE('',*,*,#17131,.F.);
#22620=ORIENTED_EDGE('',*,*,#16884,.F.);
#22621=ORIENTED_EDGE('',*,*,#17135,.T.);
#22622=ORIENTED_EDGE('',*,*,#17136,.T.);
#22623=ORIENTED_EDGE('',*,*,#17133,.F.);
#22624=ORIENTED_EDGE('',*,*,#16888,.F.);
#22625=ORIENTED_EDGE('',*,*,#17137,.T.);
#22626=ORIENTED_EDGE('',*,*,#17138,.T.);
#22627=ORIENTED_EDGE('',*,*,#17135,.F.);
#22628=ORIENTED_EDGE('',*,*,#16892,.F.);
#22629=ORIENTED_EDGE('',*,*,#17139,.T.);
#22630=ORIENTED_EDGE('',*,*,#17140,.T.);
#22631=ORIENTED_EDGE('',*,*,#17137,.F.);
#22632=ORIENTED_EDGE('',*,*,#16896,.F.);
#22633=ORIENTED_EDGE('',*,*,#17141,.T.);
#22634=ORIENTED_EDGE('',*,*,#17142,.T.);
#22635=ORIENTED_EDGE('',*,*,#17139,.F.);
#22636=ORIENTED_EDGE('',*,*,#16900,.F.);
#22637=ORIENTED_EDGE('',*,*,#17143,.T.);
#22638=ORIENTED_EDGE('',*,*,#17144,.T.);
#22639=ORIENTED_EDGE('',*,*,#17141,.F.);
#22640=ORIENTED_EDGE('',*,*,#16904,.F.);
#22641=ORIENTED_EDGE('',*,*,#17145,.T.);
#22642=ORIENTED_EDGE('',*,*,#17146,.T.);
#22643=ORIENTED_EDGE('',*,*,#17143,.F.);
#22644=ORIENTED_EDGE('',*,*,#16905,.F.);
#22645=ORIENTED_EDGE('',*,*,#17147,.T.);
#22646=ORIENTED_EDGE('',*,*,#17148,.T.);
#22647=ORIENTED_EDGE('',*,*,#17145,.F.);
#22648=ORIENTED_EDGE('',*,*,#16912,.F.);
#22649=ORIENTED_EDGE('',*,*,#17149,.T.);
#22650=ORIENTED_EDGE('',*,*,#17150,.T.);
#22651=ORIENTED_EDGE('',*,*,#17147,.F.);
#22652=ORIENTED_EDGE('',*,*,#16916,.F.);
#22653=ORIENTED_EDGE('',*,*,#17151,.T.);
#22654=ORIENTED_EDGE('',*,*,#17152,.T.);
#22655=ORIENTED_EDGE('',*,*,#17149,.F.);
#22656=ORIENTED_EDGE('',*,*,#16920,.F.);
#22657=ORIENTED_EDGE('',*,*,#17153,.T.);
#22658=ORIENTED_EDGE('',*,*,#17154,.T.);
#22659=ORIENTED_EDGE('',*,*,#17151,.F.);
#22660=ORIENTED_EDGE('',*,*,#16924,.F.);
#22661=ORIENTED_EDGE('',*,*,#17155,.T.);
#22662=ORIENTED_EDGE('',*,*,#17156,.T.);
#22663=ORIENTED_EDGE('',*,*,#17153,.F.);
#22664=ORIENTED_EDGE('',*,*,#16928,.F.);
#22665=ORIENTED_EDGE('',*,*,#17157,.T.);
#22666=ORIENTED_EDGE('',*,*,#17158,.T.);
#22667=ORIENTED_EDGE('',*,*,#17155,.F.);
#22668=ORIENTED_EDGE('',*,*,#16932,.F.);
#22669=ORIENTED_EDGE('',*,*,#17159,.T.);
#22670=ORIENTED_EDGE('',*,*,#17160,.T.);
#22671=ORIENTED_EDGE('',*,*,#17157,.F.);
#22672=ORIENTED_EDGE('',*,*,#16936,.F.);
#22673=ORIENTED_EDGE('',*,*,#17161,.T.);
#22674=ORIENTED_EDGE('',*,*,#17162,.T.);
#22675=ORIENTED_EDGE('',*,*,#17159,.F.);
#22676=ORIENTED_EDGE('',*,*,#16940,.F.);
#22677=ORIENTED_EDGE('',*,*,#17163,.T.);
#22678=ORIENTED_EDGE('',*,*,#17164,.T.);
#22679=ORIENTED_EDGE('',*,*,#17161,.F.);
#22680=ORIENTED_EDGE('',*,*,#16944,.F.);
#22681=ORIENTED_EDGE('',*,*,#17165,.T.);
#22682=ORIENTED_EDGE('',*,*,#17166,.T.);
#22683=ORIENTED_EDGE('',*,*,#17163,.F.);
#22684=ORIENTED_EDGE('',*,*,#16948,.F.);
#22685=ORIENTED_EDGE('',*,*,#17167,.T.);
#22686=ORIENTED_EDGE('',*,*,#17168,.T.);
#22687=ORIENTED_EDGE('',*,*,#17165,.F.);
#22688=ORIENTED_EDGE('',*,*,#16952,.F.);
#22689=ORIENTED_EDGE('',*,*,#17169,.T.);
#22690=ORIENTED_EDGE('',*,*,#17170,.T.);
#22691=ORIENTED_EDGE('',*,*,#17167,.F.);
#22692=ORIENTED_EDGE('',*,*,#16956,.F.);
#22693=ORIENTED_EDGE('',*,*,#17171,.T.);
#22694=ORIENTED_EDGE('',*,*,#17172,.T.);
#22695=ORIENTED_EDGE('',*,*,#17169,.F.);
#22696=ORIENTED_EDGE('',*,*,#16960,.F.);
#22697=ORIENTED_EDGE('',*,*,#17173,.T.);
#22698=ORIENTED_EDGE('',*,*,#17174,.T.);
#22699=ORIENTED_EDGE('',*,*,#17171,.F.);
#22700=ORIENTED_EDGE('',*,*,#16964,.F.);
#22701=ORIENTED_EDGE('',*,*,#17175,.T.);
#22702=ORIENTED_EDGE('',*,*,#17176,.T.);
#22703=ORIENTED_EDGE('',*,*,#17173,.F.);
#22704=ORIENTED_EDGE('',*,*,#16968,.F.);
#22705=ORIENTED_EDGE('',*,*,#17177,.T.);
#22706=ORIENTED_EDGE('',*,*,#17178,.T.);
#22707=ORIENTED_EDGE('',*,*,#17175,.F.);
#22708=ORIENTED_EDGE('',*,*,#16972,.F.);
#22709=ORIENTED_EDGE('',*,*,#17106,.T.);
#22710=ORIENTED_EDGE('',*,*,#17179,.T.);
#22711=ORIENTED_EDGE('',*,*,#17180,.F.);
#22712=ORIENTED_EDGE('',*,*,#16975,.F.);
#22713=ORIENTED_EDGE('',*,*,#17181,.T.);
#22714=ORIENTED_EDGE('',*,*,#17182,.T.);
#22715=ORIENTED_EDGE('',*,*,#17177,.F.);
#22716=ORIENTED_EDGE('',*,*,#16980,.F.);
#22717=ORIENTED_EDGE('',*,*,#17180,.T.);
#22718=ORIENTED_EDGE('',*,*,#17183,.T.);
#22719=ORIENTED_EDGE('',*,*,#17181,.F.);
#22720=ORIENTED_EDGE('',*,*,#16982,.F.);
#22721=ORIENTED_EDGE('',*,*,#17168,.F.);
#22722=ORIENTED_EDGE('',*,*,#17170,.F.);
#22723=ORIENTED_EDGE('',*,*,#17172,.F.);
#22724=ORIENTED_EDGE('',*,*,#17174,.F.);
#22725=ORIENTED_EDGE('',*,*,#17176,.F.);
#22726=ORIENTED_EDGE('',*,*,#17178,.F.);
#22727=ORIENTED_EDGE('',*,*,#17182,.F.);
#22728=ORIENTED_EDGE('',*,*,#17183,.F.);
#22729=ORIENTED_EDGE('',*,*,#17179,.F.);
#22730=ORIENTED_EDGE('',*,*,#17105,.F.);
#22731=ORIENTED_EDGE('',*,*,#17108,.F.);
#22732=ORIENTED_EDGE('',*,*,#17110,.F.);
#22733=ORIENTED_EDGE('',*,*,#17112,.F.);
#22734=ORIENTED_EDGE('',*,*,#17114,.F.);
#22735=ORIENTED_EDGE('',*,*,#17116,.F.);
#22736=ORIENTED_EDGE('',*,*,#17118,.F.);
#22737=ORIENTED_EDGE('',*,*,#17120,.F.);
#22738=ORIENTED_EDGE('',*,*,#17122,.F.);
#22739=ORIENTED_EDGE('',*,*,#17124,.F.);
#22740=ORIENTED_EDGE('',*,*,#17126,.F.);
#22741=ORIENTED_EDGE('',*,*,#17128,.F.);
#22742=ORIENTED_EDGE('',*,*,#17130,.F.);
#22743=ORIENTED_EDGE('',*,*,#17132,.F.);
#22744=ORIENTED_EDGE('',*,*,#17134,.F.);
#22745=ORIENTED_EDGE('',*,*,#17136,.F.);
#22746=ORIENTED_EDGE('',*,*,#17138,.F.);
#22747=ORIENTED_EDGE('',*,*,#17140,.F.);
#22748=ORIENTED_EDGE('',*,*,#17142,.F.);
#22749=ORIENTED_EDGE('',*,*,#17144,.F.);
#22750=ORIENTED_EDGE('',*,*,#17146,.F.);
#22751=ORIENTED_EDGE('',*,*,#17148,.F.);
#22752=ORIENTED_EDGE('',*,*,#17150,.F.);
#22753=ORIENTED_EDGE('',*,*,#17152,.F.);
#22754=ORIENTED_EDGE('',*,*,#17154,.F.);
#22755=ORIENTED_EDGE('',*,*,#17156,.F.);
#22756=ORIENTED_EDGE('',*,*,#17158,.F.);
#22757=ORIENTED_EDGE('',*,*,#17160,.F.);
#22758=ORIENTED_EDGE('',*,*,#17162,.F.);
#22759=ORIENTED_EDGE('',*,*,#17164,.F.);
#22760=ORIENTED_EDGE('',*,*,#17166,.F.);
#22761=ORIENTED_EDGE('',*,*,#17020,.T.);
#22762=ORIENTED_EDGE('',*,*,#16751,.F.);
#22763=ORIENTED_EDGE('',*,*,#17184,.F.);
#22764=ORIENTED_EDGE('',*,*,#17185,.F.);
#22765=ORIENTED_EDGE('',*,*,#17186,.T.);
#22766=ORIENTED_EDGE('',*,*,#17187,.F.);
#22767=ORIENTED_EDGE('',*,*,#17188,.T.);
#22768=ORIENTED_EDGE('',*,*,#17189,.F.);
#22769=ORIENTED_EDGE('',*,*,#17190,.F.);
#22770=ORIENTED_EDGE('',*,*,#17191,.F.);
#22771=ORIENTED_EDGE('',*,*,#17192,.F.);
#22772=ORIENTED_EDGE('',*,*,#17193,.F.);
#22773=ORIENTED_EDGE('',*,*,#16986,.T.);
#22774=ORIENTED_EDGE('',*,*,#17021,.F.);
#22775=ORIENTED_EDGE('',*,*,#17194,.F.);
#22776=ORIENTED_EDGE('',*,*,#17195,.T.);
#22777=ORIENTED_EDGE('',*,*,#17196,.F.);
#22778=ORIENTED_EDGE('',*,*,#17197,.T.);
#22779=ORIENTED_EDGE('',*,*,#17198,.T.);
#22780=ORIENTED_EDGE('',*,*,#17199,.F.);
#22781=ORIENTED_EDGE('',*,*,#17200,.F.);
#22782=ORIENTED_EDGE('',*,*,#17201,.F.);
#22783=ORIENTED_EDGE('',*,*,#17202,.F.);
#22784=ORIENTED_EDGE('',*,*,#17203,.F.);
#22785=ORIENTED_EDGE('',*,*,#17198,.F.);
#22786=ORIENTED_EDGE('',*,*,#17204,.T.);
#22787=ORIENTED_EDGE('',*,*,#17205,.T.);
#22788=ORIENTED_EDGE('',*,*,#17184,.T.);
#22789=ORIENTED_EDGE('',*,*,#16754,.T.);
#22790=ORIENTED_EDGE('',*,*,#17206,.F.);
#22791=ORIENTED_EDGE('',*,*,#17207,.F.);
#22792=ORIENTED_EDGE('',*,*,#17199,.T.);
#22793=ORIENTED_EDGE('',*,*,#17203,.T.);
#22794=ORIENTED_EDGE('',*,*,#17208,.F.);
#22795=ORIENTED_EDGE('',*,*,#17209,.F.);
#22796=ORIENTED_EDGE('',*,*,#17210,.T.);
#22797=ORIENTED_EDGE('',*,*,#17211,.F.);
#22798=ORIENTED_EDGE('',*,*,#17200,.T.);
#22799=ORIENTED_EDGE('',*,*,#17209,.T.);
#22800=ORIENTED_EDGE('',*,*,#17201,.T.);
#22801=ORIENTED_EDGE('',*,*,#17211,.T.);
#22802=ORIENTED_EDGE('',*,*,#17212,.F.);
#22803=ORIENTED_EDGE('',*,*,#17213,.F.);
#22804=ORIENTED_EDGE('',*,*,#17214,.T.);
#22805=ORIENTED_EDGE('',*,*,#17018,.F.);
#22806=ORIENTED_EDGE('',*,*,#17202,.T.);
#22807=ORIENTED_EDGE('',*,*,#17213,.T.);
#22808=ORIENTED_EDGE('',*,*,#17215,.T.);
#22809=ORIENTED_EDGE('',*,*,#17216,.T.);
#22810=ORIENTED_EDGE('',*,*,#17217,.F.);
#22811=ORIENTED_EDGE('',*,*,#17186,.F.);
#22812=ORIENTED_EDGE('',*,*,#17218,.T.);
#22813=ORIENTED_EDGE('',*,*,#17215,.F.);
#22814=ORIENTED_EDGE('',*,*,#17185,.T.);
#22815=ORIENTED_EDGE('',*,*,#17207,.T.);
#22816=ORIENTED_EDGE('',*,*,#17219,.T.);
#22817=ORIENTED_EDGE('',*,*,#17220,.F.);
#22818=ORIENTED_EDGE('',*,*,#17187,.T.);
#22819=ORIENTED_EDGE('',*,*,#17217,.T.);
#22820=ORIENTED_EDGE('',*,*,#17220,.T.);
#22821=ORIENTED_EDGE('',*,*,#17221,.T.);
#22822=ORIENTED_EDGE('',*,*,#17222,.F.);
#22823=ORIENTED_EDGE('',*,*,#17188,.F.);
#22824=ORIENTED_EDGE('',*,*,#17222,.T.);
#22825=ORIENTED_EDGE('',*,*,#17223,.T.);
#22826=ORIENTED_EDGE('',*,*,#17224,.F.);
#22827=ORIENTED_EDGE('',*,*,#17189,.T.);
#22828=ORIENTED_EDGE('',*,*,#17225,.T.);
#22829=ORIENTED_EDGE('',*,*,#17226,.T.);
#22830=ORIENTED_EDGE('',*,*,#17204,.F.);
#22831=ORIENTED_EDGE('',*,*,#17197,.F.);
#22832=ORIENTED_EDGE('',*,*,#17227,.T.);
#22833=ORIENTED_EDGE('',*,*,#17225,.F.);
#22834=ORIENTED_EDGE('',*,*,#17196,.T.);
#22835=ORIENTED_EDGE('',*,*,#17228,.T.);
#22836=ORIENTED_EDGE('',*,*,#17228,.F.);
#22837=ORIENTED_EDGE('',*,*,#17195,.F.);
#22838=ORIENTED_EDGE('',*,*,#17229,.T.);
#22839=ORIENTED_EDGE('',*,*,#17230,.T.);
#22840=ORIENTED_EDGE('',*,*,#17231,.T.);
#22841=ORIENTED_EDGE('',*,*,#16983,.F.);
#22842=ORIENTED_EDGE('',*,*,#17193,.T.);
#22843=ORIENTED_EDGE('',*,*,#17232,.T.);
#22844=ORIENTED_EDGE('',*,*,#17192,.T.);
#22845=ORIENTED_EDGE('',*,*,#17233,.T.);
#22846=ORIENTED_EDGE('',*,*,#17234,.F.);
#22847=ORIENTED_EDGE('',*,*,#17232,.F.);
#22848=ORIENTED_EDGE('',*,*,#17235,.T.);
#22849=ORIENTED_EDGE('',*,*,#17233,.F.);
#22850=ORIENTED_EDGE('',*,*,#17191,.T.);
#22851=ORIENTED_EDGE('',*,*,#17236,.T.);
#22852=ORIENTED_EDGE('',*,*,#17190,.T.);
#22853=ORIENTED_EDGE('',*,*,#17224,.T.);
#22854=ORIENTED_EDGE('',*,*,#17237,.F.);
#22855=ORIENTED_EDGE('',*,*,#17236,.F.);
#22856=ORIENTED_EDGE('',*,*,#17068,.T.);
#22857=ORIENTED_EDGE('',*,*,#17025,.T.);
#22858=ORIENTED_EDGE('',*,*,#17030,.T.);
#22859=ORIENTED_EDGE('',*,*,#17238,.T.);
#22860=ORIENTED_EDGE('',*,*,#17239,.F.);
#22861=ORIENTED_EDGE('',*,*,#17240,.F.);
#22862=ORIENTED_EDGE('',*,*,#17028,.T.);
#22863=ORIENTED_EDGE('',*,*,#17241,.T.);
#22864=ORIENTED_EDGE('',*,*,#17242,.T.);
#22865=ORIENTED_EDGE('',*,*,#17238,.F.);
#22866=ORIENTED_EDGE('',*,*,#17032,.T.);
#22867=ORIENTED_EDGE('',*,*,#17038,.T.);
#22868=ORIENTED_EDGE('',*,*,#17243,.T.);
#22869=ORIENTED_EDGE('',*,*,#17244,.F.);
#22870=ORIENTED_EDGE('',*,*,#17241,.F.);
#22871=ORIENTED_EDGE('',*,*,#17034,.T.);
#22872=ORIENTED_EDGE('',*,*,#17046,.T.);
#22873=ORIENTED_EDGE('',*,*,#17245,.T.);
#22874=ORIENTED_EDGE('',*,*,#17246,.F.);
#22875=ORIENTED_EDGE('',*,*,#17247,.F.);
#22876=ORIENTED_EDGE('',*,*,#17036,.T.);
#22877=ORIENTED_EDGE('',*,*,#17247,.T.);
#22878=ORIENTED_EDGE('',*,*,#17248,.T.);
#22879=ORIENTED_EDGE('',*,*,#17243,.F.);
#22880=ORIENTED_EDGE('',*,*,#17040,.T.);
#22881=ORIENTED_EDGE('',*,*,#17249,.T.);
#22882=ORIENTED_EDGE('',*,*,#17250,.F.);
#22883=ORIENTED_EDGE('',*,*,#17245,.F.);
#22884=ORIENTED_EDGE('',*,*,#17043,.T.);
#22885=ORIENTED_EDGE('',*,*,#17251,.T.);
#22886=ORIENTED_EDGE('',*,*,#17252,.F.);
#22887=ORIENTED_EDGE('',*,*,#17249,.F.);
#22888=ORIENTED_EDGE('',*,*,#17045,.T.);
#22889=ORIENTED_EDGE('',*,*,#17048,.T.);
#22890=ORIENTED_EDGE('',*,*,#17253,.T.);
#22891=ORIENTED_EDGE('',*,*,#17254,.F.);
#22892=ORIENTED_EDGE('',*,*,#17251,.F.);
#22893=ORIENTED_EDGE('',*,*,#17050,.T.);
#22894=ORIENTED_EDGE('',*,*,#17052,.T.);
#22895=ORIENTED_EDGE('',*,*,#17255,.T.);
#22896=ORIENTED_EDGE('',*,*,#17256,.T.);
#22897=ORIENTED_EDGE('',*,*,#17253,.F.);
#22898=ORIENTED_EDGE('',*,*,#17054,.T.);
#22899=ORIENTED_EDGE('',*,*,#17257,.T.);
#22900=ORIENTED_EDGE('',*,*,#17258,.F.);
#22901=ORIENTED_EDGE('',*,*,#17255,.F.);
#22902=ORIENTED_EDGE('',*,*,#17056,.T.);
#22903=ORIENTED_EDGE('',*,*,#17062,.T.);
#22904=ORIENTED_EDGE('',*,*,#17259,.F.);
#22905=ORIENTED_EDGE('',*,*,#17257,.F.);
#22906=ORIENTED_EDGE('',*,*,#17260,.T.);
#22907=ORIENTED_EDGE('',*,*,#17229,.F.);
#22908=ORIENTED_EDGE('',*,*,#17194,.T.);
#22909=ORIENTED_EDGE('',*,*,#17023,.T.);
#22910=ORIENTED_EDGE('',*,*,#17070,.T.);
#22911=ORIENTED_EDGE('',*,*,#17240,.T.);
#22912=ORIENTED_EDGE('',*,*,#17261,.T.);
#22913=ORIENTED_EDGE('',*,*,#17065,.F.);
#22914=ORIENTED_EDGE('',*,*,#17006,.T.);
#22915=ORIENTED_EDGE('',*,*,#17262,.T.);
#22916=ORIENTED_EDGE('',*,*,#17263,.F.);
#22917=ORIENTED_EDGE('',*,*,#17073,.F.);
#22918=ORIENTED_EDGE('',*,*,#17078,.F.);
#22919=ORIENTED_EDGE('',*,*,#17083,.F.);
#22920=ORIENTED_EDGE('',*,*,#17263,.T.);
#22921=ORIENTED_EDGE('',*,*,#17264,.F.);
#22922=ORIENTED_EDGE('',*,*,#16991,.F.);
#22923=ORIENTED_EDGE('',*,*,#17075,.F.);
#22924=ORIENTED_EDGE('',*,*,#17265,.F.);
#22925=ORIENTED_EDGE('',*,*,#17266,.T.);
#22926=ORIENTED_EDGE('',*,*,#17267,.T.);
#22927=ORIENTED_EDGE('',*,*,#17268,.T.);
#22928=ORIENTED_EDGE('',*,*,#17269,.T.);
#22929=ORIENTED_EDGE('',*,*,#17270,.T.);
#22930=ORIENTED_EDGE('',*,*,#17266,.F.);
#22931=ORIENTED_EDGE('',*,*,#17271,.F.);
#22932=ORIENTED_EDGE('',*,*,#17272,.T.);
#22933=ORIENTED_EDGE('',*,*,#17273,.T.);
#22934=ORIENTED_EDGE('',*,*,#17269,.F.);
#22935=ORIENTED_EDGE('',*,*,#17274,.F.);
#22936=ORIENTED_EDGE('',*,*,#16750,.T.);
#22937=ORIENTED_EDGE('',*,*,#17275,.T.);
#22938=ORIENTED_EDGE('',*,*,#17272,.F.);
#22939=ORIENTED_EDGE('',*,*,#17276,.F.);
#22940=ORIENTED_EDGE('',*,*,#16730,.T.);
#22941=ORIENTED_EDGE('',*,*,#16674,.F.);
#22942=ORIENTED_EDGE('',*,*,#17276,.T.);
#22943=ORIENTED_EDGE('',*,*,#17274,.T.);
#22944=ORIENTED_EDGE('',*,*,#17271,.T.);
#22945=ORIENTED_EDGE('',*,*,#17265,.T.);
#22946=ORIENTED_EDGE('',*,*,#17277,.F.);
#22947=ORIENTED_EDGE('',*,*,#17277,.T.);
#22948=ORIENTED_EDGE('',*,*,#17278,.F.);
#22949=ORIENTED_EDGE('',*,*,#17279,.F.);
#22950=ORIENTED_EDGE('',*,*,#17280,.F.);
#22951=ORIENTED_EDGE('',*,*,#17281,.F.);
#22952=ORIENTED_EDGE('',*,*,#17282,.T.);
#22953=ORIENTED_EDGE('',*,*,#16731,.F.);
#22954=ORIENTED_EDGE('',*,*,#16732,.T.);
#22955=ORIENTED_EDGE('',*,*,#17282,.F.);
#22956=ORIENTED_EDGE('',*,*,#17283,.F.);
#22957=ORIENTED_EDGE('',*,*,#17284,.T.);
#22958=ORIENTED_EDGE('',*,*,#17284,.F.);
#22959=ORIENTED_EDGE('',*,*,#17285,.F.);
#22960=ORIENTED_EDGE('',*,*,#17286,.F.);
#22961=ORIENTED_EDGE('',*,*,#17287,.F.);
#22962=ORIENTED_EDGE('',*,*,#16733,.T.);
#22963=ORIENTED_EDGE('',*,*,#17287,.T.);
#22964=ORIENTED_EDGE('',*,*,#17288,.F.);
#22965=ORIENTED_EDGE('',*,*,#17289,.F.);
#22966=ORIENTED_EDGE('',*,*,#17290,.F.);
#22967=ORIENTED_EDGE('',*,*,#16726,.F.);
#22968=ORIENTED_EDGE('',*,*,#16727,.T.);
#22969=ORIENTED_EDGE('',*,*,#17290,.T.);
#22970=ORIENTED_EDGE('',*,*,#17291,.F.);
#22971=ORIENTED_EDGE('',*,*,#17292,.F.);
#22972=ORIENTED_EDGE('',*,*,#17293,.T.);
#22973=ORIENTED_EDGE('',*,*,#17294,.T.);
#22974=ORIENTED_EDGE('',*,*,#17295,.F.);
#22975=ORIENTED_EDGE('',*,*,#16728,.T.);
#22976=ORIENTED_EDGE('',*,*,#17295,.T.);
#22977=ORIENTED_EDGE('',*,*,#17296,.T.);
#22978=ORIENTED_EDGE('',*,*,#17297,.T.);
#22979=ORIENTED_EDGE('',*,*,#17298,.F.);
#22980=ORIENTED_EDGE('',*,*,#16729,.F.);
#22981=ORIENTED_EDGE('',*,*,#17298,.T.);
#22982=ORIENTED_EDGE('',*,*,#17299,.T.);
#22983=ORIENTED_EDGE('',*,*,#17300,.T.);
#22984=ORIENTED_EDGE('',*,*,#16672,.T.);
#22985=ORIENTED_EDGE('',*,*,#17301,.T.);
#22986=ORIENTED_EDGE('',*,*,#17302,.T.);
#22987=ORIENTED_EDGE('',*,*,#16749,.F.);
#22988=ORIENTED_EDGE('',*,*,#17300,.F.);
#22989=ORIENTED_EDGE('',*,*,#17303,.T.);
#22990=ORIENTED_EDGE('',*,*,#17304,.T.);
#22991=ORIENTED_EDGE('',*,*,#17301,.F.);
#22992=ORIENTED_EDGE('',*,*,#17299,.F.);
#22993=ORIENTED_EDGE('',*,*,#17305,.T.);
#22994=ORIENTED_EDGE('',*,*,#17306,.T.);
#22995=ORIENTED_EDGE('',*,*,#17303,.F.);
#22996=ORIENTED_EDGE('',*,*,#17297,.F.);
#22997=ORIENTED_EDGE('',*,*,#17307,.T.);
#22998=ORIENTED_EDGE('',*,*,#17308,.T.);
#22999=ORIENTED_EDGE('',*,*,#17305,.F.);
#23000=ORIENTED_EDGE('',*,*,#17296,.F.);
#23001=ORIENTED_EDGE('',*,*,#17309,.T.);
#23002=ORIENTED_EDGE('',*,*,#17310,.T.);
#23003=ORIENTED_EDGE('',*,*,#17307,.F.);
#23004=ORIENTED_EDGE('',*,*,#17294,.F.);
#23005=ORIENTED_EDGE('',*,*,#17311,.T.);
#23006=ORIENTED_EDGE('',*,*,#17309,.F.);
#23007=ORIENTED_EDGE('',*,*,#17293,.F.);
#23008=ORIENTED_EDGE('',*,*,#17312,.T.);
#23009=ORIENTED_EDGE('',*,*,#17312,.F.);
#23010=ORIENTED_EDGE('',*,*,#17292,.T.);
#23011=ORIENTED_EDGE('',*,*,#17313,.T.);
#23012=ORIENTED_EDGE('',*,*,#17314,.F.);
#23013=ORIENTED_EDGE('',*,*,#17291,.T.);
#23014=ORIENTED_EDGE('',*,*,#17315,.T.);
#23015=ORIENTED_EDGE('',*,*,#17316,.F.);
#23016=ORIENTED_EDGE('',*,*,#17313,.F.);
#23017=ORIENTED_EDGE('',*,*,#17289,.T.);
#23018=ORIENTED_EDGE('',*,*,#17317,.T.);
#23019=ORIENTED_EDGE('',*,*,#17318,.F.);
#23020=ORIENTED_EDGE('',*,*,#17315,.F.);
#23021=ORIENTED_EDGE('',*,*,#17288,.T.);
#23022=ORIENTED_EDGE('',*,*,#17319,.T.);
#23023=ORIENTED_EDGE('',*,*,#17320,.F.);
#23024=ORIENTED_EDGE('',*,*,#17317,.F.);
#23025=ORIENTED_EDGE('',*,*,#17286,.T.);
#23026=ORIENTED_EDGE('',*,*,#17321,.T.);
#23027=ORIENTED_EDGE('',*,*,#17322,.F.);
#23028=ORIENTED_EDGE('',*,*,#17319,.F.);
#23029=ORIENTED_EDGE('',*,*,#17285,.T.);
#23030=ORIENTED_EDGE('',*,*,#17323,.T.);
#23031=ORIENTED_EDGE('',*,*,#17324,.F.);
#23032=ORIENTED_EDGE('',*,*,#17321,.F.);
#23033=ORIENTED_EDGE('',*,*,#17283,.T.);
#23034=ORIENTED_EDGE('',*,*,#17325,.T.);
#23035=ORIENTED_EDGE('',*,*,#17323,.F.);
#23036=ORIENTED_EDGE('',*,*,#17281,.T.);
#23037=ORIENTED_EDGE('',*,*,#17326,.T.);
#23038=ORIENTED_EDGE('',*,*,#17327,.F.);
#23039=ORIENTED_EDGE('',*,*,#17325,.F.);
#23040=ORIENTED_EDGE('',*,*,#17280,.T.);
#23041=ORIENTED_EDGE('',*,*,#17328,.T.);
#23042=ORIENTED_EDGE('',*,*,#17329,.F.);
#23043=ORIENTED_EDGE('',*,*,#17326,.F.);
#23044=ORIENTED_EDGE('',*,*,#17279,.T.);
#23045=ORIENTED_EDGE('',*,*,#17330,.T.);
#23046=ORIENTED_EDGE('',*,*,#17331,.F.);
#23047=ORIENTED_EDGE('',*,*,#17328,.F.);
#23048=ORIENTED_EDGE('',*,*,#17268,.F.);
#23049=ORIENTED_EDGE('',*,*,#17332,.F.);
#23050=ORIENTED_EDGE('',*,*,#17330,.F.);
#23051=ORIENTED_EDGE('',*,*,#17278,.T.);
#23052=ORIENTED_EDGE('',*,*,#17332,.T.);
#23053=ORIENTED_EDGE('',*,*,#17333,.T.);
#23054=ORIENTED_EDGE('',*,*,#17334,.T.);
#23055=ORIENTED_EDGE('',*,*,#17335,.T.);
#23056=ORIENTED_EDGE('',*,*,#17336,.F.);
#23057=ORIENTED_EDGE('',*,*,#17337,.T.);
#23058=ORIENTED_EDGE('',*,*,#17338,.F.);
#23059=ORIENTED_EDGE('',*,*,#17334,.F.);
#23060=ORIENTED_EDGE('',*,*,#17333,.F.);
#23061=ORIENTED_EDGE('',*,*,#17267,.F.);
#23062=ORIENTED_EDGE('',*,*,#17339,.T.);
#23063=ORIENTED_EDGE('',*,*,#17340,.F.);
#23064=ORIENTED_EDGE('',*,*,#17337,.F.);
#23065=ORIENTED_EDGE('',*,*,#17270,.F.);
#23066=ORIENTED_EDGE('',*,*,#17341,.T.);
#23067=ORIENTED_EDGE('',*,*,#17342,.F.);
#23068=ORIENTED_EDGE('',*,*,#17339,.F.);
#23069=ORIENTED_EDGE('',*,*,#17273,.F.);
#23070=ORIENTED_EDGE('',*,*,#17343,.T.);
#23071=ORIENTED_EDGE('',*,*,#17344,.T.);
#23072=ORIENTED_EDGE('',*,*,#17341,.F.);
#23073=ORIENTED_EDGE('',*,*,#17275,.F.);
#23074=ORIENTED_EDGE('',*,*,#17302,.F.);
#23075=ORIENTED_EDGE('',*,*,#17345,.T.);
#23076=ORIENTED_EDGE('',*,*,#17346,.T.);
#23077=ORIENTED_EDGE('',*,*,#17343,.F.);
#23078=ORIENTED_EDGE('',*,*,#17304,.F.);
#23079=ORIENTED_EDGE('',*,*,#17306,.F.);
#23080=ORIENTED_EDGE('',*,*,#17347,.T.);
#23081=ORIENTED_EDGE('',*,*,#17348,.F.);
#23082=ORIENTED_EDGE('',*,*,#17345,.F.);
#23083=ORIENTED_EDGE('',*,*,#17308,.F.);
#23084=ORIENTED_EDGE('',*,*,#17310,.F.);
#23085=ORIENTED_EDGE('',*,*,#17349,.T.);
#23086=ORIENTED_EDGE('',*,*,#17350,.F.);
#23087=ORIENTED_EDGE('',*,*,#17347,.F.);
#23088=ORIENTED_EDGE('',*,*,#17311,.F.);
#23089=ORIENTED_EDGE('',*,*,#17314,.T.);
#23090=ORIENTED_EDGE('',*,*,#17351,.T.);
#23091=ORIENTED_EDGE('',*,*,#17352,.T.);
#23092=ORIENTED_EDGE('',*,*,#17349,.F.);
#23093=ORIENTED_EDGE('',*,*,#17316,.T.);
#23094=ORIENTED_EDGE('',*,*,#17318,.T.);
#23095=ORIENTED_EDGE('',*,*,#17353,.T.);
#23096=ORIENTED_EDGE('',*,*,#17354,.T.);
#23097=ORIENTED_EDGE('',*,*,#17351,.F.);
#23098=ORIENTED_EDGE('',*,*,#17320,.T.);
#23099=ORIENTED_EDGE('',*,*,#17322,.T.);
#23100=ORIENTED_EDGE('',*,*,#17355,.T.);
#23101=ORIENTED_EDGE('',*,*,#17356,.F.);
#23102=ORIENTED_EDGE('',*,*,#17353,.F.);
#23103=ORIENTED_EDGE('',*,*,#17324,.T.);
#23104=ORIENTED_EDGE('',*,*,#17327,.T.);
#23105=ORIENTED_EDGE('',*,*,#17357,.T.);
#23106=ORIENTED_EDGE('',*,*,#17358,.F.);
#23107=ORIENTED_EDGE('',*,*,#17355,.F.);
#23108=ORIENTED_EDGE('',*,*,#17329,.T.);
#23109=ORIENTED_EDGE('',*,*,#17359,.T.);
#23110=ORIENTED_EDGE('',*,*,#17360,.T.);
#23111=ORIENTED_EDGE('',*,*,#17357,.F.);
#23112=ORIENTED_EDGE('',*,*,#17331,.T.);
#23113=ORIENTED_EDGE('',*,*,#17336,.T.);
#23114=ORIENTED_EDGE('',*,*,#17361,.T.);
#23115=ORIENTED_EDGE('',*,*,#17359,.F.);
#23116=ORIENTED_EDGE('',*,*,#17362,.F.);
#23117=ORIENTED_EDGE('',*,*,#17363,.F.);
#23118=ORIENTED_EDGE('',*,*,#17364,.F.);
#23119=ORIENTED_EDGE('',*,*,#17365,.F.);
#23120=ORIENTED_EDGE('',*,*,#17366,.T.);
#23121=ORIENTED_EDGE('',*,*,#17367,.T.);
#23122=ORIENTED_EDGE('',*,*,#17368,.T.);
#23123=ORIENTED_EDGE('',*,*,#17013,.F.);
#23124=ORIENTED_EDGE('',*,*,#17015,.T.);
#23125=ORIENTED_EDGE('',*,*,#16745,.F.);
#23126=ORIENTED_EDGE('',*,*,#17002,.F.);
#23127=ORIENTED_EDGE('',*,*,#16999,.F.);
#23128=ORIENTED_EDGE('',*,*,#16995,.F.);
#23129=ORIENTED_EDGE('',*,*,#16988,.T.);
#23130=ORIENTED_EDGE('',*,*,#16992,.F.);
#23131=ORIENTED_EDGE('',*,*,#17264,.T.);
#23132=ORIENTED_EDGE('',*,*,#17262,.F.);
#23133=ORIENTED_EDGE('',*,*,#17005,.T.);
#23134=ORIENTED_EDGE('',*,*,#17086,.F.);
#23135=ORIENTED_EDGE('',*,*,#17087,.F.);
#23136=ORIENTED_EDGE('',*,*,#17009,.F.);
#23137=ORIENTED_EDGE('',*,*,#17354,.F.);
#23138=ORIENTED_EDGE('',*,*,#17356,.T.);
#23139=ORIENTED_EDGE('',*,*,#17358,.T.);
#23140=ORIENTED_EDGE('',*,*,#17360,.F.);
#23141=ORIENTED_EDGE('',*,*,#17361,.F.);
#23142=ORIENTED_EDGE('',*,*,#17335,.F.);
#23143=ORIENTED_EDGE('',*,*,#17338,.T.);
#23144=ORIENTED_EDGE('',*,*,#17340,.T.);
#23145=ORIENTED_EDGE('',*,*,#17342,.T.);
#23146=ORIENTED_EDGE('',*,*,#17344,.F.);
#23147=ORIENTED_EDGE('',*,*,#17346,.F.);
#23148=ORIENTED_EDGE('',*,*,#17348,.T.);
#23149=ORIENTED_EDGE('',*,*,#17350,.T.);
#23150=ORIENTED_EDGE('',*,*,#17352,.F.);
#23151=ORIENTED_EDGE('',*,*,#17250,.T.);
#23152=ORIENTED_EDGE('',*,*,#17252,.T.);
#23153=ORIENTED_EDGE('',*,*,#17254,.T.);
#23154=ORIENTED_EDGE('',*,*,#17256,.F.);
#23155=ORIENTED_EDGE('',*,*,#17258,.T.);
#23156=ORIENTED_EDGE('',*,*,#17259,.T.);
#23157=ORIENTED_EDGE('',*,*,#17061,.T.);
#23158=ORIENTED_EDGE('',*,*,#17066,.T.);
#23159=ORIENTED_EDGE('',*,*,#17261,.F.);
#23160=ORIENTED_EDGE('',*,*,#17239,.T.);
#23161=ORIENTED_EDGE('',*,*,#17242,.F.);
#23162=ORIENTED_EDGE('',*,*,#17244,.T.);
#23163=ORIENTED_EDGE('',*,*,#17248,.F.);
#23164=ORIENTED_EDGE('',*,*,#17246,.T.);
#23165=ORIENTED_EDGE('',*,*,#17369,.F.);
#23166=ORIENTED_EDGE('',*,*,#17370,.F.);
#23167=ORIENTED_EDGE('',*,*,#17363,.T.);
#23168=ORIENTED_EDGE('',*,*,#17371,.T.);
#23169=ORIENTED_EDGE('',*,*,#17372,.F.);
#23170=ORIENTED_EDGE('',*,*,#17364,.T.);
#23171=ORIENTED_EDGE('',*,*,#17370,.T.);
#23172=ORIENTED_EDGE('',*,*,#17373,.F.);
#23173=ORIENTED_EDGE('',*,*,#17374,.F.);
#23174=ORIENTED_EDGE('',*,*,#17365,.T.);
#23175=ORIENTED_EDGE('',*,*,#17372,.T.);
#23176=ORIENTED_EDGE('',*,*,#17375,.F.);
#23177=ORIENTED_EDGE('',*,*,#17376,.T.);
#23178=ORIENTED_EDGE('',*,*,#17377,.F.);
#23179=ORIENTED_EDGE('',*,*,#17366,.F.);
#23180=ORIENTED_EDGE('',*,*,#17374,.T.);
#23181=ORIENTED_EDGE('',*,*,#17378,.T.);
#23182=ORIENTED_EDGE('',*,*,#17379,.F.);
#23183=ORIENTED_EDGE('',*,*,#17367,.F.);
#23184=ORIENTED_EDGE('',*,*,#17377,.T.);
#23185=ORIENTED_EDGE('',*,*,#17368,.F.);
#23186=ORIENTED_EDGE('',*,*,#17379,.T.);
#23187=ORIENTED_EDGE('',*,*,#17380,.T.);
#23188=ORIENTED_EDGE('',*,*,#17381,.F.);
#23189=ORIENTED_EDGE('',*,*,#17382,.T.);
#23190=ORIENTED_EDGE('',*,*,#17371,.F.);
#23191=ORIENTED_EDGE('',*,*,#17362,.T.);
#23192=ORIENTED_EDGE('',*,*,#17381,.T.);
#23193=ORIENTED_EDGE('',*,*,#16753,.T.);
#23194=ORIENTED_EDGE('',*,*,#17019,.F.);
#23195=ORIENTED_EDGE('',*,*,#17214,.F.);
#23196=ORIENTED_EDGE('',*,*,#17212,.T.);
#23197=ORIENTED_EDGE('',*,*,#17210,.F.);
#23198=ORIENTED_EDGE('',*,*,#17208,.T.);
#23199=ORIENTED_EDGE('',*,*,#17205,.F.);
#23200=ORIENTED_EDGE('',*,*,#17226,.F.);
#23201=ORIENTED_EDGE('',*,*,#17227,.F.);
#23202=ORIENTED_EDGE('',*,*,#17230,.F.);
#23203=ORIENTED_EDGE('',*,*,#17260,.F.);
#23204=ORIENTED_EDGE('',*,*,#17022,.F.);
#23205=ORIENTED_EDGE('',*,*,#16984,.T.);
#23206=ORIENTED_EDGE('',*,*,#17231,.F.);
#23207=ORIENTED_EDGE('',*,*,#17234,.T.);
#23208=ORIENTED_EDGE('',*,*,#17235,.F.);
#23209=ORIENTED_EDGE('',*,*,#17237,.T.);
#23210=ORIENTED_EDGE('',*,*,#17223,.F.);
#23211=ORIENTED_EDGE('',*,*,#17221,.F.);
#23212=ORIENTED_EDGE('',*,*,#17219,.F.);
#23213=ORIENTED_EDGE('',*,*,#17216,.F.);
#23214=ORIENTED_EDGE('',*,*,#17218,.F.);
#23215=ORIENTED_EDGE('',*,*,#17206,.T.);
#23216=ORIENTED_EDGE('',*,*,#17380,.F.);
#23217=ORIENTED_EDGE('',*,*,#17378,.F.);
#23218=ORIENTED_EDGE('',*,*,#17376,.F.);
#23219=ORIENTED_EDGE('',*,*,#17375,.T.);
#23220=ORIENTED_EDGE('',*,*,#17373,.T.);
#23221=ORIENTED_EDGE('',*,*,#17369,.T.);
#23222=ORIENTED_EDGE('',*,*,#17382,.F.);
#32032=ADVANCED_FACE('',(#3284),#2522,.T.);
#32033=ADVANCED_FACE('',(#3285,#1254,#1255,#1256),#2084,.T.);
#32034=ADVANCED_FACE('',(#3286),#862,.T.);
#32035=ADVANCED_FACE('',(#3287),#710,.T.);
#32036=ADVANCED_FACE('',(#3288),#2085,.T.);
#32037=ADVANCED_FACE('',(#3289),#863,.T.);
#32038=ADVANCED_FACE('',(#3290),#2523,.F.);
#32039=ADVANCED_FACE('',(#3291),#2086,.T.);
#32040=ADVANCED_FACE('',(#3292),#2524,.F.);
#32041=ADVANCED_FACE('',(#3293),#864,.T.);
#32042=ADVANCED_FACE('',(#3294),#865,.F.);
#32043=ADVANCED_FACE('',(#3295),#866,.T.);
#32044=ADVANCED_FACE('',(#3296),#867,.T.);
#32045=ADVANCED_FACE('',(#3297),#868,.T.);
#32046=ADVANCED_FACE('',(#3298),#2525,.F.);
#32047=ADVANCED_FACE('',(#3299),#2526,.F.);
#32048=ADVANCED_FACE('',(#3300),#869,.F.);
#32049=ADVANCED_FACE('',(#3301),#2527,.F.);
#32050=ADVANCED_FACE('',(#3302),#870,.F.);
#32051=ADVANCED_FACE('',(#3303),#871,.F.);
#32052=ADVANCED_FACE('',(#3304),#872,.F.);
#32053=ADVANCED_FACE('',(#3305),#873,.T.);
#32054=ADVANCED_FACE('',(#3306),#874,.F.);
#32055=ADVANCED_FACE('',(#3307),#2528,.F.);
#32056=ADVANCED_FACE('',(#3308),#2087,.F.);
#32057=ADVANCED_FACE('',(#3309),#2529,.T.);
#32058=ADVANCED_FACE('',(#3310),#66,.T.);
#32059=ADVANCED_FACE('',(#3311),#67,.T.);
#32060=ADVANCED_FACE('',(#3312),#2530,.T.);
#32061=ADVANCED_FACE('',(#3313),#2531,.T.);
#32062=ADVANCED_FACE('',(#3314),#2088,.T.);
#32063=ADVANCED_FACE('',(#3315),#68,.T.);
#32064=ADVANCED_FACE('',(#3316),#2532,.F.);
#32065=ADVANCED_FACE('',(#3317),#2533,.T.);
#32066=ADVANCED_FACE('',(#3318),#2089,.T.);
#32067=ADVANCED_FACE('',(#3319),#69,.T.);
#32068=ADVANCED_FACE('',(#3320),#2534,.F.);
#32069=ADVANCED_FACE('',(#3321),#2535,.T.);
#32070=ADVANCED_FACE('',(#3322),#2090,.F.);
#32071=ADVANCED_FACE('',(#3323),#70,.T.);
#32072=ADVANCED_FACE('',(#3324),#2536,.T.);
#32073=ADVANCED_FACE('',(#3325),#71,.T.);
#32074=ADVANCED_FACE('',(#3326),#2537,.T.);
#32075=ADVANCED_FACE('',(#3327),#72,.T.);
#32076=ADVANCED_FACE('',(#3328),#2538,.T.);
#32077=ADVANCED_FACE('',(#3329),#2539,.T.);
#32078=ADVANCED_FACE('',(#3330),#2091,.F.);
#32079=ADVANCED_FACE('',(#3331),#73,.T.);
#32080=ADVANCED_FACE('',(#3332),#2540,.T.);
#32081=ADVANCED_FACE('',(#3333),#74,.T.);
#32082=ADVANCED_FACE('',(#3334),#2541,.T.);
#32083=ADVANCED_FACE('',(#3335),#75,.T.);
#32084=ADVANCED_FACE('',(#3336),#2542,.T.);
#32085=ADVANCED_FACE('',(#3337),#2543,.T.);
#32086=ADVANCED_FACE('',(#3338),#2092,.T.);
#32087=ADVANCED_FACE('',(#3339),#76,.T.);
#32088=ADVANCED_FACE('',(#3340),#2544,.F.);
#32089=ADVANCED_FACE('',(#3341),#2545,.T.);
#32090=ADVANCED_FACE('',(#3342),#2093,.F.);
#32091=ADVANCED_FACE('',(#3343),#77,.T.);
#32092=ADVANCED_FACE('',(#3344),#2546,.F.);
#32093=ADVANCED_FACE('',(#3345),#2547,.T.);
#32094=ADVANCED_FACE('',(#3346),#2094,.F.);
#32095=ADVANCED_FACE('',(#3347),#78,.T.);
#32096=ADVANCED_FACE('',(#3348),#2548,.T.);
#32097=ADVANCED_FACE('',(#3349),#2549,.T.);
#32098=ADVANCED_FACE('',(#3350),#79,.T.);
#32099=ADVANCED_FACE('',(#3351),#80,.T.);
#32100=ADVANCED_FACE('',(#3352),#2550,.T.);
#32101=ADVANCED_FACE('',(#3353),#2551,.T.);
#32102=ADVANCED_FACE('',(#3354),#2095,.T.);
#32103=ADVANCED_FACE('',(#3355),#81,.T.);
#32104=ADVANCED_FACE('',(#3356),#2552,.F.);
#32105=ADVANCED_FACE('',(#3357),#2553,.T.);
#32106=ADVANCED_FACE('',(#3358),#2096,.T.);
#32107=ADVANCED_FACE('',(#3359),#82,.T.);
#32108=ADVANCED_FACE('',(#3360),#2554,.F.);
#32109=ADVANCED_FACE('',(#3361),#2555,.T.);
#32110=ADVANCED_FACE('',(#3362),#2097,.F.);
#32111=ADVANCED_FACE('',(#3363),#83,.T.);
#32112=ADVANCED_FACE('',(#3364),#2556,.T.);
#32113=ADVANCED_FACE('',(#3365),#84,.T.);
#32114=ADVANCED_FACE('',(#3366),#2557,.T.);
#32115=ADVANCED_FACE('',(#3367),#85,.T.);
#32116=ADVANCED_FACE('',(#3368),#2558,.T.);
#32117=ADVANCED_FACE('',(#3369),#2559,.T.);
#32118=ADVANCED_FACE('',(#3370),#2098,.T.);
#32119=ADVANCED_FACE('',(#3371),#86,.T.);
#32120=ADVANCED_FACE('',(#3372),#2560,.T.);
#32121=ADVANCED_FACE('',(#3373),#87,.T.);
#32122=ADVANCED_FACE('',(#3374),#2561,.T.);
#32123=ADVANCED_FACE('',(#3375),#88,.T.);
#32124=ADVANCED_FACE('',(#3376),#2562,.T.);
#32125=ADVANCED_FACE('',(#3377),#2563,.T.);
#32126=ADVANCED_FACE('',(#3378),#2099,.T.);
#32127=ADVANCED_FACE('',(#3379),#89,.T.);
#32128=ADVANCED_FACE('',(#3380),#2564,.F.);
#32129=ADVANCED_FACE('',(#3381),#2565,.T.);
#32130=ADVANCED_FACE('',(#3382),#2100,.F.);
#32131=ADVANCED_FACE('',(#3383),#90,.T.);
#32132=ADVANCED_FACE('',(#3384),#2566,.T.);
#32133=ADVANCED_FACE('',(#3385),#91,.T.);
#32134=ADVANCED_FACE('',(#3386),#2567,.F.);
#32135=ADVANCED_FACE('',(#3387),#2568,.T.);
#32136=ADVANCED_FACE('',(#3388),#2101,.F.);
#32137=ADVANCED_FACE('',(#3389),#2102,.F.);
#32138=ADVANCED_FACE('',(#3390),#875,.T.);
#32139=ADVANCED_FACE('',(#3391),#2103,.T.);
#32140=ADVANCED_FACE('',(#3392),#876,.T.);
#32141=ADVANCED_FACE('',(#3393),#877,.T.);
#32142=ADVANCED_FACE('',(#3394),#878,.T.);
#32143=ADVANCED_FACE('',(#3395),#879,.T.);
#32144=ADVANCED_FACE('',(#3396),#880,.T.);
#32145=ADVANCED_FACE('',(#3397),#881,.T.);
#32146=ADVANCED_FACE('',(#3398),#882,.T.);
#32147=ADVANCED_FACE('',(#3399),#2104,.F.);
#32148=ADVANCED_FACE('',(#3400),#2105,.T.);
#32149=ADVANCED_FACE('',(#3401),#883,.F.);
#32150=ADVANCED_FACE('',(#3402),#884,.F.);
#32151=ADVANCED_FACE('',(#3403),#885,.F.);
#32152=ADVANCED_FACE('',(#3404),#2569,.T.);
#32153=ADVANCED_FACE('',(#3405),#886,.F.);
#32154=ADVANCED_FACE('',(#3406),#887,.F.);
#32155=ADVANCED_FACE('',(#3407),#888,.F.);
#32156=ADVANCED_FACE('',(#3408),#889,.F.);
#32157=ADVANCED_FACE('',(#3409),#890,.F.);
#32158=ADVANCED_FACE('',(#3410),#891,.F.);
#32159=ADVANCED_FACE('',(#3411),#892,.F.);
#32160=ADVANCED_FACE('',(#3412),#893,.T.);
#32161=ADVANCED_FACE('',(#3413),#894,.T.);
#32162=ADVANCED_FACE('',(#3414),#895,.F.);
#32163=ADVANCED_FACE('',(#3415),#896,.F.);
#32164=ADVANCED_FACE('',(#3416),#897,.F.);
#32165=ADVANCED_FACE('',(#3417),#898,.F.);
#32166=ADVANCED_FACE('',(#3418),#899,.F.);
#32167=ADVANCED_FACE('',(#3419),#900,.F.);
#32168=ADVANCED_FACE('',(#3420),#901,.F.);
#32169=ADVANCED_FACE('',(#3421),#902,.F.);
#32170=ADVANCED_FACE('',(#3422),#903,.F.);
#32171=ADVANCED_FACE('',(#3423),#904,.F.);
#32172=ADVANCED_FACE('',(#3424),#905,.F.);
#32173=ADVANCED_FACE('',(#3425),#906,.T.);
#32174=ADVANCED_FACE('',(#3426),#907,.T.);
#32175=ADVANCED_FACE('',(#3427),#908,.T.);
#32176=ADVANCED_FACE('',(#3428),#909,.T.);
#32177=ADVANCED_FACE('',(#3429),#910,.T.);
#32178=ADVANCED_FACE('',(#3430),#911,.T.);
#32179=ADVANCED_FACE('',(#3431),#912,.T.);
#32180=ADVANCED_FACE('',(#3432),#913,.T.);
#32181=ADVANCED_FACE('',(#3433),#914,.T.);
#32182=ADVANCED_FACE('',(#3434),#915,.T.);
#32183=ADVANCED_FACE('',(#3435),#916,.T.);
#32184=ADVANCED_FACE('',(#3436),#917,.T.);
#32185=ADVANCED_FACE('',(#3437),#918,.T.);
#32186=ADVANCED_FACE('',(#3438),#919,.T.);
#32187=ADVANCED_FACE('',(#3439),#920,.F.);
#32188=ADVANCED_FACE('',(#3440),#921,.F.);
#32189=ADVANCED_FACE('',(#3441),#922,.T.);
#32190=ADVANCED_FACE('',(#3442),#923,.T.);
#32191=ADVANCED_FACE('',(#3443),#924,.T.);
#32192=ADVANCED_FACE('',(#3444),#925,.T.);
#32193=ADVANCED_FACE('',(#3445),#926,.T.);
#32194=ADVANCED_FACE('',(#3446),#927,.T.);
#32195=ADVANCED_FACE('',(#3447),#928,.T.);
#32196=ADVANCED_FACE('',(#3448),#2570,.T.);
#32197=ADVANCED_FACE('',(#3449),#92,.T.);
#32198=ADVANCED_FACE('',(#3450),#93,.T.);
#32199=ADVANCED_FACE('',(#3451),#2571,.T.);
#32200=ADVANCED_FACE('',(#3452),#94,.T.);
#32201=ADVANCED_FACE('',(#3453),#2572,.T.);
#32202=ADVANCED_FACE('',(#3454),#95,.T.);
#32203=ADVANCED_FACE('',(#3455),#2573,.T.);
#32204=ADVANCED_FACE('',(#3456),#96,.T.);
#32205=ADVANCED_FACE('',(#3457),#97,.T.);
#32206=ADVANCED_FACE('',(#3458),#98,.T.);
#32207=ADVANCED_FACE('',(#3459),#2574,.T.);
#32208=ADVANCED_FACE('',(#3460),#99,.T.);
#32209=ADVANCED_FACE('',(#3461),#100,.T.);
#32210=ADVANCED_FACE('',(#3462),#101,.T.);
#32211=ADVANCED_FACE('',(#3463),#2575,.T.);
#32212=ADVANCED_FACE('',(#3464),#102,.T.);
#32213=ADVANCED_FACE('',(#3465),#2576,.T.);
#32214=ADVANCED_FACE('',(#3466),#103,.T.);
#32215=ADVANCED_FACE('',(#3467),#2577,.T.);
#32216=ADVANCED_FACE('',(#3468),#104,.T.);
#32217=ADVANCED_FACE('',(#3469),#105,.T.);
#32218=ADVANCED_FACE('',(#3470),#106,.T.);
#32219=ADVANCED_FACE('',(#3471),#2578,.T.);
#32220=ADVANCED_FACE('',(#3472),#107,.T.);
#32221=ADVANCED_FACE('',(#3473),#2579,.T.);
#32222=ADVANCED_FACE('',(#3474),#108,.T.);
#32223=ADVANCED_FACE('',(#3475),#2580,.T.);
#32224=ADVANCED_FACE('',(#3476),#109,.T.);
#32225=ADVANCED_FACE('',(#3477),#110,.T.);
#32226=ADVANCED_FACE('',(#3478),#111,.T.);
#32227=ADVANCED_FACE('',(#3479),#2581,.T.);
#32228=ADVANCED_FACE('',(#3480),#112,.T.);
#32229=ADVANCED_FACE('',(#3481),#113,.T.);
#32230=ADVANCED_FACE('',(#3482),#114,.T.);
#32231=ADVANCED_FACE('',(#3483),#2582,.T.);
#32232=ADVANCED_FACE('',(#3484),#115,.T.);
#32233=ADVANCED_FACE('',(#3485),#2583,.T.);
#32234=ADVANCED_FACE('',(#3486),#116,.T.);
#32235=ADVANCED_FACE('',(#3487),#117,.T.);
#32236=ADVANCED_FACE('',(#3488),#2584,.T.);
#32237=ADVANCED_FACE('',(#3489,#1257),#2106,.F.);
#32238=ADVANCED_FACE('',(#3490),#2585,.F.);
#32239=ADVANCED_FACE('',(#3491),#2107,.T.);
#32240=ADVANCED_FACE('',(#3492),#2108,.T.);
#32241=ADVANCED_FACE('',(#3493),#2586,.T.);
#32242=ADVANCED_FACE('',(#3494),#2109,.T.);
#32243=ADVANCED_FACE('',(#3495),#2587,.T.);
#32244=ADVANCED_FACE('',(#3496),#2110,.F.);
#32245=ADVANCED_FACE('',(#3497),#2588,.T.);
#32246=ADVANCED_FACE('',(#3498),#2589,.T.);
#32247=ADVANCED_FACE('',(#3499),#2111,.F.);
#32248=ADVANCED_FACE('',(#3500),#2590,.F.);
#32249=ADVANCED_FACE('',(#3501),#2112,.F.);
#32250=ADVANCED_FACE('',(#3502),#2591,.T.);
#32251=ADVANCED_FACE('',(#3503),#2113,.F.);
#32252=ADVANCED_FACE('',(#3504),#2592,.T.);
#32253=ADVANCED_FACE('',(#3505),#2114,.T.);
#32254=ADVANCED_FACE('',(#3506),#2593,.T.);
#32255=ADVANCED_FACE('',(#3507),#2115,.T.);
#32256=ADVANCED_FACE('',(#3508),#929,.F.);
#32257=ADVANCED_FACE('',(#3509),#930,.F.);
#32258=ADVANCED_FACE('',(#3510),#2116,.F.);
#32259=ADVANCED_FACE('',(#3511),#931,.F.);
#32260=ADVANCED_FACE('',(#3512),#932,.F.);
#32261=ADVANCED_FACE('',(#3513),#933,.F.);
#32262=ADVANCED_FACE('',(#3514),#934,.F.);
#32263=ADVANCED_FACE('',(#3515),#935,.F.);
#32264=ADVANCED_FACE('',(#3516),#936,.F.);
#32265=ADVANCED_FACE('',(#3517),#937,.F.);
#32266=ADVANCED_FACE('',(#3518),#938,.F.);
#32267=ADVANCED_FACE('',(#3519),#2594,.T.);
#32268=ADVANCED_FACE('',(#3520),#939,.F.);
#32269=ADVANCED_FACE('',(#3521),#940,.T.);
#32270=ADVANCED_FACE('',(#3522),#941,.T.);
#32271=ADVANCED_FACE('',(#3523),#942,.T.);
#32272=ADVANCED_FACE('',(#3524),#943,.T.);
#32273=ADVANCED_FACE('',(#3525),#944,.T.);
#32274=ADVANCED_FACE('',(#3526),#945,.T.);
#32275=ADVANCED_FACE('',(#3527),#2595,.F.);
#32276=ADVANCED_FACE('',(#3528),#2596,.F.);
#32277=ADVANCED_FACE('',(#3529),#2597,.T.);
#32278=ADVANCED_FACE('',(#3530),#2117,.T.);
#32279=ADVANCED_FACE('',(#3531),#2598,.F.);
#32280=ADVANCED_FACE('',(#3532),#2599,.F.);
#32281=ADVANCED_FACE('',(#3533),#2600,.F.);
#32282=ADVANCED_FACE('',(#3534),#2118,.F.);
#32283=ADVANCED_FACE('',(#3535),#946,.T.);
#32284=ADVANCED_FACE('',(#3536),#947,.T.);
#32285=ADVANCED_FACE('',(#3537),#948,.T.);
#32286=ADVANCED_FACE('',(#3538),#949,.T.);
#32287=ADVANCED_FACE('',(#3539),#950,.T.);
#32288=ADVANCED_FACE('',(#3540),#951,.T.);
#32289=ADVANCED_FACE('',(#3541),#952,.F.);
#32290=ADVANCED_FACE('',(#3542),#953,.F.);
#32291=ADVANCED_FACE('',(#3543),#954,.F.);
#32292=ADVANCED_FACE('',(#3544),#955,.F.);
#32293=ADVANCED_FACE('',(#3545),#956,.F.);
#32294=ADVANCED_FACE('',(#3546),#957,.F.);
#32295=ADVANCED_FACE('',(#3547),#711,.T.);
#32296=ADVANCED_FACE('',(#3548),#958,.F.);
#32297=ADVANCED_FACE('',(#3549),#959,.F.);
#32298=ADVANCED_FACE('',(#3550),#960,.F.);
#32299=ADVANCED_FACE('',(#3551),#961,.F.);
#32300=ADVANCED_FACE('',(#3552),#962,.F.);
#32301=ADVANCED_FACE('',(#3553),#963,.T.);
#32302=ADVANCED_FACE('',(#3554),#964,.T.);
#32303=ADVANCED_FACE('',(#3555),#965,.T.);
#32304=ADVANCED_FACE('',(#3556),#966,.T.);
#32305=ADVANCED_FACE('',(#3557),#967,.T.);
#32306=ADVANCED_FACE('',(#3558),#968,.T.);
#32307=ADVANCED_FACE('',(#3559),#969,.T.);
#32308=ADVANCED_FACE('',(#3560),#970,.F.);
#32309=ADVANCED_FACE('',(#3561),#971,.F.);
#32310=ADVANCED_FACE('',(#3562),#972,.F.);
#32311=ADVANCED_FACE('',(#3563),#973,.F.);
#32312=ADVANCED_FACE('',(#3564),#974,.F.);
#32313=ADVANCED_FACE('',(#3565),#975,.F.);
#32314=ADVANCED_FACE('',(#3566,#1258,#1259,#1260),#2119,.F.);
#32315=ADVANCED_FACE('',(#3567),#2601,.T.);
#32316=ADVANCED_FACE('',(#3568),#2602,.T.);
#32317=ADVANCED_FACE('',(#3569),#2603,.T.);
#32318=ADVANCED_FACE('',(#3570),#2604,.T.);
#32319=ADVANCED_FACE('',(#3571),#2605,.T.);
#32320=ADVANCED_FACE('',(#3572),#2606,.T.);
#32321=ADVANCED_FACE('',(#3573),#2607,.T.);
#32322=ADVANCED_FACE('',(#3574,#1261),#2120,.F.);
#34168=CLOSED_SHELL('',(#32032,#32033,#32034,#32035,#32036,#32037,#32038,
#32039,#32040,#32041,#32042,#32043,#32044,#32045,#32046,#32047,#32048,#32049,
#32050,#32051,#32052,#32053,#32054,#32055,#32056,#32057,#32058,#32059,#32060,
#32061,#32062,#32063,#32064,#32065,#32066,#32067,#32068,#32069,#32070,#32071,
#32072,#32073,#32074,#32075,#32076,#32077,#32078,#32079,#32080,#32081,#32082,
#32083,#32084,#32085,#32086,#32087,#32088,#32089,#32090,#32091,#32092,#32093,
#32094,#32095,#32096,#32097,#32098,#32099,#32100,#32101,#32102,#32103,#32104,
#32105,#32106,#32107,#32108,#32109,#32110,#32111,#32112,#32113,#32114,#32115,
#32116,#32117,#32118,#32119,#32120,#32121,#32122,#32123,#32124,#32125,#32126,
#32127,#32128,#32129,#32130,#32131,#32132,#32133,#32134,#32135,#32136,#32137,
#32138,#32139,#32140,#32141,#32142,#32143,#32144,#32145,#32146,#32147,#32148,
#32149,#32150,#32151,#32152,#32153,#32154,#32155,#32156,#32157,#32158,#32159,
#32160,#32161,#32162,#32163,#32164,#32165,#32166,#32167,#32168,#32169,#32170,
#32171,#32172,#32173,#32174,#32175,#32176,#32177,#32178,#32179,#32180,#32181,
#32182,#32183,#32184,#32185,#32186,#32187,#32188,#32189,#32190,#32191,#32192,
#32193,#32194,#32195,#32196,#32197,#32198,#32199,#32200,#32201,#32202,#32203,
#32204,#32205,#32206,#32207,#32208,#32209,#32210,#32211,#32212,#32213,#32214,
#32215,#32216,#32217,#32218,#32219,#32220,#32221,#32222,#32223,#32224,#32225,
#32226,#32227,#32228,#32229,#32230,#32231,#32232,#32233,#32234,#32235,#32236,
#32237,#32238,#32239,#32240,#32241,#32242,#32243,#32244,#32245,#32246,#32247,
#32248,#32249,#32250,#32251,#32252,#32253,#32254,#32255,#32256,#32257,#32258,
#32259,#32260,#32261,#32262,#32263,#32264,#32265,#32266,#32267,#32268,#32269,
#32270,#32271,#32272,#32273,#32274,#32275,#32276,#32277,#32278,#32279,#32280,
#32281,#32282,#32283,#32284,#32285,#32286,#32287,#32288,#32289,#32290,#32291,
#32292,#32293,#32294,#32295,#32296,#32297,#32298,#32299,#32300,#32301,#32302,
#32303,#32304,#32305,#32306,#32307,#32308,#32309,#32310,#32311,#32312,#32313,
#32314,#32315,#32316,#32317,#32318,#32319,#32320,#32321,#32322));
#34303=AXIS2_PLACEMENT_3D('',#49130,#38645,#38646);
#34304=AXIS2_PLACEMENT_3D('',#49131,#38647,#38648);
#34305=AXIS2_PLACEMENT_3D('',#49136,#38650,#38651);
#34306=AXIS2_PLACEMENT_3D('',#49139,#38653,#38654);
#34307=AXIS2_PLACEMENT_3D('',#49140,#38655,#38656);
#34308=AXIS2_PLACEMENT_3D('',#49145,#38658,#38659);
#34309=AXIS2_PLACEMENT_3D('',#49147,#38660,#38661);
#34310=AXIS2_PLACEMENT_3D('',#49149,#38662,#38663);
#34311=AXIS2_PLACEMENT_3D('',#49153,#38665,#38666);
#34312=AXIS2_PLACEMENT_3D('',#49157,#38668,#38669);
#34313=AXIS2_PLACEMENT_3D('',#49161,#38671,#38672);
#34314=AXIS2_PLACEMENT_3D('',#49163,#38673,#38674);
#34315=AXIS2_PLACEMENT_3D('',#49165,#38675,#38676);
#34316=AXIS2_PLACEMENT_3D('',#49169,#38678,#38679);
#34317=AXIS2_PLACEMENT_3D('',#49173,#38681,#38682);
#34318=AXIS2_PLACEMENT_3D('',#49177,#38684,#38685);
#34319=AXIS2_PLACEMENT_3D('',#49179,#38686,#38687);
#34320=AXIS2_PLACEMENT_3D('',#49181,#38688,#38689);
#34321=AXIS2_PLACEMENT_3D('',#49185,#38691,#38692);
#34322=AXIS2_PLACEMENT_3D('',#49187,#38693,#38694);
#34323=AXIS2_PLACEMENT_3D('',#49189,#38695,#38696);
#34324=AXIS2_PLACEMENT_3D('',#49193,#38698,#38699);
#34325=AXIS2_PLACEMENT_3D('',#49197,#38701,#38702);
#34326=AXIS2_PLACEMENT_3D('',#49201,#38704,#38705);
#34327=AXIS2_PLACEMENT_3D('',#49203,#38706,#38707);
#34328=AXIS2_PLACEMENT_3D('',#49205,#38708,#38709);
#34329=AXIS2_PLACEMENT_3D('',#49209,#38711,#38712);
#34330=AXIS2_PLACEMENT_3D('',#49213,#38714,#38715);
#34331=AXIS2_PLACEMENT_3D('',#49217,#38717,#38718);
#34332=AXIS2_PLACEMENT_3D('',#49219,#38719,#38720);
#34333=AXIS2_PLACEMENT_3D('',#49220,#38721,#38722);
#34334=AXIS2_PLACEMENT_3D('',#49223,#38723,#38724);
#34335=AXIS2_PLACEMENT_3D('',#49271,#38725,#38726);
#34336=AXIS2_PLACEMENT_3D('',#49275,#38728,#38729);
#34337=AXIS2_PLACEMENT_3D('',#49286,#38730,#38731);
#34338=AXIS2_PLACEMENT_3D('',#49288,#38732,#38733);
#34339=AXIS2_PLACEMENT_3D('',#49290,#38734,#38735);
#34340=AXIS2_PLACEMENT_3D('',#49293,#38737,#38738);
#34341=AXIS2_PLACEMENT_3D('',#49295,#38739,#38740);
#34342=AXIS2_PLACEMENT_3D('',#49297,#38741,#38742);
#34343=AXIS2_PLACEMENT_3D('',#49303,#38745,#38746);
#34344=AXIS2_PLACEMENT_3D('',#49359,#38747,#38748);
#34345=AXIS2_PLACEMENT_3D('',#49365,#38749,#38750);
#34346=AXIS2_PLACEMENT_3D('',#49453,#38753,#38754);
#34347=AXIS2_PLACEMENT_3D('',#49455,#38755,#38756);
#34348=AXIS2_PLACEMENT_3D('',#49456,#38757,#38758);
#34349=AXIS2_PLACEMENT_3D('',#49457,#38759,#38760);
#34350=AXIS2_PLACEMENT_3D('',#49522,#38767,#38768);
#34351=AXIS2_PLACEMENT_3D('',#49535,#38770,#38771);
#34352=AXIS2_PLACEMENT_3D('',#49536,#38772,#38773);
#34353=AXIS2_PLACEMENT_3D('',#49540,#38776,#38777);
#34354=AXIS2_PLACEMENT_3D('',#49544,#38779,#38780);
#34355=AXIS2_PLACEMENT_3D('',#49586,#38781,#38782);
#34356=AXIS2_PLACEMENT_3D('',#49670,#38784,#38785);
#34357=AXIS2_PLACEMENT_3D('',#49745,#38786,#38787);
#34358=AXIS2_PLACEMENT_3D('',#49872,#38790,#38791);
#34359=AXIS2_PLACEMENT_3D('',#49975,#38794,#38795);
#34360=AXIS2_PLACEMENT_3D('',#49977,#38796,#38797);
#34361=AXIS2_PLACEMENT_3D('',#50020,#38798,#38799);
#34362=AXIS2_PLACEMENT_3D('',#50024,#38801,#38802);
#34363=AXIS2_PLACEMENT_3D('',#50118,#38805,#38806);
#34364=AXIS2_PLACEMENT_3D('',#50164,#38808,#38809);
#34365=AXIS2_PLACEMENT_3D('',#50373,#38813,#38814);
#34366=AXIS2_PLACEMENT_3D('',#50639,#38817,#38818);
#34367=AXIS2_PLACEMENT_3D('',#50784,#38819,#38820);
#34368=AXIS2_PLACEMENT_3D('',#50873,#38821,#38822);
#34369=AXIS2_PLACEMENT_3D('',#50877,#38824,#38825);
#34370=AXIS2_PLACEMENT_3D('',#50919,#38826,#38827);
#34371=AXIS2_PLACEMENT_3D('',#50920,#38828,#38829);
#34372=AXIS2_PLACEMENT_3D('',#50922,#38831,#38832);
#34373=AXIS2_PLACEMENT_3D('',#50925,#38833,#38834);
#34374=AXIS2_PLACEMENT_3D('',#50929,#38836,#38837);
#34375=AXIS2_PLACEMENT_3D('',#50931,#38839,#38840);
#34376=AXIS2_PLACEMENT_3D('',#50932,#38841,#38842);
#34377=AXIS2_PLACEMENT_3D('',#50933,#38843,#38844);
#34378=AXIS2_PLACEMENT_3D('',#50934,#38845,#38846);
#34379=AXIS2_PLACEMENT_3D('',#50936,#38847,#38848);
#34380=AXIS2_PLACEMENT_3D('',#50937,#38849,#38850);
#34381=AXIS2_PLACEMENT_3D('',#50938,#38851,#38852);
#34382=AXIS2_PLACEMENT_3D('',#50941,#38854,#38855);
#34383=AXIS2_PLACEMENT_3D('',#50942,#38856,#38857);
#34384=AXIS2_PLACEMENT_3D('',#50944,#38858,#38859);
#34385=AXIS2_PLACEMENT_3D('',#50946,#38861,#38862);
#34386=AXIS2_PLACEMENT_3D('',#50950,#38865,#38866);
#34387=AXIS2_PLACEMENT_3D('',#50952,#38867,#38868);
#34388=AXIS2_PLACEMENT_3D('',#50953,#38869,#38870);
#34389=AXIS2_PLACEMENT_3D('',#50954,#38871,#38872);
#34390=AXIS2_PLACEMENT_3D('',#50957,#38874,#38875);
#34391=AXIS2_PLACEMENT_3D('',#50958,#38876,#38877);
#34392=AXIS2_PLACEMENT_3D('',#50960,#38878,#38879);
#34393=AXIS2_PLACEMENT_3D('',#50962,#38881,#38882);
#34394=AXIS2_PLACEMENT_3D('',#50966,#38885,#38886);
#34395=AXIS2_PLACEMENT_3D('',#50968,#38887,#38888);
#34396=AXIS2_PLACEMENT_3D('',#50969,#38889,#38890);
#34397=AXIS2_PLACEMENT_3D('',#50970,#38891,#38892);
#34398=AXIS2_PLACEMENT_3D('',#50973,#38894,#38895);
#34399=AXIS2_PLACEMENT_3D('',#50974,#38896,#38897);
#34400=AXIS2_PLACEMENT_3D('',#50976,#38898,#38899);
#34401=AXIS2_PLACEMENT_3D('',#50978,#38901,#38902);
#34402=AXIS2_PLACEMENT_3D('',#50982,#38905,#38906);
#34403=AXIS2_PLACEMENT_3D('',#50984,#38907,#38908);
#34404=AXIS2_PLACEMENT_3D('',#50985,#38909,#38910);
#34405=AXIS2_PLACEMENT_3D('',#50986,#38911,#38912);
#34406=AXIS2_PLACEMENT_3D('',#50989,#38914,#38915);
#34407=AXIS2_PLACEMENT_3D('',#50990,#38916,#38917);
#34408=AXIS2_PLACEMENT_3D('',#50992,#38918,#38919);
#34409=AXIS2_PLACEMENT_3D('',#50993,#38920,#38921);
#34410=AXIS2_PLACEMENT_3D('',#50994,#38922,#38923);
#34411=AXIS2_PLACEMENT_3D('',#50997,#38925,#38926);
#34412=AXIS2_PLACEMENT_3D('',#50998,#38927,#38928);
#34413=AXIS2_PLACEMENT_3D('',#51000,#38929,#38930);
#34414=AXIS2_PLACEMENT_3D('',#51001,#38931,#38932);
#34415=AXIS2_PLACEMENT_3D('',#51002,#38933,#38934);
#34416=AXIS2_PLACEMENT_3D('',#51005,#38936,#38937);
#34417=AXIS2_PLACEMENT_3D('',#51006,#38938,#38939);
#34418=AXIS2_PLACEMENT_3D('',#51008,#38940,#38941);
#34419=AXIS2_PLACEMENT_3D('',#51010,#38943,#38944);
#34420=AXIS2_PLACEMENT_3D('',#51014,#38947,#38948);
#34421=AXIS2_PLACEMENT_3D('',#51016,#38949,#38950);
#34422=AXIS2_PLACEMENT_3D('',#51017,#38951,#38952);
#34423=AXIS2_PLACEMENT_3D('',#51018,#38953,#38954);
#34424=AXIS2_PLACEMENT_3D('',#51021,#38956,#38957);
#34425=AXIS2_PLACEMENT_3D('',#51022,#38958,#38959);
#34426=AXIS2_PLACEMENT_3D('',#51024,#38960,#38961);
#34427=AXIS2_PLACEMENT_3D('',#51025,#38962,#38963);
#34428=AXIS2_PLACEMENT_3D('',#51026,#38964,#38965);
#34429=AXIS2_PLACEMENT_3D('',#51029,#38967,#38968);
#34430=AXIS2_PLACEMENT_3D('',#51030,#38969,#38970);
#34431=AXIS2_PLACEMENT_3D('',#51032,#38971,#38972);
#34432=AXIS2_PLACEMENT_3D('',#51033,#38973,#38974);
#34433=AXIS2_PLACEMENT_3D('',#51034,#38975,#38976);
#34434=AXIS2_PLACEMENT_3D('',#51037,#38978,#38979);
#34435=AXIS2_PLACEMENT_3D('',#51038,#38980,#38981);
#34436=AXIS2_PLACEMENT_3D('',#51040,#38982,#38983);
#34437=AXIS2_PLACEMENT_3D('',#51042,#38985,#38986);
#34438=AXIS2_PLACEMENT_3D('',#51046,#38989,#38990);
#34439=AXIS2_PLACEMENT_3D('',#51048,#38991,#38992);
#34440=AXIS2_PLACEMENT_3D('',#51049,#38993,#38994);
#34441=AXIS2_PLACEMENT_3D('',#51050,#38995,#38996);
#34442=AXIS2_PLACEMENT_3D('',#51053,#38998,#38999);
#34443=AXIS2_PLACEMENT_3D('',#51054,#39000,#39001);
#34444=AXIS2_PLACEMENT_3D('',#51056,#39002,#39003);
#34445=AXIS2_PLACEMENT_3D('',#51058,#39005,#39006);
#34446=AXIS2_PLACEMENT_3D('',#51062,#39009,#39010);
#34447=AXIS2_PLACEMENT_3D('',#51064,#39011,#39012);
#34448=AXIS2_PLACEMENT_3D('',#51065,#39013,#39014);
#34449=AXIS2_PLACEMENT_3D('',#51066,#39015,#39016);
#34450=AXIS2_PLACEMENT_3D('',#51069,#39018,#39019);
#34451=AXIS2_PLACEMENT_3D('',#51070,#39020,#39021);
#34452=AXIS2_PLACEMENT_3D('',#51072,#39022,#39023);
#34453=AXIS2_PLACEMENT_3D('',#51074,#39025,#39026);
#34454=AXIS2_PLACEMENT_3D('',#51078,#39029,#39030);
#34455=AXIS2_PLACEMENT_3D('',#51080,#39031,#39032);
#34456=AXIS2_PLACEMENT_3D('',#51081,#39033,#39034);
#34457=AXIS2_PLACEMENT_3D('',#51082,#39035,#39036);
#34458=AXIS2_PLACEMENT_3D('',#51085,#39038,#39039);
#34459=AXIS2_PLACEMENT_3D('',#51086,#39040,#39041);
#34460=AXIS2_PLACEMENT_3D('',#51088,#39042,#39043);
#34461=AXIS2_PLACEMENT_3D('',#51090,#39044,#39045);
#34462=AXIS2_PLACEMENT_3D('',#51092,#39047,#39048);
#34463=AXIS2_PLACEMENT_3D('',#51093,#39049,#39050);
#34464=AXIS2_PLACEMENT_3D('',#51094,#39051,#39052);
#34465=AXIS2_PLACEMENT_3D('',#51096,#39053,#39054);
#34466=AXIS2_PLACEMENT_3D('',#51097,#39055,#39056);
#34467=AXIS2_PLACEMENT_3D('',#51098,#39057,#39058);
#34468=AXIS2_PLACEMENT_3D('',#51101,#39060,#39061);
#34469=AXIS2_PLACEMENT_3D('',#51102,#39062,#39063);
#34470=AXIS2_PLACEMENT_3D('',#51104,#39064,#39065);
#34471=AXIS2_PLACEMENT_3D('',#51106,#39067,#39068);
#34472=AXIS2_PLACEMENT_3D('',#51110,#39071,#39072);
#34473=AXIS2_PLACEMENT_3D('',#51112,#39073,#39074);
#34474=AXIS2_PLACEMENT_3D('',#51113,#39075,#39076);
#34475=AXIS2_PLACEMENT_3D('',#51114,#39077,#39078);
#34476=AXIS2_PLACEMENT_3D('',#51117,#39080,#39081);
#34477=AXIS2_PLACEMENT_3D('',#51118,#39082,#39083);
#34478=AXIS2_PLACEMENT_3D('',#51120,#39084,#39085);
#34479=AXIS2_PLACEMENT_3D('',#51122,#39087,#39088);
#34480=AXIS2_PLACEMENT_3D('',#51126,#39091,#39092);
#34481=AXIS2_PLACEMENT_3D('',#51128,#39093,#39094);
#34482=AXIS2_PLACEMENT_3D('',#51129,#39095,#39096);
#34483=AXIS2_PLACEMENT_3D('',#51130,#39097,#39098);
#34484=AXIS2_PLACEMENT_3D('',#51133,#39100,#39101);
#34485=AXIS2_PLACEMENT_3D('',#51134,#39102,#39103);
#34486=AXIS2_PLACEMENT_3D('',#51136,#39104,#39105);
#34487=AXIS2_PLACEMENT_3D('',#51138,#39107,#39108);
#34488=AXIS2_PLACEMENT_3D('',#51142,#39111,#39112);
#34489=AXIS2_PLACEMENT_3D('',#51144,#39113,#39114);
#34490=AXIS2_PLACEMENT_3D('',#51145,#39115,#39116);
#34491=AXIS2_PLACEMENT_3D('',#51146,#39117,#39118);
#34492=AXIS2_PLACEMENT_3D('',#51149,#39120,#39121);
#34493=AXIS2_PLACEMENT_3D('',#51150,#39122,#39123);
#34494=AXIS2_PLACEMENT_3D('',#51152,#39124,#39125);
#34495=AXIS2_PLACEMENT_3D('',#51153,#39126,#39127);
#34496=AXIS2_PLACEMENT_3D('',#51154,#39128,#39129);
#34497=AXIS2_PLACEMENT_3D('',#51157,#39131,#39132);
#34498=AXIS2_PLACEMENT_3D('',#51158,#39133,#39134);
#34499=AXIS2_PLACEMENT_3D('',#51160,#39135,#39136);
#34500=AXIS2_PLACEMENT_3D('',#51161,#39137,#39138);
#34501=AXIS2_PLACEMENT_3D('',#51162,#39139,#39140);
#34502=AXIS2_PLACEMENT_3D('',#51165,#39142,#39143);
#34503=AXIS2_PLACEMENT_3D('',#51166,#39144,#39145);
#34504=AXIS2_PLACEMENT_3D('',#51168,#39146,#39147);
#34505=AXIS2_PLACEMENT_3D('',#51170,#39149,#39150);
#34506=AXIS2_PLACEMENT_3D('',#51174,#39153,#39154);
#34507=AXIS2_PLACEMENT_3D('',#51176,#39155,#39156);
#34508=AXIS2_PLACEMENT_3D('',#51177,#39157,#39158);
#34509=AXIS2_PLACEMENT_3D('',#51178,#39159,#39160);
#34510=AXIS2_PLACEMENT_3D('',#51181,#39162,#39163);
#34511=AXIS2_PLACEMENT_3D('',#51182,#39164,#39165);
#34512=AXIS2_PLACEMENT_3D('',#51184,#39166,#39167);
#34513=AXIS2_PLACEMENT_3D('',#51185,#39168,#39169);
#34514=AXIS2_PLACEMENT_3D('',#51186,#39170,#39171);
#34515=AXIS2_PLACEMENT_3D('',#51189,#39173,#39174);
#34516=AXIS2_PLACEMENT_3D('',#51190,#39175,#39176);
#34517=AXIS2_PLACEMENT_3D('',#51192,#39177,#39178);
#34518=AXIS2_PLACEMENT_3D('',#51193,#39179,#39180);
#34519=AXIS2_PLACEMENT_3D('',#51194,#39181,#39182);
#34520=AXIS2_PLACEMENT_3D('',#51197,#39184,#39185);
#34521=AXIS2_PLACEMENT_3D('',#51198,#39186,#39187);
#34522=AXIS2_PLACEMENT_3D('',#51200,#39188,#39189);
#34523=AXIS2_PLACEMENT_3D('',#51202,#39191,#39192);
#34524=AXIS2_PLACEMENT_3D('',#51206,#39195,#39196);
#34525=AXIS2_PLACEMENT_3D('',#51208,#39197,#39198);
#34526=AXIS2_PLACEMENT_3D('',#51209,#39199,#39200);
#34527=AXIS2_PLACEMENT_3D('',#51210,#39201,#39202);
#34528=AXIS2_PLACEMENT_3D('',#51213,#39204,#39205);
#34529=AXIS2_PLACEMENT_3D('',#51214,#39206,#39207);
#34530=AXIS2_PLACEMENT_3D('',#51216,#39208,#39209);
#34531=AXIS2_PLACEMENT_3D('',#51218,#39211,#39212);
#34532=AXIS2_PLACEMENT_3D('',#51222,#39215,#39216);
#34533=AXIS2_PLACEMENT_3D('',#51224,#39217,#39218);
#34534=AXIS2_PLACEMENT_3D('',#51225,#39219,#39220);
#34535=AXIS2_PLACEMENT_3D('',#51226,#39221,#39222);
#34536=AXIS2_PLACEMENT_3D('',#51228,#39223,#39224);
#34537=AXIS2_PLACEMENT_3D('',#51230,#39226,#39227);
#34538=AXIS2_PLACEMENT_3D('',#51232,#39228,#39229);
#34539=AXIS2_PLACEMENT_3D('',#51233,#39230,#39231);
#34540=AXIS2_PLACEMENT_3D('',#51234,#39232,#39233);
#34541=AXIS2_PLACEMENT_3D('',#51237,#39235,#39236);
#34542=AXIS2_PLACEMENT_3D('',#51238,#39237,#39238);
#34543=AXIS2_PLACEMENT_3D('',#51240,#39240,#39241);
#34544=AXIS2_PLACEMENT_3D('',#51242,#39243,#39244);
#34545=AXIS2_PLACEMENT_3D('',#51328,#39251,#39252);
#34546=AXIS2_PLACEMENT_3D('',#51334,#39255,#39256);
#34547=AXIS2_PLACEMENT_3D('',#51367,#39259,#39260);
#34548=AXIS2_PLACEMENT_3D('',#51530,#39263,#39264);
#34549=AXIS2_PLACEMENT_3D('',#51694,#39269,#39270);
#34550=AXIS2_PLACEMENT_3D('',#51817,#39271,#39272);
#34551=AXIS2_PLACEMENT_3D('',#51823,#39276,#39277);
#34552=AXIS2_PLACEMENT_3D('',#51866,#39281,#39282);
#34553=AXIS2_PLACEMENT_3D('',#51899,#39283,#39284);
#34554=AXIS2_PLACEMENT_3D('',#51955,#39285,#39286);
#34555=AXIS2_PLACEMENT_3D('',#51994,#39287,#39288);
#34556=AXIS2_PLACEMENT_3D('',#52041,#39289,#39290);
#34557=AXIS2_PLACEMENT_3D('',#52043,#39291,#39292);
#34558=AXIS2_PLACEMENT_3D('',#52082,#39294,#39295);
#34559=AXIS2_PLACEMENT_3D('',#52084,#39296,#39297);
#34560=AXIS2_PLACEMENT_3D('',#52085,#39298,#39299);
#34561=AXIS2_PLACEMENT_3D('',#52178,#39300,#39301);
#34562=AXIS2_PLACEMENT_3D('',#52215,#39302,#39303);
#34563=AXIS2_PLACEMENT_3D('',#52289,#39304,#39305);
#34564=AXIS2_PLACEMENT_3D('',#52424,#39306,#39307);
#34565=AXIS2_PLACEMENT_3D('',#52480,#39308,#39309);
#34566=AXIS2_PLACEMENT_3D('',#52561,#39310,#39311);
#34567=AXIS2_PLACEMENT_3D('',#52727,#39312,#39313);
#34568=AXIS2_PLACEMENT_3D('',#52793,#39314,#39315);
#34569=AXIS2_PLACEMENT_3D('',#52943,#39316,#39317);
#34570=AXIS2_PLACEMENT_3D('',#53006,#39318,#39319);
#34571=AXIS2_PLACEMENT_3D('',#53099,#39320,#39321);
#34572=AXIS2_PLACEMENT_3D('',#53237,#39322,#39323);
#34573=AXIS2_PLACEMENT_3D('',#53457,#39326,#39327);
#34574=AXIS2_PLACEMENT_3D('',#53538,#39329,#39330);
#34575=AXIS2_PLACEMENT_3D('',#53576,#39331,#39332);
#34576=AXIS2_PLACEMENT_3D('',#53577,#39333,#39334);
#34577=AXIS2_PLACEMENT_3D('',#53651,#39335,#39336);
#34578=AXIS2_PLACEMENT_3D('',#53725,#39337,#39338);
#34579=AXIS2_PLACEMENT_3D('',#53737,#39339,#39340);
#34580=AXIS2_PLACEMENT_3D('',#53801,#39341,#39342);
#34581=AXIS2_PLACEMENT_3D('',#53839,#39343,#39344);
#34582=AXIS2_PLACEMENT_3D('',#53883,#39345,#39346);
#34583=AXIS2_PLACEMENT_3D('',#53884,#39347,#39348);
#34584=AXIS2_PLACEMENT_3D('',#53885,#39349,#39350);
#34585=AXIS2_PLACEMENT_3D('',#53940,#39351,#39352);
#34586=AXIS2_PLACEMENT_3D('',#53977,#39353,#39354);
#34587=AXIS2_PLACEMENT_3D('',#54159,#39356,#39357);
#34588=AXIS2_PLACEMENT_3D('',#54196,#39358,#39359);
#34589=AXIS2_PLACEMENT_3D('',#54269,#39360,#39361);
#34590=AXIS2_PLACEMENT_3D('',#54324,#39362,#39363);
#34591=AXIS2_PLACEMENT_3D('',#54361,#39364,#39365);
#34592=AXIS2_PLACEMENT_3D('',#54416,#39366,#39367);
#34593=AXIS2_PLACEMENT_3D('',#54453,#39368,#39369);
#34594=AXIS2_PLACEMENT_3D('',#54508,#39370,#39371);
#34595=AXIS2_PLACEMENT_3D('',#54563,#39372,#39373);
#34596=AXIS2_PLACEMENT_3D('',#54636,#39374,#39375);
#34597=AXIS2_PLACEMENT_3D('',#54673,#39376,#39377);
#34598=AXIS2_PLACEMENT_3D('',#54710,#39378,#39379);
#34599=AXIS2_PLACEMENT_3D('',#54711,#39380,#39381);
#34600=AXIS2_PLACEMENT_3D('',#54766,#39382,#39383);
#34601=AXIS2_PLACEMENT_3D('',#54803,#39384,#39385);
#34602=AXIS2_PLACEMENT_3D('',#54804,#39386,#39387);
#34603=AXIS2_PLACEMENT_3D('',#54806,#39388,#39389);
#34604=AXIS2_PLACEMENT_3D('',#54808,#39390,#39391);
#34605=AXIS2_PLACEMENT_3D('',#54809,#39392,#39393);
#34606=AXIS2_PLACEMENT_3D('',#54810,#39394,#39395);
#34607=AXIS2_PLACEMENT_3D('',#54812,#39396,#39397);
#34608=AXIS2_PLACEMENT_3D('',#54813,#39398,#39399);
#34609=AXIS2_PLACEMENT_3D('',#54814,#39400,#39401);
#34610=AXIS2_PLACEMENT_3D('',#54816,#39402,#39403);
#34611=AXIS2_PLACEMENT_3D('',#54818,#39405,#39406);
#34612=AXIS2_PLACEMENT_3D('',#54820,#39407,#39408);
#34613=AXIS2_PLACEMENT_3D('',#54821,#39409,#39410);
#34614=AXIS2_PLACEMENT_3D('',#54822,#39411,#39412);
#34615=AXIS2_PLACEMENT_3D('',#54824,#39413,#39414);
#34616=AXIS2_PLACEMENT_3D('',#54826,#39416,#39417);
#34617=AXIS2_PLACEMENT_3D('',#54828,#39418,#39419);
#34618=AXIS2_PLACEMENT_3D('',#54829,#39420,#39421);
#34619=AXIS2_PLACEMENT_3D('',#54830,#39422,#39423);
#34620=AXIS2_PLACEMENT_3D('',#54832,#39424,#39425);
#34621=AXIS2_PLACEMENT_3D('',#54834,#39427,#39428);
#34622=AXIS2_PLACEMENT_3D('',#54836,#39429,#39430);
#34623=AXIS2_PLACEMENT_3D('',#54837,#39431,#39432);
#34624=AXIS2_PLACEMENT_3D('',#54838,#39433,#39434);
#34625=AXIS2_PLACEMENT_3D('',#54840,#39435,#39436);
#34626=AXIS2_PLACEMENT_3D('',#54841,#39437,#39438);
#34627=AXIS2_PLACEMENT_3D('',#54842,#39439,#39440);
#34628=AXIS2_PLACEMENT_3D('',#54844,#39441,#39442);
#34629=AXIS2_PLACEMENT_3D('',#54845,#39443,#39444);
#34630=AXIS2_PLACEMENT_3D('',#54846,#39445,#39446);
#34631=AXIS2_PLACEMENT_3D('',#54848,#39447,#39448);
#34632=AXIS2_PLACEMENT_3D('',#54850,#39450,#39451);
#34633=AXIS2_PLACEMENT_3D('',#54852,#39452,#39453);
#34634=AXIS2_PLACEMENT_3D('',#54853,#39454,#39455);
#34635=AXIS2_PLACEMENT_3D('',#54854,#39456,#39457);
#34636=AXIS2_PLACEMENT_3D('',#54856,#39458,#39459);
#34637=AXIS2_PLACEMENT_3D('',#54857,#39460,#39461);
#34638=AXIS2_PLACEMENT_3D('',#54858,#39462,#39463);
#34639=AXIS2_PLACEMENT_3D('',#54860,#39464,#39465);
#34640=AXIS2_PLACEMENT_3D('',#54861,#39466,#39467);
#34641=AXIS2_PLACEMENT_3D('',#54862,#39468,#39469);
#34642=AXIS2_PLACEMENT_3D('',#54864,#39470,#39471);
#34643=AXIS2_PLACEMENT_3D('',#54866,#39473,#39474);
#34644=AXIS2_PLACEMENT_3D('',#54868,#39475,#39476);
#34645=AXIS2_PLACEMENT_3D('',#54869,#39477,#39478);
#34646=AXIS2_PLACEMENT_3D('',#54870,#39479,#39480);
#34647=AXIS2_PLACEMENT_3D('',#54872,#39481,#39482);
#34648=AXIS2_PLACEMENT_3D('',#54874,#39484,#39485);
#34649=AXIS2_PLACEMENT_3D('',#54876,#39486,#39487);
#34650=AXIS2_PLACEMENT_3D('',#54877,#39488,#39489);
#34651=AXIS2_PLACEMENT_3D('',#54878,#39490,#39491);
#34652=AXIS2_PLACEMENT_3D('',#54880,#39492,#39493);
#34653=AXIS2_PLACEMENT_3D('',#54882,#39495,#39496);
#34654=AXIS2_PLACEMENT_3D('',#54884,#39497,#39498);
#34655=AXIS2_PLACEMENT_3D('',#54885,#39499,#39500);
#34656=AXIS2_PLACEMENT_3D('',#54886,#39501,#39502);
#34657=AXIS2_PLACEMENT_3D('',#54888,#39503,#39504);
#34658=AXIS2_PLACEMENT_3D('',#54889,#39505,#39506);
#34659=AXIS2_PLACEMENT_3D('',#54890,#39507,#39508);
#34660=AXIS2_PLACEMENT_3D('',#54892,#39509,#39510);
#34661=AXIS2_PLACEMENT_3D('',#54893,#39511,#39512);
#34662=AXIS2_PLACEMENT_3D('',#54894,#39513,#39514);
#34663=AXIS2_PLACEMENT_3D('',#54896,#39515,#39516);
#34664=AXIS2_PLACEMENT_3D('',#54898,#39518,#39519);
#34665=AXIS2_PLACEMENT_3D('',#54900,#39520,#39521);
#34666=AXIS2_PLACEMENT_3D('',#54901,#39522,#39523);
#34667=AXIS2_PLACEMENT_3D('',#54902,#39524,#39525);
#34668=AXIS2_PLACEMENT_3D('',#54904,#39526,#39527);
#34669=AXIS2_PLACEMENT_3D('',#54906,#39529,#39530);
#34670=AXIS2_PLACEMENT_3D('',#54908,#39531,#39532);
#34671=AXIS2_PLACEMENT_3D('',#54909,#39533,#39534);
#34672=AXIS2_PLACEMENT_3D('',#54910,#39535,#39536);
#34673=AXIS2_PLACEMENT_3D('',#54912,#39537,#39538);
#34674=AXIS2_PLACEMENT_3D('',#54914,#39540,#39541);
#34675=AXIS2_PLACEMENT_3D('',#54916,#39542,#39543);
#34676=AXIS2_PLACEMENT_3D('',#54917,#39544,#39545);
#34677=AXIS2_PLACEMENT_3D('',#54918,#39546,#39547);
#34678=AXIS2_PLACEMENT_3D('',#54920,#39548,#39549);
#34679=AXIS2_PLACEMENT_3D('',#54921,#39550,#39551);
#34680=AXIS2_PLACEMENT_3D('',#54922,#39552,#39553);
#34681=AXIS2_PLACEMENT_3D('',#54924,#39554,#39555);
#34682=AXIS2_PLACEMENT_3D('',#54925,#39556,#39557);
#34683=AXIS2_PLACEMENT_3D('',#54926,#39558,#39559);
#34684=AXIS2_PLACEMENT_3D('',#54928,#39560,#39561);
#34685=AXIS2_PLACEMENT_3D('',#54930,#39563,#39564);
#34686=AXIS2_PLACEMENT_3D('',#54932,#39565,#39566);
#34687=AXIS2_PLACEMENT_3D('',#54933,#39567,#39568);
#34688=AXIS2_PLACEMENT_3D('',#54934,#39569,#39570);
#34689=AXIS2_PLACEMENT_3D('',#54936,#39571,#39572);
#34690=AXIS2_PLACEMENT_3D('',#54937,#39573,#39574);
#34691=AXIS2_PLACEMENT_3D('',#54938,#39575,#39576);
#34692=AXIS2_PLACEMENT_3D('',#54940,#39577,#39578);
#34693=AXIS2_PLACEMENT_3D('',#54941,#39579,#39580);
#34694=AXIS2_PLACEMENT_3D('',#54942,#39581,#39582);
#34695=AXIS2_PLACEMENT_3D('',#54944,#39583,#39584);
#34696=AXIS2_PLACEMENT_3D('',#54946,#39586,#39587);
#34697=AXIS2_PLACEMENT_3D('',#54948,#39588,#39589);
#34698=AXIS2_PLACEMENT_3D('',#54949,#39590,#39591);
#34699=AXIS2_PLACEMENT_3D('',#54950,#39592,#39593);
#34700=AXIS2_PLACEMENT_3D('',#54952,#39594,#39595);
#34701=AXIS2_PLACEMENT_3D('',#54954,#39597,#39598);
#34702=AXIS2_PLACEMENT_3D('',#54956,#39599,#39600);
#34703=AXIS2_PLACEMENT_3D('',#54957,#39601,#39602);
#34704=AXIS2_PLACEMENT_3D('',#54958,#39603,#39604);
#34705=AXIS2_PLACEMENT_3D('',#54960,#39605,#39606);
#34706=AXIS2_PLACEMENT_3D('',#54961,#39607,#39608);
#34707=AXIS2_PLACEMENT_3D('',#54962,#39609,#39610);
#34708=AXIS2_PLACEMENT_3D('',#54964,#39612,#39613);
#34709=AXIS2_PLACEMENT_3D('',#54968,#39615,#39616);
#34710=AXIS2_PLACEMENT_3D('',#54972,#39618,#39619);
#34711=AXIS2_PLACEMENT_3D('',#54976,#39621,#39622);
#34712=AXIS2_PLACEMENT_3D('',#54980,#39624,#39625);
#34713=AXIS2_PLACEMENT_3D('',#54983,#39627,#39628);
#34714=AXIS2_PLACEMENT_3D('',#54985,#39629,#39630);
#34715=AXIS2_PLACEMENT_3D('',#54989,#39632,#39633);
#34716=AXIS2_PLACEMENT_3D('',#54993,#39635,#39636);
#34717=AXIS2_PLACEMENT_3D('',#54997,#39638,#39639);
#34718=AXIS2_PLACEMENT_3D('',#55000,#39641,#39642);
#34719=AXIS2_PLACEMENT_3D('',#55001,#39643,#39644);
#34720=AXIS2_PLACEMENT_3D('',#55006,#39647,#39648);
#34721=AXIS2_PLACEMENT_3D('',#55007,#39649,#39650);
#34722=AXIS2_PLACEMENT_3D('',#55011,#39653,#39654);
#34723=AXIS2_PLACEMENT_3D('',#55015,#39657,#39658);
#34724=AXIS2_PLACEMENT_3D('',#55017,#39659,#39660);
#34725=AXIS2_PLACEMENT_3D('',#55019,#39662,#39663);
#34726=AXIS2_PLACEMENT_3D('',#55023,#39666,#39667);
#34727=AXIS2_PLACEMENT_3D('',#55024,#39668,#39669);
#34728=AXIS2_PLACEMENT_3D('',#55025,#39670,#39671);
#34729=AXIS2_PLACEMENT_3D('',#55031,#39675,#39676);
#34730=AXIS2_PLACEMENT_3D('',#55032,#39677,#39678);
#34731=AXIS2_PLACEMENT_3D('',#55033,#39679,#39680);
#34732=AXIS2_PLACEMENT_3D('',#55035,#39681,#39682);
#34733=AXIS2_PLACEMENT_3D('',#55037,#39684,#39685);
#34734=AXIS2_PLACEMENT_3D('',#55041,#39688,#39689);
#34735=AXIS2_PLACEMENT_3D('',#55043,#39690,#39691);
#34736=AXIS2_PLACEMENT_3D('',#55045,#39693,#39694);
#34737=AXIS2_PLACEMENT_3D('',#55049,#39697,#39698);
#34738=AXIS2_PLACEMENT_3D('',#55051,#39699,#39700);
#34739=AXIS2_PLACEMENT_3D('',#55053,#39702,#39703);
#34740=AXIS2_PLACEMENT_3D('',#55057,#39706,#39707);
#34741=AXIS2_PLACEMENT_3D('',#55059,#39708,#39709);
#34742=AXIS2_PLACEMENT_3D('',#55061,#39711,#39712);
#34743=AXIS2_PLACEMENT_3D('',#55065,#39715,#39716);
#34744=AXIS2_PLACEMENT_3D('',#55067,#39717,#39718);
#34745=AXIS2_PLACEMENT_3D('',#55069,#39720,#39721);
#34746=AXIS2_PLACEMENT_3D('',#55133,#39726,#39727);
#34747=AXIS2_PLACEMENT_3D('',#55410,#39737,#39738);
#34748=AXIS2_PLACEMENT_3D('',#55502,#39739,#39740);
#34749=AXIS2_PLACEMENT_3D('',#55503,#39741,#39742);
#34750=AXIS2_PLACEMENT_3D('',#55516,#39743,#39744);
#34751=AXIS2_PLACEMENT_3D('',#55738,#39746,#39747);
#34752=AXIS2_PLACEMENT_3D('',#55851,#39748,#39749);
#34753=AXIS2_PLACEMENT_3D('',#55933,#39750,#39751);
#34754=AXIS2_PLACEMENT_3D('',#56065,#39752,#39753);
#34755=AXIS2_PLACEMENT_3D('',#56066,#39754,#39755);
#34756=AXIS2_PLACEMENT_3D('',#56068,#39757,#39758);
#34757=AXIS2_PLACEMENT_3D('',#56156,#39759,#39760);
#34758=AXIS2_PLACEMENT_3D('',#56158,#39762,#39763);
#34759=AXIS2_PLACEMENT_3D('',#56160,#39764,#39765);
#34760=AXIS2_PLACEMENT_3D('',#56162,#39767,#39768);
#34761=AXIS2_PLACEMENT_3D('',#56164,#39769,#39770);
#34762=AXIS2_PLACEMENT_3D('',#56189,#39772,#39773);
#34763=AXIS2_PLACEMENT_3D('',#56191,#39774,#39775);
#34764=AXIS2_PLACEMENT_3D('',#56222,#39777,#39778);
#34765=AXIS2_PLACEMENT_3D('',#56224,#39779,#39780);
#34766=AXIS2_PLACEMENT_3D('',#56328,#39781,#39782);
#34767=AXIS2_PLACEMENT_3D('',#56330,#39784,#39785);
#34768=AXIS2_PLACEMENT_3D('',#56361,#39786,#39787);
#34769=AXIS2_PLACEMENT_3D('',#56363,#39789,#39790);
#34770=AXIS2_PLACEMENT_3D('',#56387,#39791,#39792);
#34771=AXIS2_PLACEMENT_3D('',#56425,#39793,#39794);
#34772=AXIS2_PLACEMENT_3D('',#56469,#39795,#39796);
#34773=AXIS2_PLACEMENT_3D('',#56523,#39797,#39798);
#34774=AXIS2_PLACEMENT_3D('',#56524,#39799,#39800);
#34775=AXIS2_PLACEMENT_3D('',#56580,#39801,#39802);
#34776=AXIS2_PLACEMENT_3D('',#56621,#39803,#39804);
#34777=AXIS2_PLACEMENT_3D('',#56690,#39805,#39806);
#34778=AXIS2_PLACEMENT_3D('',#56746,#39807,#39808);
#34779=AXIS2_PLACEMENT_3D('',#56875,#39809,#39810);
#34780=AXIS2_PLACEMENT_3D('',#56935,#39811,#39812);
#34781=AXIS2_PLACEMENT_3D('',#56995,#39813,#39814);
#34782=AXIS2_PLACEMENT_3D('',#56996,#39815,#39816);
#34783=AXIS2_PLACEMENT_3D('',#57034,#39817,#39818);
#34784=AXIS2_PLACEMENT_3D('',#57076,#39819,#39820);
#34785=AXIS2_PLACEMENT_3D('',#57090,#39821,#39822);
#34786=AXIS2_PLACEMENT_3D('',#57091,#39823,#39824);
#34787=AXIS2_PLACEMENT_3D('',#57147,#39825,#39826);
#34788=AXIS2_PLACEMENT_3D('',#57219,#39827,#39828);
#34789=AXIS2_PLACEMENT_3D('',#57324,#39829,#39830);
#34790=AXIS2_PLACEMENT_3D('',#57688,#39834,#39835);
#34791=AXIS2_PLACEMENT_3D('',#57703,#39837,#39838);
#34792=AXIS2_PLACEMENT_3D('',#57718,#39840,#39841);
#34793=AXIS2_PLACEMENT_3D('',#57753,#39844,#39845);
#34794=AXIS2_PLACEMENT_3D('',#57768,#39847,#39848);
#34795=AXIS2_PLACEMENT_3D('',#57783,#39850,#39851);
#34796=AXIS2_PLACEMENT_3D('',#57798,#39853,#39854);
#34797=AXIS2_PLACEMENT_3D('',#57833,#39857,#39858);
#34798=AXIS2_PLACEMENT_3D('',#57848,#39860,#39861);
#34799=AXIS2_PLACEMENT_3D('',#57861,#39862,#39863);
#34800=AXIS2_PLACEMENT_3D('',#57862,#39864,#39865);
#34801=AXIS2_PLACEMENT_3D('',#57865,#39866,#39867);
#34802=AXIS2_PLACEMENT_3D('',#57867,#39868,#39869);
#34803=AXIS2_PLACEMENT_3D('',#57869,#39870,#39871);
#34804=AXIS2_PLACEMENT_3D('',#57871,#39872,#39873);
#34805=AXIS2_PLACEMENT_3D('',#57873,#39874,#39875);
#34806=AXIS2_PLACEMENT_3D('',#57875,#39876,#39877);
#34807=AXIS2_PLACEMENT_3D('',#57876,#39878,#39879);
#34808=AXIS2_PLACEMENT_3D('',#57877,#39880,#39881);
#34809=AXIS2_PLACEMENT_3D('',#57880,#39882,#39883);
#34810=AXIS2_PLACEMENT_3D('',#57883,#39886,#39887);
#34811=AXIS2_PLACEMENT_3D('',#57886,#39889,#39890);
#34812=AXIS2_PLACEMENT_3D('',#57887,#39891,#39892);
#34813=AXIS2_PLACEMENT_3D('',#57890,#39894,#39895);
#34814=AXIS2_PLACEMENT_3D('',#57891,#39896,#39897);
#34815=AXIS2_PLACEMENT_3D('',#57893,#39898,#39899);
#34816=AXIS2_PLACEMENT_3D('',#57895,#39901,#39902);
#34817=AXIS2_PLACEMENT_3D('',#57897,#39903,#39904);
#34818=AXIS2_PLACEMENT_3D('',#57899,#39906,#39907);
#34819=AXIS2_PLACEMENT_3D('',#57901,#39908,#39909);
#34820=AXIS2_PLACEMENT_3D('',#57903,#39911,#39912);
#34821=AXIS2_PLACEMENT_3D('',#57904,#39913,#39914);
#34822=AXIS2_PLACEMENT_3D('',#57905,#39915,#39916);
#38645=DIRECTION('axis',(0.,0.,1.));
#38646=DIRECTION('refdir',(1.,0.,0.));
#38647=DIRECTION('center_axis',(2.44929359829375E-16,1.,-1.22464679914625E-16));
#38648=DIRECTION('ref_axis',(0.70655827709904,-8.63941405564051E-17,0.707654860128041));
#38649=DIRECTION('',(0.,-1.,0.));
#38650=DIRECTION('center_axis',(-1.56278055360592E-9,-1.,3.44451669369109E-9));
#38651=DIRECTION('ref_axis',(0.706558277096871,1.33333344365384E-9,0.707654860130206));
#38652=DIRECTION('',(-2.96059473233E-16,-1.,0.));
#38653=DIRECTION('center_axis',(-2.44929359829E-16,-1.,1.22464679915E-16));
#38654=DIRECTION('ref_axis',(1.,-2.44929359829E-16,2.99951956532444E-32));
#38655=DIRECTION('center_axis',(-2.44929359829E-16,-1.,1.22464679915E-16));
#38656=DIRECTION('ref_axis',(-1.,2.44929359829E-16,0.));
#38657=DIRECTION('',(3.9900198549E-16,0.,-1.));
#38658=DIRECTION('center_axis',(-2.44929359829E-16,-1.,1.22464679915E-16));
#38659=DIRECTION('ref_axis',(1.,-2.44929359829E-16,2.99951956532444E-32));
#38660=DIRECTION('center_axis',(-2.44929359829E-16,-1.,1.22464679915E-16));
#38661=DIRECTION('ref_axis',(1.,-2.44929359829E-16,5.91180967883826E-34));
#38662=DIRECTION('center_axis',(-2.44929359829E-16,-1.,1.22464679915E-16));
#38663=DIRECTION('ref_axis',(1.,-2.44929359829E-16,2.99951956532443E-32));
#38664=DIRECTION('',(0.716064653814028,0.,0.698033961608027));
#38665=DIRECTION('center_axis',(2.44929359829E-16,1.,-1.22464679915E-16));
#38666=DIRECTION('ref_axis',(1.,-2.44929359829E-16,2.99951956532444E-32));
#38667=DIRECTION('',(0.698033961608027,-4.30707715433016E-16,-0.716064653814028));
#38668=DIRECTION('center_axis',(2.44929359829E-16,1.,-1.22464679915E-16));
#38669=DIRECTION('ref_axis',(1.,-2.44929359829E-16,2.99951956532444E-32));
#38670=DIRECTION('',(-0.716064653814028,0.,-0.698033961608027));
#38671=DIRECTION('center_axis',(-2.44929359829E-16,-1.,1.22464679915E-16));
#38672=DIRECTION('ref_axis',(1.,-2.44929359829E-16,2.99951956532443E-32));
#38673=DIRECTION('center_axis',(-2.44929359829E-16,-1.,1.22464679915E-16));
#38674=DIRECTION('ref_axis',(1.,-2.44929359829E-16,5.91180967883826E-34));
#38675=DIRECTION('center_axis',(-2.44929359829E-16,-1.,1.22464679915E-16));
#38676=DIRECTION('ref_axis',(1.,-2.44929359829E-16,2.99951956532443E-32));
#38677=DIRECTION('',(-0.716064653814028,2.5912401877601E-16,0.698033961608027));
#38678=DIRECTION('center_axis',(2.44929359829E-16,1.,-1.22464679915E-16));
#38679=DIRECTION('ref_axis',(1.,-2.44929359829E-16,2.99951956532444E-32));
#38680=DIRECTION('',(0.698033961608027,0.,0.716064653814028));
#38681=DIRECTION('center_axis',(2.44929359829E-16,1.,-1.22464679915E-16));
#38682=DIRECTION('ref_axis',(1.,-2.44929359829E-16,2.99951956532444E-32));
#38683=DIRECTION('',(0.716064653814028,-2.6102542122301E-16,-0.698033961608027));
#38684=DIRECTION('center_axis',(-2.44929359829E-16,-1.,1.22464679915E-16));
#38685=DIRECTION('ref_axis',(1.,-2.44929359829E-16,2.99951956532443E-32));
#38686=DIRECTION('center_axis',(-2.44929359829E-16,-1.,1.22464679915E-16));
#38687=DIRECTION('ref_axis',(1.,-2.44929359829E-16,6.68589598176748E-33));
#38688=DIRECTION('center_axis',(-2.44929359829E-16,-1.,1.22464679915E-16));
#38689=DIRECTION('ref_axis',(1.,-2.44929359829E-16,2.99951956532444E-32));
#38690=DIRECTION('',(-3.9900198549E-16,0.,1.));
#38691=DIRECTION('center_axis',(-2.44929359829E-16,-1.,1.22464679915E-16));
#38692=DIRECTION('ref_axis',(1.,-2.44929359829E-16,2.99951956532444E-32));
#38693=DIRECTION('center_axis',(-2.44929359829E-16,-1.,1.22464679915E-16));
#38694=DIRECTION('ref_axis',(1.,-2.44929359829E-16,-2.37876790876508E-32));
#38695=DIRECTION('center_axis',(-2.44929359829E-16,-1.,1.22464679915E-16));
#38696=DIRECTION('ref_axis',(1.,-2.44929359829E-16,2.99951956532443E-32));
#38697=DIRECTION('',(-0.716064653814028,0.,-0.698033961608027));
#38698=DIRECTION('center_axis',(2.44929359829E-16,1.,-1.22464679915E-16));
#38699=DIRECTION('ref_axis',(1.,-2.44929359829E-16,2.99951956532444E-32));
#38700=DIRECTION('',(-0.698033961608027,4.30707715433016E-16,0.716064653814028));
#38701=DIRECTION('center_axis',(2.44929359829E-16,1.,-1.22464679915E-16));
#38702=DIRECTION('ref_axis',(1.,-2.44929359829E-16,2.99951956532444E-32));
#38703=DIRECTION('',(0.716064653814028,0.,0.698033961608027));
#38704=DIRECTION('center_axis',(-2.44929359829E-16,-1.,1.22464679915E-16));
#38705=DIRECTION('ref_axis',(1.,-2.44929359829E-16,2.99951956532443E-32));
#38706=DIRECTION('center_axis',(-2.44929359829E-16,-1.,1.22464679915E-16));
#38707=DIRECTION('ref_axis',(1.,-2.44929359829E-16,5.91180967883826E-34));
#38708=DIRECTION('center_axis',(-2.44929359829E-16,-1.,1.22464679915E-16));
#38709=DIRECTION('ref_axis',(1.,-2.44929359829E-16,2.99951956532443E-32));
#38710=DIRECTION('',(0.716064653814028,-2.6393829599301E-16,-0.698033961608027));
#38711=DIRECTION('center_axis',(2.44929359829E-16,1.,-1.22464679915E-16));
#38712=DIRECTION('ref_axis',(1.,-2.44929359829E-16,2.99951956532443E-32));
#38713=DIRECTION('',(-0.698033961608027,0.,-0.716064653814028));
#38714=DIRECTION('center_axis',(2.44929359829E-16,1.,-1.22464679915E-16));
#38715=DIRECTION('ref_axis',(1.,-2.44929359829E-16,2.99951956532444E-32));
#38716=DIRECTION('',(-0.716064653814028,2.6591127623201E-16,0.698033961608027));
#38717=DIRECTION('center_axis',(-2.44929359829E-16,-1.,1.22464679915E-16));
#38718=DIRECTION('ref_axis',(1.,-2.44929359829E-16,2.99951956532443E-32));
#38719=DIRECTION('center_axis',(-2.44929359829E-16,-1.,1.22464679915E-16));
#38720=DIRECTION('ref_axis',(1.,-2.44929359829E-16,-2.37876790876508E-32));
#38721=DIRECTION('center_axis',(-2.44929359829E-16,-1.,1.22464679915E-16));
#38722=DIRECTION('ref_axis',(1.,-2.44929359829E-16,2.99951956532444E-32));
#38723=DIRECTION('center_axis',(2.44929359829E-16,1.,-1.22464679915E-16));
#38724=DIRECTION('ref_axis',(1.,-2.44929359829E-16,2.99951956532444E-32));
#38725=DIRECTION('center_axis',(2.44929359829E-16,1.,-1.22464679915E-16));
#38726=DIRECTION('ref_axis',(1.,-2.44929359829E-16,2.99951956532443E-32));
#38727=DIRECTION('',(4.20437734738E-16,0.,-1.));
#38728=DIRECTION('center_axis',(2.44929359829E-16,1.,-1.22464679915E-16));
#38729=DIRECTION('ref_axis',(1.,-2.44929359829E-16,2.99951956532443E-32));
#38730=DIRECTION('center_axis',(2.44929359829E-16,1.,-1.22464679915E-16));
#38731=DIRECTION('ref_axis',(1.,-2.44929359829E-16,2.99951956532444E-32));
#38732=DIRECTION('center_axis',(-2.44929359829E-16,-1.,1.22464679915E-16));
#38733=DIRECTION('ref_axis',(1.,-2.44929359829E-16,2.99951956532443E-32));
#38734=DIRECTION('center_axis',(-2.44929359829E-16,-1.,1.22464679915E-16));
#38735=DIRECTION('ref_axis',(1.,-2.44929359829E-16,2.99951956532444E-32));
#38736=DIRECTION('',(-0.0656339938339316,0.,0.99784376475148));
#38737=DIRECTION('center_axis',(-2.44929359829E-16,-1.,1.22464679915E-16));
#38738=DIRECTION('ref_axis',(1.,-2.44929359829E-16,2.99951956532443E-32));
#38739=DIRECTION('center_axis',(2.44929359829E-16,1.,-1.22464679915E-16));
#38740=DIRECTION('ref_axis',(1.,-2.44929359829E-16,2.99951956532443E-32));
#38741=DIRECTION('center_axis',(2.44929359829E-16,1.,-1.22464679915E-16));
#38742=DIRECTION('ref_axis',(1.,-2.44929359829E-16,2.99951956532444E-32));
#38743=DIRECTION('',(0.0656339938339316,0.,0.99784376475148));
#38744=DIRECTION('',(4.20437734738E-16,0.,-1.));
#38745=DIRECTION('center_axis',(-2.44929359829E-16,-1.,1.22464679915E-16));
#38746=DIRECTION('ref_axis',(1.,-2.44929359829E-16,2.99951956532444E-32));
#38747=DIRECTION('center_axis',(-2.44929359829E-16,-1.,1.22464679915E-16));
#38748=DIRECTION('ref_axis',(1.,-2.44929359829E-16,2.99951956532444E-32));
#38749=DIRECTION('center_axis',(-2.44929359829E-16,-1.,1.22464679915E-16));
#38750=DIRECTION('ref_axis',(1.,-2.44929359829E-16,2.99951956532444E-32));
#38751=DIRECTION('',(-0.288070798801296,0.943889906160958,0.161514890723551));
#38752=DIRECTION('',(-0.185892369076962,0.87281982032212,0.451253352754101));
#38753=DIRECTION('center_axis',(0.631948690569006,-0.772532669185509,-0.0619203321150045));
#38754=DIRECTION('ref_axis',(-0.212600461685972,-0.249632918685971,0.944713951203874));
#38755=DIRECTION('center_axis',(-0.0594793302428471,-0.422789452293976,
0.904273901150986));
#38756=DIRECTION('ref_axis',(0.74528916761046,0.583836479538853,0.321992269786383));
#38757=DIRECTION('center_axis',(-0.629470113233292,0.456900095359148,0.628497954974293));
#38758=DIRECTION('ref_axis',(0.745284573628305,0.583834639915972,0.322006238364825));
#38759=DIRECTION('center_axis',(-1.,2.44929359829E-16,-4.93371725307E-16));
#38760=DIRECTION('ref_axis',(-4.93371725307E-16,0.,1.));
#38761=DIRECTION('',(3.93680872405E-16,0.,-1.));
#38762=DIRECTION('',(0.,-1.,0.));
#38763=DIRECTION('',(3.70074341542E-16,0.,-1.));
#38764=DIRECTION('',(0.,-1.,0.));
#38765=DIRECTION('',(2.1147105231E-16,1.,0.));
#38766=DIRECTION('',(4.22942104619E-16,1.,0.));
#38767=DIRECTION('center_axis',(2.44929359829E-16,1.,-1.22464679915E-16));
#38768=DIRECTION('ref_axis',(-1.,2.44929359829E-16,-2.99951956532444E-32));
#38769=DIRECTION('',(2.67621944414E-16,1.,-1.07048777765E-15));
#38770=DIRECTION('center_axis',(-0.455243749742543,-0.0346073179899924,
0.889694027102514));
#38771=DIRECTION('ref_axis',(0.0631992828870565,-0.997979881587316,-0.00648124907159732));
#38772=DIRECTION('center_axis',(1.,-2.44929359829E-16,3.67394039744E-16));
#38773=DIRECTION('ref_axis',(-3.67394039744E-16,0.,1.));
#38774=DIRECTION('',(2.1147105231E-16,1.,0.));
#38775=DIRECTION('',(0.,0.,-1.));
#38776=DIRECTION('center_axis',(2.44929359829009E-16,1.,-1.22464679915049E-16));
#38777=DIRECTION('ref_axis',(0.17719394991793,-1.63926793636935E-16,-0.984175951805612));
#38778=DIRECTION('',(2.96059473233E-16,1.,0.));
#38779=DIRECTION('center_axis',(0.164797595711241,-0.072937415919611,-0.983626903763192));
#38780=DIRECTION('ref_axis',(-0.00994679585199009,0.997088453026087,-0.0756021037691614));
#38781=DIRECTION('center_axis',(-0.996740111917573,-0.0806792990324772,
-1.47358394346062E-6));
#38782=DIRECTION('ref_axis',(0.080679298682933,-0.996740105534059,-0.000113066272843588));
#38783=DIRECTION('',(1.18423789293E-15,1.,-1.48029736617E-16));
#38784=DIRECTION('center_axis',(-0.815291085828504,-0.452356370985093,0.361488808952332));
#38785=DIRECTION('ref_axis',(0.410559632229298,-0.0113482213864199,0.911763130563585));
#38786=DIRECTION('center_axis',(-0.181645839985608,-0.207917305089807,0.961132240152267));
#38787=DIRECTION('ref_axis',(0.0696529687957434,-0.977657575872474,-0.198328334529125));
#38788=DIRECTION('',(1.18423789293E-15,1.,0.));
#38789=DIRECTION('',(0.,1.,0.));
#38790=DIRECTION('center_axis',(0.062548597995711,-0.99472870449491,-0.0812556296058808));
#38791=DIRECTION('ref_axis',(0.441715695037133,0.100598146276716,-0.891497200064897));
#38792=DIRECTION('',(0.,1.,0.));
#38793=DIRECTION('',(4.22942104619E-16,1.,0.));
#38794=DIRECTION('center_axis',(2.44929359828923E-16,1.,-1.22464679914962E-16));
#38795=DIRECTION('ref_axis',(-0.898888448298522,2.73825444514855E-16,0.438177541089767));
#38796=DIRECTION('center_axis',(-0.891374682075179,-0.0362585643310429,
0.451814666282565));
#38797=DIRECTION('ref_axis',(0.0137554448307947,-0.998500150383736,-0.0529928053717017));
#38798=DIRECTION('center_axis',(-2.44929359829E-16,-1.,1.22464679915E-16));
#38799=DIRECTION('ref_axis',(1.,-2.44929359829E-16,2.99951956532444E-32));
#38800=DIRECTION('',(2.96059473233E-16,1.,-5.92118946467E-16));
#38801=DIRECTION('center_axis',(-0.455243749742543,0.0346073179899924,-0.889694027102514));
#38802=DIRECTION('ref_axis',(0.0631992828870565,0.997979881587316,0.00648124907159732));
#38803=DIRECTION('',(2.67621944414E-16,1.,-1.07048777765E-15));
#38804=DIRECTION('',(4.22942104619E-16,1.,0.));
#38805=DIRECTION('center_axis',(-2.44929359828974E-16,-1.,1.22464679915013E-16));
#38806=DIRECTION('ref_axis',(0.898888448298522,-1.66502899883911E-16,0.438177541089767));
#38807=DIRECTION('',(0.,1.,0.));
#38808=DIRECTION('center_axis',(-0.891374682075179,0.0362585643310429,-0.451814666282565));
#38809=DIRECTION('ref_axis',(0.0137554448307947,0.998500150383736,0.0529928053717017));
#38810=DIRECTION('',(0.,1.,0.));
#38811=DIRECTION('',(0.,1.,0.));
#38812=DIRECTION('',(1.18423789293E-15,1.,0.));
#38813=DIRECTION('center_axis',(0.062548597995711,0.99472870449491,0.0812556296058808));
#38814=DIRECTION('ref_axis',(0.441715695037133,-0.100598146276716,0.891497200064897));
#38815=DIRECTION('',(1.18423789293E-15,1.,-1.48029736617E-16));
#38816=DIRECTION('',(2.1147105231E-16,1.,0.));
#38817=DIRECTION('center_axis',(-0.181645839985592,0.207917305090092,-0.961132240152208));
#38818=DIRECTION('ref_axis',(-0.0696529687957387,-0.977657575872416,-0.198328334529416));
#38819=DIRECTION('center_axis',(-0.815291085828504,0.452356370985093,-0.361488808952332));
#38820=DIRECTION('ref_axis',(0.410559632229298,0.0113482213864199,-0.911763130563585));
#38821=DIRECTION('center_axis',(-2.44929359829084E-16,-1.,1.22464679914533E-16));
#38822=DIRECTION('ref_axis',(-0.17719394991793,-7.71267921984697E-17,-0.984175951805612));
#38823=DIRECTION('',(2.67621944414E-16,1.,-1.07048777765E-15));
#38824=DIRECTION('center_axis',(-0.996740111917573,0.0806792990324772,1.47358394346062E-6));
#38825=DIRECTION('ref_axis',(0.080679298682933,0.996740105534059,0.000113066272843588));
#38826=DIRECTION('center_axis',(0.164797595711241,0.072937415919611,0.983626903763192));
#38827=DIRECTION('ref_axis',(-0.00994679585199009,-0.997088453026087,0.0756021037691614));
#38828=DIRECTION('center_axis',(1.,-2.44929359829E-16,3.67394039744E-16));
#38829=DIRECTION('ref_axis',(-3.67394039744E-16,0.,1.));
#38830=DIRECTION('',(0.,0.,-1.));
#38831=DIRECTION('center_axis',(-2.44929359829E-16,-1.,1.22464679915E-16));
#38832=DIRECTION('ref_axis',(-7.42634721754E-16,1.22464679915E-16,1.));
#38833=DIRECTION('center_axis',(-2.44929359829E-16,-1.,1.22464679915E-16));
#38834=DIRECTION('ref_axis',(1.,-2.44929359829E-16,6.54860237547756E-33));
#38835=DIRECTION('',(0.,-1.,0.));
#38836=DIRECTION('center_axis',(-2.44929359829E-16,-1.,1.22464679915E-16));
#38837=DIRECTION('ref_axis',(1.,-2.44929359829E-16,6.83249535077049E-33));
#38838=DIRECTION('',(0.,-1.,0.));
#38839=DIRECTION('center_axis',(-2.18773443555785E-16,-1.,1.58554584738017E-16));
#38840=DIRECTION('ref_axis',(0.586831315816962,0.,0.809709211245947));
#38841=DIRECTION('center_axis',(-0.809709211245947,2.70187668013982E-16,
0.586831315816962));
#38842=DIRECTION('ref_axis',(0.586831315816962,-1.3944828999061E-30,0.809709211245947));
#38843=DIRECTION('center_axis',(-0.828419399070054,1.34310750335009E-16,
-0.560108292426036));
#38844=DIRECTION('ref_axis',(0.560108292426036,6.83578973261393E-31,-0.828419399070054));
#38845=DIRECTION('center_axis',(-6.43747505554034E-17,-1.,-6.27537777746355E-17));
#38846=DIRECTION('ref_axis',(0.698033961608026,0.,-0.716064653814029));
#38847=DIRECTION('center_axis',(0.716064653814028,-8.99007515774035E-17,
0.698033961608027));
#38848=DIRECTION('ref_axis',(0.698033961608027,-7.96736102322353E-31,-0.716064653814028));
#38849=DIRECTION('center_axis',(-2.44929359829E-16,-1.,1.22464679915E-16));
#38850=DIRECTION('ref_axis',(1.,-2.44929359829E-16,2.99951956532444E-32));
#38851=DIRECTION('center_axis',(2.44929359829294E-16,1.,-1.22464679914594E-16));
#38852=DIRECTION('ref_axis',(0.586831315816961,-4.4571439131697E-17,0.809709211245947));
#38853=DIRECTION('',(-4.80096443081E-16,-1.,0.));
#38854=DIRECTION('center_axis',(-2.44929359829E-16,-1.,1.22464679915E-16));
#38855=DIRECTION('ref_axis',(1.,-2.44929359829E-16,2.99951956532444E-32));
#38856=DIRECTION('center_axis',(0.716064653814028,-8.990075157705E-17,0.698033961608027));
#38857=DIRECTION('ref_axis',(-3.28514270034646E-16,-1.,2.08208645226189E-16));
#38858=DIRECTION('center_axis',(0.716064653814028,-8.99007515774035E-17,
0.698033961608027));
#38859=DIRECTION('ref_axis',(0.698033961608027,-7.96736102322353E-31,-0.716064653814028));
#38860=DIRECTION('',(0.716064653814028,0.,0.698033961608027));
#38861=DIRECTION('center_axis',(0.698033961608027,-2.5866163998301E-16,
-0.716064653814028));
#38862=DIRECTION('ref_axis',(-5.0987642944624E-33,-1.,3.6122665544973E-16));
#38863=DIRECTION('',(0.,1.,0.));
#38864=DIRECTION('',(0.716064653814028,0.,0.698033961608027));
#38865=DIRECTION('center_axis',(-6.43747505554034E-17,-1.,-6.27537777746355E-17));
#38866=DIRECTION('ref_axis',(-0.698033961608025,0.,0.71606465381403));
#38867=DIRECTION('center_axis',(-0.698033961608027,2.5866163998301E-16,
0.716064653814028));
#38868=DIRECTION('ref_axis',(0.716064653814028,2.30891390163356E-30,0.698033961608027));
#38869=DIRECTION('center_axis',(2.44929359829E-16,1.,-1.22464679915E-16));
#38870=DIRECTION('ref_axis',(1.,-2.44929359829E-16,2.99951956532444E-32));
#38871=DIRECTION('center_axis',(-2.44929359828773E-16,-1.,1.22464679914767E-16));
#38872=DIRECTION('ref_axis',(-0.698033961608027,2.5866163998301E-16,0.716064653814028));
#38873=DIRECTION('',(4.80096443081E-16,1.,0.));
#38874=DIRECTION('center_axis',(2.44929359829E-16,1.,-1.22464679915E-16));
#38875=DIRECTION('ref_axis',(1.,-2.44929359829E-16,2.99951956532444E-32));
#38876=DIRECTION('center_axis',(-0.698033961608027,2.58661639983637E-16,
0.716064653814028));
#38877=DIRECTION('ref_axis',(-1.80554609273807E-16,-1.,1.85218457689851E-16));
#38878=DIRECTION('center_axis',(-0.698033961608027,2.5866163998301E-16,
0.716064653814028));
#38879=DIRECTION('ref_axis',(0.716064653814028,2.30891390163356E-30,0.698033961608027));
#38880=DIRECTION('',(-0.698033961608027,0.,0.716064653814028));
#38881=DIRECTION('center_axis',(0.716064653814028,-8.99007515774035E-17,
0.698033961608027));
#38882=DIRECTION('ref_axis',(-2.12219958443594E-33,-1.,-1.28791371941708E-16));
#38883=DIRECTION('',(0.,1.,0.));
#38884=DIRECTION('',(-0.698033961608027,4.30707715433016E-16,0.716064653814028));
#38885=DIRECTION('center_axis',(-1.80554609273596E-16,-1.,1.85218457689635E-16));
#38886=DIRECTION('ref_axis',(-0.71606465381403,0.,-0.698033961608025));
#38887=DIRECTION('center_axis',(-0.716064653814028,8.99007515774035E-17,
-0.698033961608027));
#38888=DIRECTION('ref_axis',(0.698033961608027,-2.36964484828339E-31,-0.716064653814028));
#38889=DIRECTION('center_axis',(2.44929359829E-16,1.,-1.22464679915E-16));
#38890=DIRECTION('ref_axis',(1.,-2.44929359829E-16,2.99951956532444E-32));
#38891=DIRECTION('center_axis',(-2.44929359829491E-16,-1.,1.22464679914521E-16));
#38892=DIRECTION('ref_axis',(-0.716064653814027,8.99007515774033E-17,-0.698033961608028));
#38893=DIRECTION('',(4.80096443081E-16,1.,-2.40048221541E-16));
#38894=DIRECTION('center_axis',(2.44929359829E-16,1.,-1.22464679915E-16));
#38895=DIRECTION('ref_axis',(1.,-2.44929359829E-16,2.99951956532444E-32));
#38896=DIRECTION('center_axis',(0.716064653814028,-8.99007515774036E-17,
0.698033961608027));
#38897=DIRECTION('ref_axis',(-0.698033961608027,4.9741364910786E-33,0.716064653814028));
#38898=DIRECTION('center_axis',(-0.716064653814028,8.99007515774035E-17,
-0.698033961608027));
#38899=DIRECTION('ref_axis',(0.698033961608027,-7.96736102322353E-31,-0.716064653814028));
#38900=DIRECTION('',(-0.716064653814028,0.,-0.698033961608027));
#38901=DIRECTION('center_axis',(0.698033961608027,-2.5866163998301E-16,
-0.716064653814028));
#38902=DIRECTION('ref_axis',(-5.0987642944624E-33,-1.,3.6122665544973E-16));
#38903=DIRECTION('',(0.,-1.,0.));
#38904=DIRECTION('',(-0.716064653814028,0.,-0.698033961608027));
#38905=DIRECTION('center_axis',(-1.32057957382078E-16,-1.,1.9781552453987E-16));
#38906=DIRECTION('ref_axis',(0.831699011544245,0.,0.555226759258166));
#38907=DIRECTION('center_axis',(-0.555226759258164,2.37845087940071E-16,
0.831699011544246));
#38908=DIRECTION('ref_axis',(0.831699011544246,1.10558455272238E-30,0.555226759258164));
#38909=DIRECTION('center_axis',(-2.44929359829E-16,-1.,1.22464679915E-16));
#38910=DIRECTION('ref_axis',(1.,-2.44929359829E-16,2.99951956532444E-32));
#38911=DIRECTION('center_axis',(-2.4492935982974E-16,-1.,1.22464679914506E-16));
#38912=DIRECTION('ref_axis',(0.831699011544246,-1.3571183911604E-16,0.555226759258164));
#38913=DIRECTION('',(-4.55476112667E-16,-1.,0.));
#38914=DIRECTION('center_axis',(-2.44929359829E-16,-1.,1.22464679915E-16));
#38915=DIRECTION('ref_axis',(1.,-2.44929359829E-16,2.99951956532444E-32));
#38916=DIRECTION('center_axis',(-9.88589466193077E-17,-1.,1.96101782897063E-16));
#38917=DIRECTION('ref_axis',(0.892950553792926,0.,0.450154760588963));
#38918=DIRECTION('center_axis',(-0.450154760588963,2.19611021084982E-16,
0.892950553792926));
#38919=DIRECTION('ref_axis',(0.892950553792926,5.80220876798355E-31,0.450154760588963));
#38920=DIRECTION('center_axis',(-2.44929359829E-16,-1.,1.22464679915E-16));
#38921=DIRECTION('ref_axis',(1.,-2.44929359829E-16,6.83249535077049E-33));
#38922=DIRECTION('center_axis',(2.44929359829E-16,1.,-1.22464679915E-16));
#38923=DIRECTION('ref_axis',(7.84664226532002E-18,1.22464679915E-16,1.));
#38924=DIRECTION('',(0.,-1.,0.));
#38925=DIRECTION('center_axis',(-2.44929359829E-16,-1.,1.22464679915E-16));
#38926=DIRECTION('ref_axis',(1.,-2.44929359829E-16,-2.34494220138087E-32));
#38927=DIRECTION('center_axis',(-8.70163887007781E-31,-1.,1.22464679915002E-16));
#38928=DIRECTION('ref_axis',(1.,0.,7.105427357601E-15));
#38929=DIRECTION('center_axis',(-3.67394039744E-16,1.22464679915E-16,1.));
#38930=DIRECTION('ref_axis',(1.,4.49927934799277E-32,3.67394039744E-16));
#38931=DIRECTION('center_axis',(-2.44929359829E-16,-1.,1.22464679915E-16));
#38932=DIRECTION('ref_axis',(1.,-2.44929359829E-16,2.99951956532443E-32));
#38933=DIRECTION('center_axis',(-2.44929359829001E-16,-1.,1.22464679915E-16));
#38934=DIRECTION('ref_axis',(1.,-2.44929359829E-16,6.93889390390722E-15));
#38935=DIRECTION('',(-4.80096443081E-16,-1.,2.40048221541E-16));
#38936=DIRECTION('center_axis',(-2.44929359829E-16,-1.,1.22464679915E-16));
#38937=DIRECTION('ref_axis',(1.,-2.44929359829E-16,2.99951956532443E-32));
#38938=DIRECTION('center_axis',(3.67394039744E-16,-1.22464679915E-16,-1.));
#38939=DIRECTION('ref_axis',(1.,-4.87061678881549E-46,3.67394039744E-16));
#38940=DIRECTION('center_axis',(-3.33066907388E-16,1.22464679915E-16,1.));
#38941=DIRECTION('ref_axis',(1.,4.07889322035504E-32,3.33066907388E-16));
#38942=DIRECTION('',(-5.12480847979E-16,0.,1.));
#38943=DIRECTION('center_axis',(-1.,2.44929359829E-16,-4.93371725307E-16));
#38944=DIRECTION('ref_axis',(-4.93371725307E-16,0.,1.));
#38945=DIRECTION('',(0.,-1.,0.));
#38946=DIRECTION('',(-4.78802382588E-16,0.,1.));
#38947=DIRECTION('center_axis',(-4.05685585531587E-19,-1.,-8.04739169685281E-19));
#38948=DIRECTION('ref_axis',(0.892950553792926,0.,-0.450154760588964));
#38949=DIRECTION('center_axis',(0.450154760588963,-9.01213585416925E-19,
0.892950553792926));
#38950=DIRECTION('ref_axis',(0.892950553792926,2.40393060631611E-33,-0.450154760588963));
#38951=DIRECTION('center_axis',(-2.44929359829E-16,-1.,1.22464679915E-16));
#38952=DIRECTION('ref_axis',(1.,-2.44929359829E-16,2.99951956532443E-32));
#38953=DIRECTION('center_axis',(-2.44929359828808E-16,-1.,1.22464679914903E-16));
#38954=DIRECTION('ref_axis',(0.892950553792926,-2.73837866166978E-16,-0.450154760588963));
#38955=DIRECTION('',(0.,-1.,2.27738056333E-16));
#38956=DIRECTION('center_axis',(-2.44929359829E-16,-1.,1.22464679915E-16));
#38957=DIRECTION('ref_axis',(1.,-2.44929359829E-16,2.99951956532443E-32));
#38958=DIRECTION('center_axis',(-3.90625602496874E-16,-1.,2.19728776096112E-16));
#38959=DIRECTION('ref_axis',(0.831699011544246,-4.46882223748491E-16,-0.555226759258164));
#38960=DIRECTION('center_axis',(0.555226759258164,-3.41375814712101E-17,
0.831699011544246));
#38961=DIRECTION('ref_axis',(0.831699011544246,1.57834305747204E-31,-0.555226759258164));
#38962=DIRECTION('center_axis',(-2.44929359829E-16,-1.,1.22464679915E-16));
#38963=DIRECTION('ref_axis',(1.,-2.44929359829E-16,6.83249535077049E-33));
#38964=DIRECTION('center_axis',(2.44929359829E-16,1.,-1.22464679915E-16));
#38965=DIRECTION('ref_axis',(7.84664226532002E-18,1.22464679915E-16,1.));
#38966=DIRECTION('',(0.,-1.,0.));
#38967=DIRECTION('center_axis',(-2.44929359829E-16,-1.,1.22464679915E-16));
#38968=DIRECTION('ref_axis',(1.,-2.44929359829E-16,6.54860237547756E-33));
#38969=DIRECTION('center_axis',(-1.86799616485145E-16,-1.,1.82095954083848E-16));
#38970=DIRECTION('ref_axis',(-0.698033961608026,0.,-0.716064653814029));
#38971=DIRECTION('center_axis',(0.716064653814028,-2.6086976293301E-16,
-0.698033961608027));
#38972=DIRECTION('ref_axis',(0.698033961608027,-2.32071020223926E-30,0.716064653814028));
#38973=DIRECTION('center_axis',(-2.44929359829E-16,-1.,1.22464679915E-16));
#38974=DIRECTION('ref_axis',(1.,-2.44929359829E-16,2.99951956532444E-32));
#38975=DIRECTION('center_axis',(2.44929359829285E-16,1.,-1.2246467991519E-16));
#38976=DIRECTION('ref_axis',(0.831699011544246,-2.7170317382108E-16,-0.555226759258164));
#38977=DIRECTION('',(-4.80096443081E-16,-1.,0.));
#38978=DIRECTION('center_axis',(-2.44929359829E-16,-1.,1.22464679915E-16));
#38979=DIRECTION('ref_axis',(1.,-2.44929359829E-16,2.99951956532444E-32));
#38980=DIRECTION('center_axis',(0.716064653814028,-2.60869762933355E-16,
-0.698033961608027));
#38981=DIRECTION('ref_axis',(-1.8679961648542E-16,-1.,1.82095954084116E-16));
#38982=DIRECTION('center_axis',(0.716064653814028,-2.6086976293301E-16,
-0.698033961608027));
#38983=DIRECTION('ref_axis',(0.698033961608027,-7.02188537105379E-31,0.716064653814028));
#38984=DIRECTION('',(0.716064653814028,0.,-0.698033961608027));
#38985=DIRECTION('center_axis',(-0.698033961608027,8.32763827281032E-17,
-0.716064653814028));
#38986=DIRECTION('ref_axis',(-0.716064653814028,-6.03301243078373E-33,0.698033961608027));
#38987=DIRECTION('',(0.,1.,0.));
#38988=DIRECTION('',(0.716064653814028,-2.6102542122301E-16,-0.698033961608027));
#38989=DIRECTION('center_axis',(-1.86799616485145E-16,-1.,1.82095954083848E-16));
#38990=DIRECTION('ref_axis',(0.698033961608026,0.,0.716064653814029));
#38991=DIRECTION('center_axis',(0.698033961608027,-8.32763827281032E-17,
0.716064653814028));
#38992=DIRECTION('ref_axis',(0.716064653814028,7.37176741734741E-31,-0.698033961608027));
#38993=DIRECTION('center_axis',(2.44929359829E-16,1.,-1.22464679915E-16));
#38994=DIRECTION('ref_axis',(1.,-2.44929359829E-16,2.99951956532444E-32));
#38995=DIRECTION('center_axis',(-2.44929359829229E-16,-1.,1.22464679914765E-16));
#38996=DIRECTION('ref_axis',(0.698033961608028,-8.32763827281037E-17,0.716064653814027));
#38997=DIRECTION('',(4.80096443081E-16,1.,-2.40048221541E-16));
#38998=DIRECTION('center_axis',(2.44929359829E-16,1.,-1.22464679915E-16));
#38999=DIRECTION('ref_axis',(1.,-2.44929359829E-16,2.99951956532444E-32));
#39000=DIRECTION('center_axis',(-0.698033961608027,8.32763827281032E-17,
-0.716064653814028));
#39001=DIRECTION('ref_axis',(0.716064653814028,7.37176741734741E-31,-0.698033961608027));
#39002=DIRECTION('center_axis',(0.698033961608027,-8.32763827281032E-17,
0.716064653814028));
#39003=DIRECTION('ref_axis',(0.716064653814028,7.37176741734741E-31,-0.698033961608027));
#39004=DIRECTION('',(0.698033961608027,0.,0.716064653814028));
#39005=DIRECTION('center_axis',(-0.716064653814028,2.6086976293301E-16,
0.698033961608027));
#39006=DIRECTION('ref_axis',(3.64310347597135E-16,1.,-2.26745038145461E-32));
#39007=DIRECTION('',(0.,1.,0.));
#39008=DIRECTION('',(0.698033961608027,0.,0.716064653814028));
#39009=DIRECTION('center_axis',(-5.81297433438548E-17,-1.,-5.96312741688484E-17));
#39010=DIRECTION('ref_axis',(-0.71606465381403,0.,0.698033961608025));
#39011=DIRECTION('center_axis',(-0.716064653814028,2.6086976293301E-16,
0.698033961608027));
#39012=DIRECTION('ref_axis',(0.698033961608027,-2.32071020223926E-30,0.716064653814028));
#39013=DIRECTION('center_axis',(2.44929359829E-16,1.,-1.22464679915E-16));
#39014=DIRECTION('ref_axis',(1.,-2.44929359829E-16,2.99951956532444E-32));
#39015=DIRECTION('center_axis',(-2.44929359829028E-16,-1.,1.22464679915027E-16));
#39016=DIRECTION('ref_axis',(-0.716064653814028,2.6086976293301E-16,0.698033961608027));
#39017=DIRECTION('',(4.80096443081E-16,1.,0.));
#39018=DIRECTION('center_axis',(2.44929359829E-16,1.,-1.22464679915E-16));
#39019=DIRECTION('ref_axis',(1.,-2.44929359829E-16,2.99951956532444E-32));
#39020=DIRECTION('center_axis',(0.716064653814028,-2.6086976293301E-16,
-0.698033961608027));
#39021=DIRECTION('ref_axis',(0.698033961608027,-1.10143058876371E-32,0.716064653814028));
#39022=DIRECTION('center_axis',(-0.716064653814028,2.6086976293301E-16,
0.698033961608027));
#39023=DIRECTION('ref_axis',(0.698033961608027,-2.32071020223926E-30,0.716064653814028));
#39024=DIRECTION('',(-0.716064653814028,0.,0.698033961608027));
#39025=DIRECTION('center_axis',(-0.698033961608027,8.32763827281032E-17,
-0.716064653814028));
#39026=DIRECTION('ref_axis',(-0.716064653814028,-6.03301243078373E-33,0.698033961608027));
#39027=DIRECTION('',(0.,-1.,0.));
#39028=DIRECTION('',(-0.716064653814028,2.5912401877601E-16,0.698033961608027));
#39029=DIRECTION('center_axis',(-1.02392142274414E-16,-1.,-7.42080178237726E-17));
#39030=DIRECTION('ref_axis',(0.586831315816962,0.,-0.809709211245946));
#39031=DIRECTION('center_axis',(0.809709211245947,-1.26455449502992E-16,
0.586831315816962));
#39032=DIRECTION('ref_axis',(0.586831315816962,-6.48713419669698E-31,-0.809709211245947));
#39033=DIRECTION('center_axis',(-2.44929359829E-16,-1.,1.22464679915E-16));
#39034=DIRECTION('ref_axis',(1.,-2.44929359829E-16,2.99951956532444E-32));
#39035=DIRECTION('center_axis',(-2.4492935982892E-16,-1.,1.2246467991489E-16));
#39036=DIRECTION('ref_axis',(0.586831315816961,-2.42892997889984E-16,-0.809709211245947));
#39037=DIRECTION('',(0.,-1.,0.));
#39038=DIRECTION('center_axis',(-2.44929359829E-16,-1.,1.22464679915E-16));
#39039=DIRECTION('ref_axis',(1.,-2.44929359829E-16,2.99951956532444E-32));
#39040=DIRECTION('center_axis',(2.44929359829E-16,1.,-1.22464679915E-16));
#39041=DIRECTION('ref_axis',(1.14618037649415E-16,-1.22464679915E-16,-1.));
#39042=DIRECTION('center_axis',(-2.44929359829E-16,-1.,1.22464679915E-16));
#39043=DIRECTION('ref_axis',(1.,-2.44929359829E-16,7.76111877854652E-34));
#39044=DIRECTION('center_axis',(-2.44929359829E-16,-1.,1.22464679915E-16));
#39045=DIRECTION('ref_axis',(1.,-2.44929359829E-16,6.83249535077049E-33));
#39046=DIRECTION('',(0.,-1.,0.));
#39047=DIRECTION('center_axis',(-2.18773443555785E-16,-1.,1.58554584738017E-16));
#39048=DIRECTION('ref_axis',(-0.586831315816962,0.,-0.809709211245947));
#39049=DIRECTION('center_axis',(0.809709211245947,-2.70187668013982E-16,
-0.586831315816962));
#39050=DIRECTION('ref_axis',(0.586831315816962,-1.3944828999061E-30,0.809709211245947));
#39051=DIRECTION('center_axis',(-6.43747505554034E-17,-1.,-6.27537777746355E-17));
#39052=DIRECTION('ref_axis',(-0.698033961608026,0.,0.716064653814029));
#39053=DIRECTION('center_axis',(-0.716064653814028,8.99007515774035E-17,
-0.698033961608027));
#39054=DIRECTION('ref_axis',(0.698033961608027,-7.96736102322353E-31,-0.716064653814028));
#39055=DIRECTION('center_axis',(-2.44929359829E-16,-1.,1.22464679915E-16));
#39056=DIRECTION('ref_axis',(1.,-2.44929359829E-16,2.99951956532444E-32));
#39057=DIRECTION('center_axis',(2.44929359829294E-16,1.,-1.22464679914594E-16));
#39058=DIRECTION('ref_axis',(-0.586831315816961,4.4571439131697E-17,-0.809709211245947));
#39059=DIRECTION('',(-4.80096443081E-16,-1.,0.));
#39060=DIRECTION('center_axis',(-2.44929359829E-16,-1.,1.22464679915E-16));
#39061=DIRECTION('ref_axis',(1.,-2.44929359829E-16,2.99951956532444E-32));
#39062=DIRECTION('center_axis',(-0.716064653814028,8.99007515776184E-17,
-0.698033961608027));
#39063=DIRECTION('ref_axis',(-6.43747505560482E-17,-1.,-6.27537777752641E-17));
#39064=DIRECTION('center_axis',(-0.716064653814028,8.99007515774035E-17,
-0.698033961608027));
#39065=DIRECTION('ref_axis',(0.698033961608027,-7.96736102322353E-31,-0.716064653814028));
#39066=DIRECTION('',(-0.716064653814028,0.,-0.698033961608027));
#39067=DIRECTION('center_axis',(-0.698033961608027,2.5866163998301E-16,
0.716064653814028));
#39068=DIRECTION('ref_axis',(3.70557385756911E-16,1.,-1.7912467654698E-32));
#39069=DIRECTION('',(0.,1.,0.));
#39070=DIRECTION('',(-0.716064653814028,0.,-0.698033961608027));
#39071=DIRECTION('center_axis',(-6.43747505554034E-17,-1.,-6.27537777746355E-17));
#39072=DIRECTION('ref_axis',(0.698033961608025,0.,-0.71606465381403));
#39073=DIRECTION('center_axis',(0.698033961608027,-2.5866163998301E-16,
-0.716064653814028));
#39074=DIRECTION('ref_axis',(0.716064653814028,2.30891390163356E-30,0.698033961608027));
#39075=DIRECTION('center_axis',(2.44929359829E-16,1.,-1.22464679915E-16));
#39076=DIRECTION('ref_axis',(1.,-2.44929359829E-16,2.99951956532444E-32));
#39077=DIRECTION('center_axis',(-2.44929359828773E-16,-1.,1.22464679914767E-16));
#39078=DIRECTION('ref_axis',(0.698033961608027,-2.5866163998301E-16,-0.716064653814028));
#39079=DIRECTION('',(4.80096443081E-16,1.,0.));
#39080=DIRECTION('center_axis',(2.44929359829E-16,1.,-1.22464679915E-16));
#39081=DIRECTION('ref_axis',(1.,-2.44929359829E-16,2.99951956532444E-32));
#39082=DIRECTION('center_axis',(0.698033961608027,-2.58661639983667E-16,
-0.716064653814028));
#39083=DIRECTION('ref_axis',(-1.80554609273828E-16,-1.,1.85218457689873E-16));
#39084=DIRECTION('center_axis',(0.698033961608027,-2.5866163998301E-16,
-0.716064653814028));
#39085=DIRECTION('ref_axis',(0.716064653814028,2.30891390163356E-30,0.698033961608027));
#39086=DIRECTION('',(0.698033961608027,0.,-0.716064653814028));
#39087=DIRECTION('center_axis',(-0.716064653814028,8.99007515774035E-17,
-0.698033961608027));
#39088=DIRECTION('ref_axis',(-0.698033961608027,-3.69855194764065E-33,0.716064653814028));
#39089=DIRECTION('',(0.,1.,0.));
#39090=DIRECTION('',(0.698033961608027,-4.30707715433016E-16,-0.716064653814028));
#39091=DIRECTION('center_axis',(-1.80554609273596E-16,-1.,1.85218457689635E-16));
#39092=DIRECTION('ref_axis',(0.71606465381403,0.,0.698033961608025));
#39093=DIRECTION('center_axis',(0.716064653814028,-8.99007515774035E-17,
0.698033961608027));
#39094=DIRECTION('ref_axis',(0.698033961608027,-2.36964484828339E-31,-0.716064653814028));
#39095=DIRECTION('center_axis',(2.44929359829E-16,1.,-1.22464679915E-16));
#39096=DIRECTION('ref_axis',(1.,-2.44929359829E-16,2.99951956532444E-32));
#39097=DIRECTION('center_axis',(-2.44929359829491E-16,-1.,1.22464679914521E-16));
#39098=DIRECTION('ref_axis',(0.716064653814027,-8.99007515774033E-17,0.698033961608028));
#39099=DIRECTION('',(4.80096443081E-16,1.,-2.40048221541E-16));
#39100=DIRECTION('center_axis',(2.44929359829E-16,1.,-1.22464679915E-16));
#39101=DIRECTION('ref_axis',(1.,-2.44929359829E-16,2.99951956532444E-32));
#39102=DIRECTION('center_axis',(-0.716064653814028,8.99007515774036E-17,
-0.698033961608027));
#39103=DIRECTION('ref_axis',(0.698033961608027,-4.9741364910786E-33,-0.716064653814028));
#39104=DIRECTION('center_axis',(0.716064653814028,-8.99007515774035E-17,
0.698033961608027));
#39105=DIRECTION('ref_axis',(0.698033961608027,-7.96736102322353E-31,-0.716064653814028));
#39106=DIRECTION('',(0.716064653814028,0.,0.698033961608027));
#39107=DIRECTION('center_axis',(-0.698033961608027,2.5866163998301E-16,
0.716064653814028));
#39108=DIRECTION('ref_axis',(3.70557385756911E-16,1.,-1.7912467654698E-32));
#39109=DIRECTION('',(0.,-1.,0.));
#39110=DIRECTION('',(0.716064653814028,0.,0.698033961608027));
#39111=DIRECTION('center_axis',(-1.32057957382078E-16,-1.,1.9781552453987E-16));
#39112=DIRECTION('ref_axis',(-0.831699011544245,0.,-0.555226759258166));
#39113=DIRECTION('center_axis',(0.555226759258164,-2.37845087940071E-16,
-0.831699011544246));
#39114=DIRECTION('ref_axis',(0.831699011544246,1.10558455272238E-30,0.555226759258164));
#39115=DIRECTION('center_axis',(-2.44929359829E-16,-1.,1.22464679915E-16));
#39116=DIRECTION('ref_axis',(1.,-2.44929359829E-16,2.99951956532444E-32));
#39117=DIRECTION('center_axis',(-2.4492935982974E-16,-1.,1.22464679914506E-16));
#39118=DIRECTION('ref_axis',(-0.831699011544246,1.3571183911604E-16,-0.555226759258164));
#39119=DIRECTION('',(0.,-1.,0.));
#39120=DIRECTION('center_axis',(-2.44929359829E-16,-1.,1.22464679915E-16));
#39121=DIRECTION('ref_axis',(1.,-2.44929359829E-16,2.99951956532444E-32));
#39122=DIRECTION('center_axis',(-9.88589466193077E-17,-1.,1.96101782897063E-16));
#39123=DIRECTION('ref_axis',(-0.892950553792926,0.,-0.450154760588963));
#39124=DIRECTION('center_axis',(0.450154760588963,-2.19611021084982E-16,
-0.892950553792926));
#39125=DIRECTION('ref_axis',(0.892950553792926,5.80220876798355E-31,0.450154760588963));
#39126=DIRECTION('center_axis',(-2.44929359829E-16,-1.,1.22464679915E-16));
#39127=DIRECTION('ref_axis',(1.,-2.44929359829E-16,6.83249535077049E-33));
#39128=DIRECTION('center_axis',(-2.44929359829E-16,-1.,1.22464679915E-16));
#39129=DIRECTION('ref_axis',(-7.42634721754E-16,1.22464679915E-16,1.));
#39130=DIRECTION('',(0.,-1.,0.));
#39131=DIRECTION('center_axis',(-2.44929359829E-16,-1.,1.22464679915E-16));
#39132=DIRECTION('ref_axis',(1.,-2.44929359829E-16,6.54860237547756E-33));
#39133=DIRECTION('center_axis',(-1.74032777401559E-30,-1.,1.22464679915003E-16));
#39134=DIRECTION('ref_axis',(-1.,0.,-1.4210854715202E-14));
#39135=DIRECTION('center_axis',(3.67394039744E-16,-1.22464679915E-16,-1.));
#39136=DIRECTION('ref_axis',(1.,4.49927934799277E-32,3.67394039744E-16));
#39137=DIRECTION('center_axis',(-2.44929359829E-16,-1.,1.22464679915E-16));
#39138=DIRECTION('ref_axis',(1.,-2.44929359829E-16,2.99951956532443E-32));
#39139=DIRECTION('center_axis',(2.44929359829246E-16,1.,-1.22464679914876E-16));
#39140=DIRECTION('ref_axis',(-0.892950553792926,1.63581748831987E-16,-0.450154760588963));
#39141=DIRECTION('',(-4.80096443081E-16,-1.,2.40048221541E-16));
#39142=DIRECTION('center_axis',(-2.44929359829E-16,-1.,1.22464679915E-16));
#39143=DIRECTION('ref_axis',(1.,-2.44929359829E-16,2.99951956532443E-32));
#39144=DIRECTION('center_axis',(3.67394039744E-16,-1.22464679915E-16,-1.));
#39145=DIRECTION('ref_axis',(-1.82825659017378E-45,-1.,1.22464679915E-16));
#39146=DIRECTION('center_axis',(2.05391259556E-15,-1.22464679915E-16,-1.));
#39147=DIRECTION('ref_axis',(1.,2.51531748588642E-31,2.05391259556E-15));
#39148=DIRECTION('',(2.5624042399E-16,0.,-1.));
#39149=DIRECTION('center_axis',(-1.,2.44929359829E-16,-2.41416354181E-16));
#39150=DIRECTION('ref_axis',(-2.41416354181E-16,0.,1.));
#39151=DIRECTION('',(0.,-1.,0.));
#39152=DIRECTION('',(3.19201588392E-16,0.,-1.));
#39153=DIRECTION('center_axis',(-4.05685585531587E-19,-1.,-8.04739169685281E-19));
#39154=DIRECTION('ref_axis',(-0.892950553792926,0.,0.450154760588964));
#39155=DIRECTION('center_axis',(-0.450154760588963,9.01213585422925E-19,
-0.892950553792926));
#39156=DIRECTION('ref_axis',(0.892950553792926,2.37605947729967E-33,-0.450154760588963));
#39157=DIRECTION('center_axis',(-2.44929359829E-16,-1.,1.22464679915E-16));
#39158=DIRECTION('ref_axis',(1.,-2.44929359829E-16,2.99951956532443E-32));
#39159=DIRECTION('center_axis',(2.44929359829E-16,1.,-1.22464679915E-16));
#39160=DIRECTION('ref_axis',(-1.,2.44929359829E-16,-2.99951956532443E-32));
#39161=DIRECTION('',(0.,-1.,2.27738056333E-16));
#39162=DIRECTION('center_axis',(-2.44929359829E-16,-1.,1.22464679915E-16));
#39163=DIRECTION('ref_axis',(1.,-2.44929359829E-16,2.99951956532443E-32));
#39164=DIRECTION('center_axis',(-3.92903534935981E-16,-1.,2.14399869159323E-16));
#39165=DIRECTION('ref_axis',(-0.849410790431843,4.46882223748491E-16,0.527732232384902));
#39166=DIRECTION('center_axis',(-0.527732232384902,2.52342972731953E-17,
-0.849410790431843));
#39167=DIRECTION('ref_axis',(0.849410790431843,-6.27761689185242E-32,-0.527732232384902));
#39168=DIRECTION('center_axis',(-2.44929359829E-16,-1.,1.22464679915E-16));
#39169=DIRECTION('ref_axis',(1.,-2.44929359829E-16,6.83249535077049E-33));
#39170=DIRECTION('center_axis',(-2.44929359829E-16,-1.,1.22464679915E-16));
#39171=DIRECTION('ref_axis',(-7.42634721754E-16,1.22464679915E-16,1.));
#39172=DIRECTION('',(0.,-1.,0.));
#39173=DIRECTION('center_axis',(-2.44929359829E-16,-1.,1.22464679915E-16));
#39174=DIRECTION('ref_axis',(1.,-2.44929359829E-16,-2.34494220138087E-32));
#39175=DIRECTION('center_axis',(-1.86799616485145E-16,-1.,1.82095954083848E-16));
#39176=DIRECTION('ref_axis',(0.698033961608023,0.,0.716064653814032));
#39177=DIRECTION('center_axis',(-0.716064653814028,2.6086976293301E-16,
0.698033961608027));
#39178=DIRECTION('ref_axis',(0.698033961608027,-2.32071020223926E-30,0.716064653814028));
#39179=DIRECTION('center_axis',(-2.44929359829E-16,-1.,1.22464679915E-16));
#39180=DIRECTION('ref_axis',(1.,-2.44929359829E-16,2.99951956532444E-32));
#39181=DIRECTION('center_axis',(2.4492935982882E-16,1.,-1.22464679914888E-16));
#39182=DIRECTION('ref_axis',(-0.849410790431843,2.7267420005195E-16,0.527732232384902));
#39183=DIRECTION('',(-4.55476112667E-16,-1.,0.));
#39184=DIRECTION('center_axis',(-2.44929359829E-16,-1.,1.22464679915E-16));
#39185=DIRECTION('ref_axis',(1.,-2.44929359829E-16,2.99951956532444E-32));
#39186=DIRECTION('center_axis',(-0.716064653814028,2.60869762932787E-16,
0.698033961608027));
#39187=DIRECTION('ref_axis',(-1.86799616485013E-16,-1.,1.8209595408372E-16));
#39188=DIRECTION('center_axis',(-0.716064653814028,2.6086976293301E-16,
0.698033961608027));
#39189=DIRECTION('ref_axis',(0.698033961608027,-7.02188537105379E-31,0.716064653814028));
#39190=DIRECTION('',(-0.716064653814028,0.,0.698033961608027));
#39191=DIRECTION('center_axis',(0.698033961608027,-8.32763827281032E-17,
0.716064653814028));
#39192=DIRECTION('ref_axis',(-1.19301333901095E-16,-1.,6.93490090905032E-33));
#39193=DIRECTION('',(0.,1.,0.));
#39194=DIRECTION('',(-0.716064653814028,2.6591127623201E-16,0.698033961608027));
#39195=DIRECTION('center_axis',(-1.86799616485145E-16,-1.,1.82095954083848E-16));
#39196=DIRECTION('ref_axis',(-0.698033961608026,0.,-0.716064653814029));
#39197=DIRECTION('center_axis',(-0.698033961608027,8.32763827281032E-17,
-0.716064653814028));
#39198=DIRECTION('ref_axis',(0.716064653814028,7.37176741734741E-31,-0.698033961608027));
#39199=DIRECTION('center_axis',(2.44929359829E-16,1.,-1.22464679915E-16));
#39200=DIRECTION('ref_axis',(1.,-2.44929359829E-16,2.99951956532444E-32));
#39201=DIRECTION('center_axis',(-2.44929359829229E-16,-1.,1.22464679914765E-16));
#39202=DIRECTION('ref_axis',(-0.698033961608028,8.32763827281037E-17,-0.716064653814027));
#39203=DIRECTION('',(4.80096443081E-16,1.,-2.40048221541E-16));
#39204=DIRECTION('center_axis',(2.44929359829E-16,1.,-1.22464679915E-16));
#39205=DIRECTION('ref_axis',(1.,-2.44929359829E-16,2.99951956532444E-32));
#39206=DIRECTION('center_axis',(0.698033961608027,-8.32763827281032E-17,
0.716064653814028));
#39207=DIRECTION('ref_axis',(-0.716064653814028,-7.37176741734741E-31,0.698033961608027));
#39208=DIRECTION('center_axis',(-0.698033961608027,8.32763827281032E-17,
-0.716064653814028));
#39209=DIRECTION('ref_axis',(0.716064653814028,2.22654728542614E-31,-0.698033961608027));
#39210=DIRECTION('',(-0.698033961608027,0.,-0.716064653814028));
#39211=DIRECTION('center_axis',(0.716064653814028,-2.6086976293301E-16,
-0.698033961608027));
#39212=DIRECTION('ref_axis',(-1.38053841875249E-32,-1.,3.73720731770783E-16));
#39213=DIRECTION('',(0.,1.,0.));
#39214=DIRECTION('',(-0.698033961608027,0.,-0.716064653814028));
#39215=DIRECTION('center_axis',(-1.11265631080723E-16,-1.,-7.52285650242949E-17));
#39216=DIRECTION('ref_axis',(-0.560108292426038,0.,0.828419399070053));
#39217=DIRECTION('center_axis',(-2.44929359829E-16,-1.,1.22464679915E-16));
#39218=DIRECTION('ref_axis',(1.,-2.44929359829E-16,2.99951956532444E-32));
#39219=DIRECTION('center_axis',(0.716064653814028,-2.6086976293301E-16,
-0.698033961608027));
#39220=DIRECTION('ref_axis',(0.698033961608027,-2.32071020223926E-30,0.716064653814028));
#39221=DIRECTION('center_axis',(-2.44929359828833E-16,-1.,1.22464679914753E-16));
#39222=DIRECTION('ref_axis',(-0.560108292426038,2.38639082041016E-16,0.828419399070053));
#39223=DIRECTION('center_axis',(-2.44929359829E-16,-1.,1.22464679915E-16));
#39224=DIRECTION('ref_axis',(1.,-2.44929359829E-16,2.99951956532444E-32));
#39225=DIRECTION('',(-4.55476112667E-16,-1.,0.));
#39226=DIRECTION('center_axis',(-5.81297433438548E-17,-1.,-5.96312741688484E-17));
#39227=DIRECTION('ref_axis',(0.716064653814029,0.,-0.698033961608026));
#39228=DIRECTION('center_axis',(0.716064653814028,-2.6086976293301E-16,
-0.698033961608027));
#39229=DIRECTION('ref_axis',(0.698033961608027,-2.32071020223926E-30,0.716064653814028));
#39230=DIRECTION('center_axis',(2.44929359829E-16,1.,-1.22464679915E-16));
#39231=DIRECTION('ref_axis',(1.,-2.44929359829E-16,2.99951956532444E-32));
#39232=DIRECTION('center_axis',(-2.44929359829028E-16,-1.,1.22464679915027E-16));
#39233=DIRECTION('ref_axis',(0.716064653814026,-2.6086976293301E-16,-0.69803396160803));
#39234=DIRECTION('',(2.27738056333E-16,1.,0.));
#39235=DIRECTION('center_axis',(2.44929359829E-16,1.,-1.22464679915E-16));
#39236=DIRECTION('ref_axis',(1.,-2.44929359829E-16,2.99951956532444E-32));
#39237=DIRECTION('center_axis',(-0.716064653814028,2.6086976293301E-16,
0.698033961608027));
#39238=DIRECTION('ref_axis',(-0.698033961608027,-1.0524566385888E-31,-0.716064653814028));
#39239=DIRECTION('',(0.716064653814028,0.,-0.698033961608027));
#39240=DIRECTION('center_axis',(0.698033961608027,-8.32763827281032E-17,
0.716064653814028));
#39241=DIRECTION('ref_axis',(-1.19301333901095E-16,-1.,6.93490090905032E-33));
#39242=DIRECTION('',(0.716064653814028,-2.6393829599301E-16,-0.698033961608027));
#39243=DIRECTION('center_axis',(-1.,2.44929359829E-16,-2.41416354181E-16));
#39244=DIRECTION('ref_axis',(-2.41416354181E-16,0.,1.));
#39245=DIRECTION('',(0.,-1.,0.));
#39246=DIRECTION('',(-3.70074341542E-16,0.,1.));
#39247=DIRECTION('',(0.,-1.,0.));
#39248=DIRECTION('',(4.15092802552E-16,0.,-1.));
#39249=DIRECTION('',(0.323037326387015,0.920901128992761,-0.21814673130851));
#39250=DIRECTION('',(0.310424970358247,0.909870545905898,-0.27526701122907));
#39251=DIRECTION('center_axis',(-0.943627470111708,0.331009361877541,0.));
#39252=DIRECTION('ref_axis',(0.,0.,1.));
#39253=DIRECTION('',(0.330975706838633,0.943531527766579,0.0142596491237413));
#39254=DIRECTION('',(-1.64651774315771E-16,0.,-1.));
#39255=DIRECTION('center_axis',(-0.943627482809182,0.331009325680119,1.49146681070121E-9));
#39256=DIRECTION('ref_axis',(0.331009318664928,0.943627462811498,-0.000205875969548059));
#39257=DIRECTION('',(8.57762605026367E-7,2.44526964337894E-6,-0.999999999996642));
#39258=DIRECTION('',(0.294062932800905,0.911816425322849,-0.286562031790662));
#39259=DIRECTION('center_axis',(0.160589675912942,0.276008879795742,0.947644476723247));
#39260=DIRECTION('ref_axis',(-0.0609933906817373,0.961045570864355,-0.269575994879275));
#39261=DIRECTION('',(-0.288992183012555,0.946290745989702,0.144973591429235));
#39262=DIRECTION('',(0.117824078681733,0.966071698379208,0.229832460878599));
#39263=DIRECTION('center_axis',(-1.48089814433846E-9,1.,-1.36711158136743E-9));
#39264=DIRECTION('ref_axis',(-0.738412059057248,-2.01542449026607E-9,-0.674349783894705));
#39265=DIRECTION('',(0.128571714532246,0.968939478859869,0.211247723133303));
#39266=DIRECTION('',(-0.255328810234173,0.774608545951679,0.578609366674121));
#39267=DIRECTION('',(-0.181492548576796,0.738445189679448,0.649429870463611));
#39268=DIRECTION('',(-0.225419688153596,0.803501199046223,0.550973490581913));
#39269=DIRECTION('center_axis',(-4.57218787640431E-10,1.,8.71360109757879E-11));
#39270=DIRECTION('ref_axis',(-0.980286226483734,-4.65421893024152E-10,0.197582676786912));
#39271=DIRECTION('center_axis',(-0.698033961608027,8.32763827281032E-17,
-0.716064653814028));
#39272=DIRECTION('ref_axis',(-0.716064653814028,-6.03301243078373E-33,0.698033961608027));
#39273=DIRECTION('',(0.,-1.,0.));
#39274=DIRECTION('',(0.716064653824126,0.,-0.698033961597667));
#39275=DIRECTION('',(0.716064653814028,0.,-0.698033961608027));
#39276=DIRECTION('center_axis',(-0.698033961608027,2.5866163998301E-16,
0.716064653814028));
#39277=DIRECTION('ref_axis',(3.70557385756911E-16,1.,-1.7912467654698E-32));
#39278=DIRECTION('',(-0.716064653814028,0.,-0.698033961608027));
#39279=DIRECTION('',(0.716064653824126,0.,0.698033961597667));
#39280=DIRECTION('',(0.,-1.,0.));
#39281=DIRECTION('center_axis',(0.892620224620875,-0.100404069962798,0.439486242483976));
#39282=DIRECTION('ref_axis',(0.450785404329455,0.208856364443758,-0.867854560554282));
#39283=DIRECTION('center_axis',(0.436083773086294,0.0976415951931109,0.894593238147353));
#39284=DIRECTION('ref_axis',(0.867935375388418,0.216985732657287,-0.446772174572843));
#39285=DIRECTION('center_axis',(0.00186553655657051,-0.00532586126953934,
0.999984077360782));
#39286=DIRECTION('ref_axis',(0.943629829775382,0.331002634962083,2.49821012154569E-6));
#39287=DIRECTION('center_axis',(0.880062092697831,0.092955957006382,0.465671453981606));
#39288=DIRECTION('ref_axis',(0.441468068374835,0.201070817369295,-0.874457815453573));
#39289=DIRECTION('center_axis',(-2.14201187043523E-15,6.10635672184588E-15,
-1.));
#39290=DIRECTION('ref_axis',(0.943627470093642,0.331009361929045,0.));
#39291=DIRECTION('center_axis',(1.54815906928092E-5,2.538769952355E-6,0.999999999876938));
#39292=DIRECTION('ref_axis',(0.943627561740588,0.331009100305164,-1.54492116365672E-5));
#39293=DIRECTION('',(-8.57762605026367E-7,2.44526964337894E-6,-0.999999999996642));
#39294=DIRECTION('center_axis',(-0.983486256238949,0.0374328207462225,-0.177069386738866));
#39295=DIRECTION('ref_axis',(-0.163009880779526,0.24184812435891,0.956523530035891));
#39296=DIRECTION('center_axis',(0.160588996966396,-0.276000094097635,-0.947647150637527));
#39297=DIRECTION('ref_axis',(0.061024966583606,0.961047601642055,-0.269561608600934));
#39298=DIRECTION('center_axis',(-0.984719314308431,-0.119059960726394,-0.127092870688182));
#39299=DIRECTION('ref_axis',(-0.152586230961459,0.238117387003548,0.959175454297898));
#39300=DIRECTION('center_axis',(-0.0289008325901315,0.0823889103331479,
0.996181112714808));
#39301=DIRECTION('ref_axis',(0.9436275874899,0.331009027260539,1.50441563718168E-7));
#39302=DIRECTION('center_axis',(-0.943627482815775,-0.331009325661324,-1.49233941105659E-9));
#39303=DIRECTION('ref_axis',(0.331008843413436,-0.943626108051448,0.00170698148083177));
#39304=DIRECTION('center_axis',(-0.430110758359808,0.046153110977895,-0.901595599972744));
#39305=DIRECTION('ref_axis',(-0.879739108301929,0.202744349618919,0.430062588493499));
#39306=DIRECTION('center_axis',(-0.980966495583046,-0.0283022044444621,
-0.19210340904602));
#39307=DIRECTION('ref_axis',(-0.19328796736646,0.236890927961216,0.952114725188628));
#39308=DIRECTION('center_axis',(-0.388851273388422,-0.0301047308393102,
-0.920808553590428));
#39309=DIRECTION('ref_axis',(-0.902832709485492,0.211566053131498,0.37434329678177));
#39310=DIRECTION('center_axis',(0.154792429944213,0.0260186560475965,-0.987604340396215));
#39311=DIRECTION('ref_axis',(-0.95105813490232,0.274540052803893,-0.141831531905127));
#39312=DIRECTION('center_axis',(0.158571788614755,0.0251030524526189,-0.987028279540702));
#39313=DIRECTION('ref_axis',(-0.949647192915505,0.277483911944001,-0.145509063635074));
#39314=DIRECTION('center_axis',(0.519128585308313,0.0837939298473311,-0.85057867903947));
#39315=DIRECTION('ref_axis',(-0.763413574425517,0.492955180837497,-0.417366630276459));
#39316=DIRECTION('center_axis',(0.53027158586854,0.0827827349147078,-0.843776667146292));
#39317=DIRECTION('ref_axis',(-0.753475381714833,0.502288029862624,-0.424242364935906));
#39318=DIRECTION('center_axis',(0.648542405801268,0.0976477666270568,-0.754889171700224));
#39319=DIRECTION('ref_axis',(-0.653871091131623,0.579173686319672,-0.4868371773573));
#39320=DIRECTION('center_axis',(0.494563463497324,-0.191710317879514,0.847734707672198));
#39321=DIRECTION('ref_axis',(0.865846793003873,0.193521564619003,-0.461366161603039));
#39322=DIRECTION('center_axis',(0.464395725684733,-0.198543507192818,0.863085792790801));
#39323=DIRECTION('ref_axis',(0.883803239974284,0.166419749377341,-0.437259991341698));
#39324=DIRECTION('',(0.113178938997705,0.763679548992658,0.635597415206925));
#39325=DIRECTION('',(0.181492548576796,0.738445189679448,0.649429870463611));
#39326=DIRECTION('center_axis',(-0.396005905940162,-0.201097924900932,0.8959570006764));
#39327=DIRECTION('ref_axis',(0.891702233585015,0.148696398124815,0.427500301525276));
#39328=DIRECTION('',(-0.117824078681021,0.96607169838126,0.229832460870341));
#39329=DIRECTION('center_axis',(0.922778105750095,-0.103279309791534,0.371233015392289));
#39330=DIRECTION('ref_axis',(0.385281285161793,0.262890595038936,-0.884560267219906));
#39331=DIRECTION('center_axis',(-0.878226997877743,-0.135323395232607,0.458699159473141));
#39332=DIRECTION('ref_axis',(0.477362666720091,-0.189841514555233,0.857954010290329));
#39333=DIRECTION('center_axis',(0.456738059260596,-0.0359334235885344,0.888875207378444));
#39334=DIRECTION('ref_axis',(0.872740846734216,0.211709714743671,-0.439889089572357));
#39335=DIRECTION('center_axis',(0.920065996825176,-0.0139599992294347,0.391514597311019));
#39336=DIRECTION('ref_axis',(0.381633312533999,0.257729359286959,-0.887655108770214));
#39337=DIRECTION('center_axis',(0.892620455906449,0.100404015839207,-0.439485785095176));
#39338=DIRECTION('ref_axis',(-0.450784946851557,0.208856415901993,-0.867854785795764));
#39339=DIRECTION('center_axis',(0.880062092716156,-0.092955957010435,-0.465671453946163));
#39340=DIRECTION('ref_axis',(-0.441468068339719,0.201070817365602,-0.874457815472151));
#39341=DIRECTION('center_axis',(0.00186854672551137,0.0053252415770575,
-0.999984075040838));
#39342=DIRECTION('ref_axis',(-0.943627592819709,0.33100901206617,-5.09303340548844E-7));
#39343=DIRECTION('center_axis',(0.436083773086294,-0.0976415951931109,-0.894593238147353));
#39344=DIRECTION('ref_axis',(-0.867935375388418,0.216985732657287,-0.446772174572843));
#39345=DIRECTION('center_axis',(0.922778105089071,0.103279310020637,-0.371233016971665));
#39346=DIRECTION('ref_axis',(-0.38528128674108,0.262890594935205,-0.884560266562856));
#39347=DIRECTION('center_axis',(-0.396017498125805,0.201038848453509,-0.895965134695913));
#39348=DIRECTION('ref_axis',(0.888623240590356,-0.161920158177116,-0.429104414634237));
#39349=DIRECTION('center_axis',(0.919974181323324,0.0139905959715904,-0.391729203561387));
#39350=DIRECTION('ref_axis',(-0.381848078164205,0.257725957261476,-0.88756373075738));
#39351=DIRECTION('center_axis',(0.456738059260626,0.0359334235885297,-0.888875207378428));
#39352=DIRECTION('ref_axis',(-0.872740846734205,0.211709714743646,-0.43988908957239));
#39353=DIRECTION('center_axis',(-0.878226997877743,0.135323395232607,-0.458699159473141));
#39354=DIRECTION('ref_axis',(0.477362666720091,0.189841514555233,-0.857954010290329));
#39355=DIRECTION('',(-0.113178938997705,0.763679548992658,0.635597415206925));
#39356=DIRECTION('center_axis',(0.464395555049772,0.198543523260408,-0.8630858809072));
#39357=DIRECTION('ref_axis',(-0.883803329144551,0.16641971123809,-0.437259825623666));
#39358=DIRECTION('center_axis',(0.495307295122513,0.191627071871079,-0.847319153993663));
#39359=DIRECTION('ref_axis',(-0.865425172209434,0.193684803027571,-0.462088160833452));
#39360=DIRECTION('center_axis',(0.648543686882833,-0.0976472412892305,0.754888139046458));
#39361=DIRECTION('ref_axis',(0.65387002449902,0.579173846918327,-0.486838418890166));
#39362=DIRECTION('center_axis',(0.530204044384788,-0.0828039354466806,0.843817029688638));
#39363=DIRECTION('ref_axis',(0.753516762104764,0.502282247298617,-0.424175710379322));
#39364=DIRECTION('center_axis',(0.519038701925307,-0.0838213303629659,0.850630830901323));
#39365=DIRECTION('ref_axis',(0.763467531439435,0.492946409813472,-0.41727828303158));
#39366=DIRECTION('center_axis',(0.158462664464082,-0.0251186847944935,0.987045407083757));
#39367=DIRECTION('ref_axis',(0.949664686103619,0.277481196947328,-0.1454000320096));
#39368=DIRECTION('center_axis',(0.154792396107517,-0.0260186608384927,0.987604345573401));
#39369=DIRECTION('ref_axis',(0.951058139598754,0.274540054077438,-0.141831497947794));
#39370=DIRECTION('center_axis',(-0.388296589591557,0.0301690890474203,0.92104049019444));
#39371=DIRECTION('ref_axis',(0.903066320863432,0.211547985251654,0.373789606674866));
#39372=DIRECTION('center_axis',(-0.430257355733273,-0.0461697877906974,
0.901524796404832));
#39373=DIRECTION('ref_axis',(0.879669075246814,0.202736833246679,0.430209361241156));
#39374=DIRECTION('center_axis',(-0.980966495583046,0.0283022044444621,0.19210340904602));
#39375=DIRECTION('ref_axis',(0.19328796736646,0.236890927961216,0.952114725188628));
#39376=DIRECTION('center_axis',(-0.983486190287356,-0.0374327738616832,
0.177069762961054));
#39377=DIRECTION('ref_axis',(0.16301025642708,0.24184813865655,0.95652346240327));
#39378=DIRECTION('center_axis',(1.52856649600948E-5,-2.50540282491327E-6,
-0.999999999880036));
#39379=DIRECTION('ref_axis',(-0.943627561743776,0.331009100305162,-1.52532858923899E-5));
#39380=DIRECTION('center_axis',(-0.0289009651132723,-0.0823888877589006,
-0.996181110737085));
#39381=DIRECTION('ref_axis',(-0.943627583659813,0.331009038179116,2.82460236826103E-7));
#39382=DIRECTION('center_axis',(-0.984716782786941,0.119056590783676,0.127115639827304));
#39383=DIRECTION('ref_axis',(0.152607474441606,0.238116529713297,0.959172287455101));
#39384=DIRECTION('center_axis',(-2.14201187043523E-15,-6.10635672184588E-15,
1.));
#39385=DIRECTION('ref_axis',(-0.943627470093642,0.331009361929045,0.));
#39386=DIRECTION('center_axis',(-2.18773443555785E-16,-1.,1.58554584738017E-16));
#39387=DIRECTION('ref_axis',(0.586831315816962,0.,0.809709211245947));
#39388=DIRECTION('center_axis',(-0.809709211245947,2.70187668013982E-16,
0.586831315816962));
#39389=DIRECTION('ref_axis',(0.586831315816962,-1.3944828999061E-30,0.809709211245947));
#39390=DIRECTION('center_axis',(-2.44929359829E-16,-1.,1.22464679915E-16));
#39391=DIRECTION('ref_axis',(1.,-2.44929359829E-16,5.91180967883826E-34));
#39392=DIRECTION('center_axis',(-0.828419399070054,1.34310750335009E-16,
-0.560108292426036));
#39393=DIRECTION('ref_axis',(0.560108292426036,6.83578973261393E-31,-0.828419399070054));
#39394=DIRECTION('center_axis',(-6.43747505554034E-17,-1.,-6.27537777746355E-17));
#39395=DIRECTION('ref_axis',(0.698033961608026,0.,-0.716064653814029));
#39396=DIRECTION('center_axis',(0.716064653814028,-8.99007515774035E-17,
0.698033961608027));
#39397=DIRECTION('ref_axis',(0.698033961608027,-7.96736102322353E-31,-0.716064653814028));
#39398=DIRECTION('center_axis',(-2.44929359829E-16,-1.,1.22464679915E-16));
#39399=DIRECTION('ref_axis',(1.,-2.44929359829E-16,2.99951956532443E-32));
#39400=DIRECTION('center_axis',(0.716064653814028,-8.99007515774036E-17,
0.698033961608027));
#39401=DIRECTION('ref_axis',(0.698033961608027,-4.9741364910786E-33,-0.716064653814028));
#39402=DIRECTION('center_axis',(0.716064653814028,-8.99007515774035E-17,
0.698033961608027));
#39403=DIRECTION('ref_axis',(0.698033961608027,-7.96736102322353E-31,-0.716064653814028));
#39404=DIRECTION('',(0.716064653814028,0.,0.698033961608027));
#39405=DIRECTION('center_axis',(-6.43747505554034E-17,-1.,-6.27537777746355E-17));
#39406=DIRECTION('ref_axis',(-0.698033961608025,0.,0.71606465381403));
#39407=DIRECTION('center_axis',(-0.698033961608027,2.5866163998301E-16,
0.716064653814028));
#39408=DIRECTION('ref_axis',(0.716064653814028,2.30891390163356E-30,0.698033961608027));
#39409=DIRECTION('center_axis',(2.44929359829E-16,1.,-1.22464679915E-16));
#39410=DIRECTION('ref_axis',(1.,-2.44929359829E-16,2.99951956532444E-32));
#39411=DIRECTION('center_axis',(-0.698033961608027,2.5866163998301E-16,
0.716064653814028));
#39412=DIRECTION('ref_axis',(0.716064653814028,2.30891390163356E-30,0.698033961608027));
#39413=DIRECTION('center_axis',(-0.698033961608027,2.5866163998301E-16,
0.716064653814028));
#39414=DIRECTION('ref_axis',(0.716064653814028,2.30891390163356E-30,0.698033961608027));
#39415=DIRECTION('',(-0.698033961608027,0.,0.716064653814028));
#39416=DIRECTION('center_axis',(-1.80554609273596E-16,-1.,1.85218457689635E-16));
#39417=DIRECTION('ref_axis',(-0.71606465381403,0.,-0.698033961608025));
#39418=DIRECTION('center_axis',(-0.716064653814028,8.99007515774035E-17,
-0.698033961608027));
#39419=DIRECTION('ref_axis',(0.698033961608027,-2.36964484828339E-31,-0.716064653814028));
#39420=DIRECTION('center_axis',(2.44929359829E-16,1.,-1.22464679915E-16));
#39421=DIRECTION('ref_axis',(1.,-2.44929359829E-16,2.99951956532444E-32));
#39422=DIRECTION('center_axis',(0.716064653814028,-8.99007515767179E-17,
0.698033961608027));
#39423=DIRECTION('ref_axis',(6.43747505554034E-17,1.,6.27537777746355E-17));
#39424=DIRECTION('center_axis',(-0.716064653814028,8.99007515773035E-17,
-0.698033961608027));
#39425=DIRECTION('ref_axis',(0.698033961608027,-8.0031308366142E-31,-0.716064653814028));
#39426=DIRECTION('',(-0.716064653814028,0.,-0.698033961608027));
#39427=DIRECTION('center_axis',(-1.32057957382078E-16,-1.,1.9781552453987E-16));
#39428=DIRECTION('ref_axis',(0.831699011544245,0.,0.555226759258166));
#39429=DIRECTION('center_axis',(-0.555226759258164,2.37845087940071E-16,
0.831699011544246));
#39430=DIRECTION('ref_axis',(0.831699011544246,1.10558455272238E-30,0.555226759258164));
#39431=DIRECTION('center_axis',(-2.44929359829E-16,-1.,1.22464679915E-16));
#39432=DIRECTION('ref_axis',(1.,-2.44929359829E-16,2.99951956532443E-32));
#39433=DIRECTION('center_axis',(-9.88589466193077E-17,-1.,1.96101782897063E-16));
#39434=DIRECTION('ref_axis',(0.892950553792926,0.,0.450154760588963));
#39435=DIRECTION('center_axis',(-0.450154760588963,2.19611021084982E-16,
0.892950553792926));
#39436=DIRECTION('ref_axis',(0.892950553792926,5.80220876798355E-31,0.450154760588963));
#39437=DIRECTION('center_axis',(-2.44929359829E-16,-1.,1.22464679915E-16));
#39438=DIRECTION('ref_axis',(1.,-2.44929359829E-16,6.68589598176748E-33));
#39439=DIRECTION('center_axis',(-4.0788932203553E-30,-1.,1.22464679915008E-16));
#39440=DIRECTION('ref_axis',(1.,0.,3.37507799486048E-14));
#39441=DIRECTION('center_axis',(-4.47194436842E-16,1.22464679915E-16,1.));
#39442=DIRECTION('ref_axis',(1.,5.47655235676242E-32,4.47194436842E-16));
#39443=DIRECTION('center_axis',(-2.44929359829E-16,-1.,1.22464679915E-16));
#39444=DIRECTION('ref_axis',(1.,-2.44929359829E-16,2.99951956532444E-32));
#39445=DIRECTION('center_axis',(4.47194436842E-16,-1.22464679915E-16,-1.));
#39446=DIRECTION('ref_axis',(2.22237178326514E-45,1.,-1.22464679915E-16));
#39447=DIRECTION('center_axis',(2.62012633812E-14,1.22464679915E-16,1.));
#39448=DIRECTION('ref_axis',(1.,-2.2094004949211E-32,-2.62012633812E-14));
#39449=DIRECTION('',(-3.84360635984E-16,0.,1.));
#39450=DIRECTION('center_axis',(-4.05685585531587E-19,-1.,-8.04739169685281E-19));
#39451=DIRECTION('ref_axis',(0.892950553792926,0.,-0.450154760588964));
#39452=DIRECTION('center_axis',(0.450154760588963,-9.01213585416925E-19,
0.892950553792926));
#39453=DIRECTION('ref_axis',(0.892950553792926,2.40393060631611E-33,-0.450154760588963));
#39454=DIRECTION('center_axis',(-2.44929359829E-16,-1.,1.22464679915E-16));
#39455=DIRECTION('ref_axis',(1.,-2.44929359829E-16,2.99951956532444E-32));
#39456=DIRECTION('center_axis',(-3.92977953786766E-16,-1.,2.21299161975131E-16));
#39457=DIRECTION('ref_axis',(0.831699011544246,-4.46882223748491E-16,-0.555226759258164));
#39458=DIRECTION('center_axis',(0.555226759258164,-3.41375814712101E-17,
0.831699011544246));
#39459=DIRECTION('ref_axis',(0.831699011544246,1.57834305747204E-31,-0.555226759258164));
#39460=DIRECTION('center_axis',(-2.44929359829E-16,-1.,1.22464679915E-16));
#39461=DIRECTION('ref_axis',(1.,-2.44929359829E-16,6.68589598176748E-33));
#39462=DIRECTION('center_axis',(-1.86799616485145E-16,-1.,1.82095954083848E-16));
#39463=DIRECTION('ref_axis',(-0.698033961608026,0.,-0.716064653814029));
#39464=DIRECTION('center_axis',(0.716064653814028,-2.6086976293301E-16,
-0.698033961608027));
#39465=DIRECTION('ref_axis',(0.698033961608027,-2.32071020223926E-30,0.716064653814028));
#39466=DIRECTION('center_axis',(-2.44929359829E-16,-1.,1.22464679915E-16));
#39467=DIRECTION('ref_axis',(1.,-2.44929359829E-16,2.99951956532443E-32));
#39468=DIRECTION('center_axis',(0.716064653814028,-2.6086976293301E-16,
-0.698033961608027));
#39469=DIRECTION('ref_axis',(-0.698033961608027,1.10143058876371E-32,-0.716064653814028));
#39470=DIRECTION('center_axis',(0.716064653814515,-2.60869762932824E-16,
-0.698033961607527));
#39471=DIRECTION('ref_axis',(0.698033961607527,-1.04004355553456E-30,0.716064653814515));
#39472=DIRECTION('',(0.716064653814028,0.,-0.698033961608027));
#39473=DIRECTION('center_axis',(-1.86799616485145E-16,-1.,1.82095954083848E-16));
#39474=DIRECTION('ref_axis',(0.698033961608026,0.,0.716064653814029));
#39475=DIRECTION('center_axis',(0.698033961608027,-8.32763827281032E-17,
0.716064653814028));
#39476=DIRECTION('ref_axis',(0.716064653814028,7.37176741734741E-31,-0.698033961608027));
#39477=DIRECTION('center_axis',(2.44929359829E-16,1.,-1.22464679915E-16));
#39478=DIRECTION('ref_axis',(1.,-2.44929359829E-16,2.99951956532444E-32));
#39479=DIRECTION('center_axis',(-0.698033961608027,8.32763827277746E-17,
-0.716064653814028));
#39480=DIRECTION('ref_axis',(5.81297433438548E-17,1.,5.96312741688484E-17));
#39481=DIRECTION('center_axis',(0.698033961608027,-8.32763827281032E-17,
0.716064653814028));
#39482=DIRECTION('ref_axis',(0.716064653814028,7.37176741734741E-31,-0.698033961608027));
#39483=DIRECTION('',(0.698033961608027,0.,0.716064653814028));
#39484=DIRECTION('center_axis',(-5.81297433438548E-17,-1.,-5.96312741688484E-17));
#39485=DIRECTION('ref_axis',(-0.71606465381403,0.,0.698033961608025));
#39486=DIRECTION('center_axis',(-0.716064653814028,2.6086976293301E-16,
0.698033961608027));
#39487=DIRECTION('ref_axis',(0.698033961608027,-2.32071020223926E-30,0.716064653814028));
#39488=DIRECTION('center_axis',(2.44929359829E-16,1.,-1.22464679915E-16));
#39489=DIRECTION('ref_axis',(1.,-2.44929359829E-16,2.99951956532444E-32));
#39490=DIRECTION('center_axis',(0.716064653814028,-2.60869762932971E-16,
-0.698033961608027));
#39491=DIRECTION('ref_axis',(1.86799616485145E-16,1.,-1.82095954083849E-16));
#39492=DIRECTION('center_axis',(-0.716064653814515,2.60869762932824E-16,
0.698033961607527));
#39493=DIRECTION('ref_axis',(0.698033961607527,-2.6232605074812E-30,0.716064653814515));
#39494=DIRECTION('',(-0.716064653814028,0.,0.698033961608027));
#39495=DIRECTION('center_axis',(-1.02392142274414E-16,-1.,-7.42080178237726E-17));
#39496=DIRECTION('ref_axis',(0.586831315816962,0.,-0.809709211245946));
#39497=DIRECTION('center_axis',(0.809709211245947,-1.26455449502992E-16,
0.586831315816962));
#39498=DIRECTION('ref_axis',(0.586831315816962,-6.48713419669698E-31,-0.809709211245947));
#39499=DIRECTION('center_axis',(-2.44929359829E-16,-1.,1.22464679915E-16));
#39500=DIRECTION('ref_axis',(1.,-2.44929359829E-16,2.99951956532443E-32));
#39501=DIRECTION('center_axis',(-2.18773443555785E-16,-1.,1.58554584738017E-16));
#39502=DIRECTION('ref_axis',(-0.586831315816962,0.,-0.809709211245947));
#39503=DIRECTION('center_axis',(0.809709211245947,-2.70187668013982E-16,
-0.586831315816962));
#39504=DIRECTION('ref_axis',(0.586831315816962,-1.3944828999061E-30,0.809709211245947));
#39505=DIRECTION('center_axis',(-2.44929359829E-16,-1.,1.22464679915E-16));
#39506=DIRECTION('ref_axis',(1.,-2.44929359829E-16,6.68589598176748E-33));
#39507=DIRECTION('center_axis',(-6.43747505554034E-17,-1.,-6.27537777746355E-17));
#39508=DIRECTION('ref_axis',(-0.698033961608026,0.,0.716064653814029));
#39509=DIRECTION('center_axis',(-0.716064653814028,8.99007515774035E-17,
-0.698033961608027));
#39510=DIRECTION('ref_axis',(0.698033961608027,-7.96736102322353E-31,-0.716064653814028));
#39511=DIRECTION('center_axis',(-2.44929359829E-16,-1.,1.22464679915E-16));
#39512=DIRECTION('ref_axis',(1.,-2.44929359829E-16,2.99951956532443E-32));
#39513=DIRECTION('center_axis',(-0.716064653814028,8.99007515774035E-17,
-0.698033961608027));
#39514=DIRECTION('ref_axis',(-0.698033961608027,2.4644238743985E-33,0.716064653814028));
#39515=DIRECTION('center_axis',(-0.716064653814028,8.99007515774035E-17,
-0.698033961608027));
#39516=DIRECTION('ref_axis',(0.698033961608027,-7.96736102322353E-31,-0.716064653814028));
#39517=DIRECTION('',(-0.716064653814028,0.,-0.698033961608027));
#39518=DIRECTION('center_axis',(-6.43747505554034E-17,-1.,-6.27537777746355E-17));
#39519=DIRECTION('ref_axis',(0.698033961608025,0.,-0.71606465381403));
#39520=DIRECTION('center_axis',(0.698033961608027,-2.5866163998301E-16,
-0.716064653814028));
#39521=DIRECTION('ref_axis',(0.716064653814028,2.30891390163356E-30,0.698033961608027));
#39522=DIRECTION('center_axis',(2.44929359829E-16,1.,-1.22464679915E-16));
#39523=DIRECTION('ref_axis',(1.,-2.44929359829E-16,2.99951956532444E-32));
#39524=DIRECTION('center_axis',(0.698033961608027,-2.5866163998301E-16,
-0.716064653814028));
#39525=DIRECTION('ref_axis',(-0.716064653814028,-2.30891390163356E-30,-0.698033961608027));
#39526=DIRECTION('center_axis',(0.698033961608027,-2.5866163998301E-16,
-0.716064653814028));
#39527=DIRECTION('ref_axis',(0.716064653814028,2.30891390163356E-30,0.698033961608027));
#39528=DIRECTION('',(0.698033961608027,0.,-0.716064653814028));
#39529=DIRECTION('center_axis',(-1.80554609273596E-16,-1.,1.85218457689635E-16));
#39530=DIRECTION('ref_axis',(0.71606465381403,0.,0.698033961608025));
#39531=DIRECTION('center_axis',(0.716064653814028,-8.99007515774035E-17,
0.698033961608027));
#39532=DIRECTION('ref_axis',(0.698033961608027,-2.36964484828339E-31,-0.716064653814028));
#39533=DIRECTION('center_axis',(2.44929359829E-16,1.,-1.22464679915E-16));
#39534=DIRECTION('ref_axis',(1.,-2.44929359829E-16,2.99951956532444E-32));
#39535=DIRECTION('center_axis',(-0.716064653814028,8.99007515767179E-17,
-0.698033961608027));
#39536=DIRECTION('ref_axis',(6.43747505554034E-17,1.,6.27537777746355E-17));
#39537=DIRECTION('center_axis',(0.716064653814028,-8.99007515774035E-17,
0.698033961608027));
#39538=DIRECTION('ref_axis',(0.698033961608027,-7.96736102322353E-31,-0.716064653814028));
#39539=DIRECTION('',(0.716064653814028,0.,0.698033961608027));
#39540=DIRECTION('center_axis',(-1.32057957382078E-16,-1.,1.9781552453987E-16));
#39541=DIRECTION('ref_axis',(-0.831699011544245,0.,-0.555226759258166));
#39542=DIRECTION('center_axis',(0.555226759258164,-2.37845087940071E-16,
-0.831699011544246));
#39543=DIRECTION('ref_axis',(0.831699011544246,1.10558455272238E-30,0.555226759258164));
#39544=DIRECTION('center_axis',(-2.44929359829E-16,-1.,1.22464679915E-16));
#39545=DIRECTION('ref_axis',(1.,-2.44929359829E-16,2.99951956532443E-32));
#39546=DIRECTION('center_axis',(-9.88589466193077E-17,-1.,1.96101782897063E-16));
#39547=DIRECTION('ref_axis',(-0.892950553792926,0.,-0.450154760588963));
#39548=DIRECTION('center_axis',(0.450154760588963,-2.19611021084982E-16,
-0.892950553792926));
#39549=DIRECTION('ref_axis',(0.892950553792926,5.80220876798355E-31,0.450154760588963));
#39550=DIRECTION('center_axis',(-2.44929359829E-16,-1.,1.22464679915E-16));
#39551=DIRECTION('ref_axis',(1.,-2.44929359829E-16,5.91180967883826E-34));
#39552=DIRECTION('center_axis',(-1.35963107345579E-30,-1.,1.22464679915003E-16));
#39553=DIRECTION('ref_axis',(-1.,0.,-1.06581410364015E-14));
#39554=DIRECTION('center_axis',(2.87593642646E-16,-1.22464679915E-16,-1.));
#39555=DIRECTION('ref_axis',(1.,3.52200633922313E-32,2.87593642646E-16));
#39556=DIRECTION('center_axis',(-2.44929359829E-16,-1.,1.22464679915E-16));
#39557=DIRECTION('ref_axis',(1.,-2.44929359829E-16,2.99951956532444E-32));
#39558=DIRECTION('center_axis',(2.87593642646E-16,-1.22464679915E-16,-1.));
#39559=DIRECTION('ref_axis',(-1.,-1.10148049272531E-46,-2.87593642646E-16));
#39560=DIRECTION('center_axis',(-1.74860126378E-14,-1.22464679915E-16,-1.));
#39561=DIRECTION('ref_axis',(1.,-1.6995388412451E-32,-1.74860126378E-14));
#39562=DIRECTION('',(3.84360635984E-16,0.,-1.));
#39563=DIRECTION('center_axis',(-4.05685585531587E-19,-1.,-8.04739169685281E-19));
#39564=DIRECTION('ref_axis',(-0.892950553792926,0.,0.450154760588964));
#39565=DIRECTION('center_axis',(-0.450154760588963,9.01213585422925E-19,
-0.892950553792926));
#39566=DIRECTION('ref_axis',(0.892950553792926,2.37605947729967E-33,-0.450154760588963));
#39567=DIRECTION('center_axis',(-2.44929359829E-16,-1.,1.22464679915E-16));
#39568=DIRECTION('ref_axis',(1.,-2.44929359829E-16,2.99951956532444E-32));
#39569=DIRECTION('center_axis',(-3.95305981663445E-16,-1.,2.15892490384474E-16));
#39570=DIRECTION('ref_axis',(-0.849410790431843,4.46882223748491E-16,0.527732232384902));
#39571=DIRECTION('center_axis',(-0.527732232384902,2.52342972731953E-17,
-0.849410790431843));
#39572=DIRECTION('ref_axis',(0.849410790431843,-6.27761689185242E-32,-0.527732232384902));
#39573=DIRECTION('center_axis',(-2.44929359829E-16,-1.,1.22464679915E-16));
#39574=DIRECTION('ref_axis',(1.,-2.44929359829E-16,5.91180967883826E-34));
#39575=DIRECTION('center_axis',(-1.86799616485314E-16,-1.,1.82095954083758E-16));
#39576=DIRECTION('ref_axis',(0.698033961607525,0.,0.716064653814517));
#39577=DIRECTION('center_axis',(-0.716064653814028,2.6086976293301E-16,
0.698033961608027));
#39578=DIRECTION('ref_axis',(0.698033961608027,-2.32071020223926E-30,0.716064653814028));
#39579=DIRECTION('center_axis',(-2.44929359829E-16,-1.,1.22464679915E-16));
#39580=DIRECTION('ref_axis',(1.,-2.44929359829E-16,2.99951956532443E-32));
#39581=DIRECTION('center_axis',(-0.716064653814028,2.6086976293301E-16,
0.698033961608027));
#39582=DIRECTION('ref_axis',(0.698033961608027,1.0524566385888E-31,0.716064653814028));
#39583=DIRECTION('center_axis',(-0.716064653814028,2.6086976293301E-16,
0.698033961608027));
#39584=DIRECTION('ref_axis',(0.698033961608027,-7.02188537105379E-31,0.716064653814028));
#39585=DIRECTION('',(-0.716064653814028,0.,0.698033961608027));
#39586=DIRECTION('center_axis',(-1.86799616485145E-16,-1.,1.82095954083848E-16));
#39587=DIRECTION('ref_axis',(-0.698033961608026,0.,-0.716064653814029));
#39588=DIRECTION('center_axis',(-0.698033961608027,8.32763827281032E-17,
-0.716064653814028));
#39589=DIRECTION('ref_axis',(0.716064653814028,7.37176741734741E-31,-0.698033961608027));
#39590=DIRECTION('center_axis',(2.44929359829E-16,1.,-1.22464679915E-16));
#39591=DIRECTION('ref_axis',(1.,-2.44929359829E-16,2.99951956532444E-32));
#39592=DIRECTION('center_axis',(0.698033961608027,-8.32763827277746E-17,
0.716064653814028));
#39593=DIRECTION('ref_axis',(5.81297433438548E-17,1.,5.96312741688484E-17));
#39594=DIRECTION('center_axis',(-0.698033961607527,8.32763827280436E-17,
-0.716064653814515));
#39595=DIRECTION('ref_axis',(0.716064653814515,3.35409891176131E-31,-0.698033961607527));
#39596=DIRECTION('',(-0.698033961608027,0.,-0.716064653814028));
#39597=DIRECTION('center_axis',(-1.11265631080723E-16,-1.,-7.52285650242949E-17));
#39598=DIRECTION('ref_axis',(-0.560108292426038,0.,0.828419399070053));
#39599=DIRECTION('center_axis',(-2.44929359829E-16,-1.,1.22464679915E-16));
#39600=DIRECTION('ref_axis',(1.,-2.44929359829E-16,2.99951956532443E-32));
#39601=DIRECTION('center_axis',(0.716064653814028,-2.6086976293301E-16,
-0.698033961608027));
#39602=DIRECTION('ref_axis',(0.698033961608027,-2.32071020223926E-30,0.716064653814028));
#39603=DIRECTION('center_axis',(-5.81297433438548E-17,-1.,-5.96312741688484E-17));
#39604=DIRECTION('ref_axis',(0.716064653814029,0.,-0.698033961608026));
#39605=DIRECTION('center_axis',(0.716064653814028,-2.6086976293301E-16,
-0.698033961608027));
#39606=DIRECTION('ref_axis',(0.698033961608027,-2.32071020223926E-30,0.716064653814028));
#39607=DIRECTION('center_axis',(2.44929359829E-16,1.,-1.22464679915E-16));
#39608=DIRECTION('ref_axis',(1.,-2.44929359829E-16,2.99951956532443E-32));
#39609=DIRECTION('center_axis',(-0.716064653814028,2.60869762932971E-16,
0.698033961608027));
#39610=DIRECTION('ref_axis',(1.86799616485145E-16,1.,-1.82095954083849E-16));
#39611=DIRECTION('',(0.716064653814028,0.,-0.698033961608027));
#39612=DIRECTION('center_axis',(-2.44929359829E-16,-1.,1.22464679915E-16));
#39613=DIRECTION('ref_axis',(-1.,2.44929359829E-16,0.));
#39614=DIRECTION('',(0.716064653814028,0.,0.698033961608027));
#39615=DIRECTION('center_axis',(-2.44929359829E-16,-1.,1.22464679915E-16));
#39616=DIRECTION('ref_axis',(1.,-2.44929359829E-16,2.99951956532444E-32));
#39617=DIRECTION('',(-0.698033961608027,0.,0.716064653814028));
#39618=DIRECTION('center_axis',(-2.44929359829E-16,-1.,1.22464679915E-16));
#39619=DIRECTION('ref_axis',(1.,-2.44929359829E-16,2.99951956532444E-32));
#39620=DIRECTION('',(0.716064653814028,0.,0.698033961608027));
#39621=DIRECTION('center_axis',(2.44929359829E-16,1.,-1.22464679915E-16));
#39622=DIRECTION('ref_axis',(1.,-2.44929359829E-16,9.78625965784287E-34));
#39623=DIRECTION('',(-0.716064653814028,0.,0.698033961608027));
#39624=DIRECTION('center_axis',(-2.44929359829E-16,-1.,1.22464679915E-16));
#39625=DIRECTION('ref_axis',(1.,-2.44929359829E-16,2.99951956532444E-32));
#39626=DIRECTION('',(0.698033961608027,0.,0.716064653814028));
#39627=DIRECTION('center_axis',(-2.32604145439E-16,-1.,1.36266007238E-16));
#39628=DIRECTION('ref_axis',(1.,-2.32604145439E-16,3.16960381659796E-32));
#39629=DIRECTION('center_axis',(-2.44929359829E-16,-1.,1.22464679915E-16));
#39630=DIRECTION('ref_axis',(1.,-2.44929359829E-16,2.99951956532444E-32));
#39631=DIRECTION('',(0.698033961608027,0.,-0.716064653814028));
#39632=DIRECTION('center_axis',(-2.44929359829E-16,-1.,1.22464679915E-16));
#39633=DIRECTION('ref_axis',(1.,-2.44929359829E-16,2.99951956532444E-32));
#39634=DIRECTION('',(-0.716064653814028,0.,-0.698033961608027));
#39635=DIRECTION('center_axis',(-2.44929359829E-16,-1.,1.22464679915E-16));
#39636=DIRECTION('ref_axis',(1.,-2.44929359829E-16,9.78625965784287E-34));
#39637=DIRECTION('',(0.716064653814028,0.,-0.698033961608027));
#39638=DIRECTION('center_axis',(-2.44929359829E-16,-1.,1.22464679915E-16));
#39639=DIRECTION('ref_axis',(1.,-2.44929359829E-16,2.99951956532444E-32));
#39640=DIRECTION('',(-0.698033961608027,0.,-0.716064653814028));
#39641=DIRECTION('center_axis',(-2.44929359829E-16,-1.,1.22464679915E-16));
#39642=DIRECTION('ref_axis',(1.,-2.44929359829E-16,2.99951956532444E-32));
#39643=DIRECTION('center_axis',(2.44929359828964E-16,1.,-1.22464679914979E-16));
#39644=DIRECTION('ref_axis',(-0.860090783657011,2.73135739791003E-16,0.510141003908006));
#39645=DIRECTION('',(-3.70074341542E-16,-1.,0.));
#39646=DIRECTION('',(-3.70074341542E-16,-1.,0.));
#39647=DIRECTION('center_axis',(0.,-1.,0.));
#39648=DIRECTION('ref_axis',(0.503074672515737,0.,-0.864242948408133));
#39649=DIRECTION('center_axis',(0.698033961608027,-2.5866163998301E-16,
-0.716064653814028));
#39650=DIRECTION('ref_axis',(-5.0987642944624E-33,-1.,3.6122665544973E-16));
#39651=DIRECTION('',(0.716064653824126,0.,0.698033961597667));
#39652=DIRECTION('',(0.,-1.,0.));
#39653=DIRECTION('center_axis',(-0.698033961608027,8.32763827281032E-17,
-0.716064653814028));
#39654=DIRECTION('ref_axis',(-0.716064653814028,-6.03301243078373E-33,0.698033961608027));
#39655=DIRECTION('',(0.716064653821144,0.,-0.698033961600728));
#39656=DIRECTION('',(0.,-1.,0.));
#39657=DIRECTION('center_axis',(-2.44929359829028E-16,-1.,1.22464679915027E-16));
#39658=DIRECTION('ref_axis',(-0.716064653814028,2.6086976293301E-16,0.698033961608027));
#39659=DIRECTION('center_axis',(0.,1.,0.));
#39660=DIRECTION('ref_axis',(-0.716064653820949,0.,0.698033961600927));
#39661=DIRECTION('',(-3.70074341542E-16,-1.,0.));
#39662=DIRECTION('center_axis',(-0.716064653814028,2.6086976293301E-16,
0.698033961608027));
#39663=DIRECTION('ref_axis',(3.64310347597135E-16,1.,-2.26745038145461E-32));
#39664=DIRECTION('',(-0.698033961612045,0.,-0.716064653810111));
#39665=DIRECTION('',(0.,-1.,0.));
#39666=DIRECTION('center_axis',(-2.44929359829229E-16,-1.,1.22464679914765E-16));
#39667=DIRECTION('ref_axis',(0.698033961608027,-8.32763827281033E-17,0.716064653814028));
#39668=DIRECTION('center_axis',(0.,1.,0.));
#39669=DIRECTION('ref_axis',(0.698033961600926,0.,0.71606465382095));
#39670=DIRECTION('center_axis',(0.716064653814028,-8.99007515774035E-17,
0.698033961608027));
#39671=DIRECTION('ref_axis',(-2.12219958443594E-33,-1.,-1.28791371941708E-16));
#39672=DIRECTION('',(0.,-1.,0.));
#39673=DIRECTION('',(-0.698033961612045,0.,0.716064653810111));
#39674=DIRECTION('',(0.,-1.,0.));
#39675=DIRECTION('center_axis',(-2.44929359829491E-16,-1.,1.22464679914521E-16));
#39676=DIRECTION('ref_axis',(-0.716064653814028,8.99007515774037E-17,-0.698033961608027));
#39677=DIRECTION('center_axis',(0.,1.,0.));
#39678=DIRECTION('ref_axis',(-0.716064653804541,0.,-0.698033961617759));
#39679=DIRECTION('center_axis',(-2.44929359828773E-16,-1.,1.22464679914767E-16));
#39680=DIRECTION('ref_axis',(-0.698033961608027,2.5866163998301E-16,0.716064653814028));
#39681=DIRECTION('center_axis',(0.,1.,0.));
#39682=DIRECTION('ref_axis',(-0.698033961584438,0.,0.716064653837023));
#39683=DIRECTION('',(-3.70074341542E-16,-1.,0.));
#39684=DIRECTION('center_axis',(0.698033961608027,-2.5866163998301E-16,
-0.716064653814028));
#39685=DIRECTION('ref_axis',(-5.0987642944624E-33,-1.,3.6122665544973E-16));
#39686=DIRECTION('',(0.716064653821144,0.,0.698033961600728));
#39687=DIRECTION('',(-3.70074341542E-16,-1.,0.));
#39688=DIRECTION('center_axis',(2.44929359828964E-16,1.,-1.22464679914979E-16));
#39689=DIRECTION('ref_axis',(-0.860090783657011,2.73135739791003E-16,0.510141003908006));
#39690=DIRECTION('center_axis',(0.,-1.,0.));
#39691=DIRECTION('ref_axis',(-4.52175312758849E-15,0.,1.));
#39692=DIRECTION('',(-3.70074341542E-16,-1.,0.));
#39693=DIRECTION('center_axis',(-0.698033961608027,2.5866163998301E-16,
0.716064653814028));
#39694=DIRECTION('ref_axis',(3.70557385756911E-16,1.,-1.7912467654698E-32));
#39695=DIRECTION('',(0.,-1.,0.));
#39696=DIRECTION('',(-0.716064653821144,0.,-0.698033961600728));
#39697=DIRECTION('center_axis',(-2.44929359828773E-16,-1.,1.22464679914767E-16));
#39698=DIRECTION('ref_axis',(0.698033961608027,-2.5866163998301E-16,-0.716064653814028));
#39699=DIRECTION('center_axis',(0.,1.,0.));
#39700=DIRECTION('ref_axis',(0.698033961584438,0.,-0.716064653837023));
#39701=DIRECTION('',(-3.70074341542E-16,-1.,0.));
#39702=DIRECTION('center_axis',(-0.716064653814028,8.99007515774035E-17,
-0.698033961608027));
#39703=DIRECTION('ref_axis',(-0.698033961608027,-3.69855194764065E-33,0.716064653814028));
#39704=DIRECTION('',(0.,-1.,0.));
#39705=DIRECTION('',(0.698033961612045,0.,-0.716064653810111));
#39706=DIRECTION('center_axis',(-2.32604145438773E-16,-1.,1.36266007238254E-16));
#39707=DIRECTION('ref_axis',(-0.666093971259166,5.32997876968134E-17,-0.745867831088185));
#39708=DIRECTION('center_axis',(0.,1.,0.));
#39709=DIRECTION('ref_axis',(-0.666093971264093,0.,-0.745867831083785));
#39710=DIRECTION('',(0.,-1.,0.));
#39711=DIRECTION('center_axis',(0.716064653814028,-2.6086976293301E-16,
-0.698033961608027));
#39712=DIRECTION('ref_axis',(-1.38053841875249E-32,-1.,3.73720731770783E-16));
#39713=DIRECTION('',(0.,-1.,0.));
#39714=DIRECTION('',(0.698033961610687,0.,0.716064653811435));
#39715=DIRECTION('center_axis',(-2.44929359829028E-16,-1.,1.22464679915027E-16));
#39716=DIRECTION('ref_axis',(0.716064653814028,-2.6086976293301E-16,-0.698033961608027));
#39717=DIRECTION('center_axis',(0.,1.,0.));
#39718=DIRECTION('ref_axis',(0.7160646538177,0.,-0.69803396160426));
#39719=DIRECTION('',(0.,-1.,0.));
#39720=DIRECTION('center_axis',(0.698033961608027,-8.32763827281032E-17,
0.716064653814028));
#39721=DIRECTION('ref_axis',(-1.19301333901095E-16,-1.,6.93490090905032E-33));
#39722=DIRECTION('',(-0.716064653924687,0.,0.698033961494509));
#39723=DIRECTION('',(-0.326298438494934,0.943819486756767,0.0522886742417565));
#39724=DIRECTION('',(-0.128571714532246,0.968939478859869,0.211247723133303));
#39725=DIRECTION('',(-0.330975706838633,0.943531527766579,0.0142596491237413));
#39726=DIRECTION('center_axis',(-0.943627470111708,-0.331009361877541,0.));
#39727=DIRECTION('ref_axis',(0.,0.,1.));
#39728=DIRECTION('',(-0.323037326396155,0.920901128988691,-0.218146731312158));
#39729=DIRECTION('',(1.64651774315771E-16,0.,-1.));
#39730=DIRECTION('',(-0.294062932800905,0.911816425322849,-0.286562031790662));
#39731=DIRECTION('',(-0.310424970358247,0.909870545905898,-0.27526701122907));
#39732=DIRECTION('',(0.288992183012555,0.946290745989702,0.144973591429235));
#39733=DIRECTION('',(0.288070798801296,0.943889906160958,0.161514890723551));
#39734=DIRECTION('',(0.185892369076962,0.87281982032212,0.451253352754101));
#39735=DIRECTION('',(0.225419688153596,0.803501199046223,0.550973490581913));
#39736=DIRECTION('',(0.25532881023728,0.774608545942306,0.578609366685298));
#39737=DIRECTION('center_axis',(-4.57218787640431E-10,-1.,-8.71360109757879E-11));
#39738=DIRECTION('ref_axis',(0.980286226483734,-4.65421893024152E-10,0.197582676786912));
#39739=DIRECTION('center_axis',(-2.44929359829491E-16,-1.,1.22464679914521E-16));
#39740=DIRECTION('ref_axis',(0.716064653814028,-8.99007515774037E-17,0.698033961608027));
#39741=DIRECTION('center_axis',(0.,1.,0.));
#39742=DIRECTION('ref_axis',(0.716064653804541,0.,0.698033961617759));
#39743=DIRECTION('center_axis',(-1.48089814433846E-9,-1.,1.36711158136743E-9));
#39744=DIRECTION('ref_axis',(0.738412059057248,-2.01542449026607E-9,-0.674349783894705));
#39745=DIRECTION('',(0.326298438494934,0.943819486756767,0.0522886742417565));
#39746=DIRECTION('center_axis',(0.33738697816179,0.0208183480491995,0.941135815571461));
#39747=DIRECTION('ref_axis',(0.637783973074513,0.730279477783167,-0.244792745027368));
#39748=DIRECTION('center_axis',(0.126791036026689,-0.0184132777306928,0.991758531289997));
#39749=DIRECTION('ref_axis',(0.674495541553173,0.734701613202815,-0.0725899716357153));
#39750=DIRECTION('center_axis',(-0.703555295639302,0.00327031186878069,
0.710632993209699));
#39751=DIRECTION('ref_axis',(0.595284509769511,0.548878148649461,0.586829728595623));
#39752=DIRECTION('center_axis',(0.71100199103497,0.0109882068305169,0.703104137418461));
#39753=DIRECTION('ref_axis',(0.587718788382872,-0.558268880784424,-0.585595835478255));
#39754=DIRECTION('center_axis',(-2.44929359829021E-16,-1.,1.22464679914804E-16));
#39755=DIRECTION('ref_axis',(0.106227141118038,9.57536156315344E-17,0.994341890141358));
#39756=DIRECTION('',(2.22044604925E-16,1.,0.));
#39757=DIRECTION('center_axis',(2.44929359828927E-16,1.,-1.22464679914314E-16));
#39758=DIRECTION('ref_axis',(-0.106227141118038,1.47789906972053E-16,0.994341890141358));
#39759=DIRECTION('center_axis',(0.71100199103497,-0.0109882068305169,-0.703104137418461));
#39760=DIRECTION('ref_axis',(0.587718788382872,0.558268880784424,0.585595835478255));
#39761=DIRECTION('',(-4.22942104619E-16,-1.,0.));
#39762=DIRECTION('center_axis',(-2.44929359829277E-16,-1.,1.22464679915277E-16));
#39763=DIRECTION('ref_axis',(-0.70655827709904,2.59719592428015E-16,0.707654860128041));
#39764=DIRECTION('center_axis',(1.75424076978333E-8,1.,-1.21125590716001E-8));
#39765=DIRECTION('ref_axis',(-0.706558277096875,2.09662509575991E-8,0.707654860130201));
#39766=DIRECTION('',(0.,-1.,0.));
#39767=DIRECTION('center_axis',(-0.99784376475148,2.52439080557121E-16,
0.0656339938339316));
#39768=DIRECTION('ref_axis',(2.52984574814669E-16,1.,-1.76602436617594E-34));
#39769=DIRECTION('center_axis',(0.997843762826238,-1.07495452104656E-7,
-0.0656340231035873));
#39770=DIRECTION('ref_axis',(0.0543784369549279,-0.559973082837639,0.826724338635104));
#39771=DIRECTION('',(4.22942104619E-16,1.,-1.05735526155E-16));
#39772=DIRECTION('center_axis',(2.44929359829765E-16,1.,-1.2246467991505E-16));
#39773=DIRECTION('ref_axis',(0.99784376475148,-2.52439080557122E-16,-0.0656339938339316));
#39774=DIRECTION('center_axis',(0.992604832159675,-0.0967004534711314,-0.0733803071112495));
#39775=DIRECTION('ref_axis',(0.0892087136015431,0.991051361070216,-0.0992925230741472));
#39776=DIRECTION('',(2.96059473233E-16,1.,0.));
#39777=DIRECTION('center_axis',(-2.4492935982986E-16,-1.,1.22464679914313E-16));
#39778=DIRECTION('ref_axis',(-0.781375177526389,1.14956222701057E-16,-0.624061561022311));
#39779=DIRECTION('center_axis',(-0.762365462560859,-0.0521613879530353,
0.645041154579443));
#39780=DIRECTION('ref_axis',(0.181698336597197,-0.973905518778203,0.135991745967063));
#39781=DIRECTION('center_axis',(-0.762365462560859,0.0521613879530353,-0.645041154579443));
#39782=DIRECTION('ref_axis',(0.181698336597197,0.973905518778203,-0.135991745967063));
#39783=DIRECTION('',(4.22942104619E-16,1.,-1.05735526155E-16));
#39784=DIRECTION('center_axis',(-2.44929359829589E-16,-1.,1.22464679914961E-16));
#39785=DIRECTION('ref_axis',(-0.99784376475148,2.36363388464114E-16,-0.0656339938339316));
#39786=DIRECTION('center_axis',(0.992604832159675,0.0967004534711314,0.0733803071112495));
#39787=DIRECTION('ref_axis',(0.0892087136015431,-0.991051361070216,0.0992925230741472));
#39788=DIRECTION('',(0.,1.,-1.71536605105E-16));
#39789=DIRECTION('center_axis',(-0.99784376475148,2.36363388464114E-16,
-0.0656339938339316));
#39790=DIRECTION('ref_axis',(-0.0656339938339316,2.57699594238361E-34,0.99784376475148));
#39791=DIRECTION('center_axis',(0.997843762826238,1.07495452104656E-7,0.0656340231035873));
#39792=DIRECTION('ref_axis',(0.0543784369549279,0.559973082837639,-0.826724338635104));
#39793=DIRECTION('center_axis',(-0.065618044097648,-0.0267441093839493,
0.997486353241015));
#39794=DIRECTION('ref_axis',(0.827047674636938,0.557835994841529,0.0693624302976431));
#39795=DIRECTION('center_axis',(-0.0655782124791017,-0.0412186949466952,
0.996995745845958));
#39796=DIRECTION('ref_axis',(0.269397312004974,-0.962775872182078,-0.0220841171101169));
#39797=DIRECTION('center_axis',(-0.0856235883015126,0.0624824447695074,
0.994366403908538));
#39798=DIRECTION('ref_axis',(0.0924863865976304,-0.993223888733409,0.0703745347650614));
#39799=DIRECTION('center_axis',(0.979394141707147,0.188333569461664,0.0729217512375316));
#39800=DIRECTION('ref_axis',(-0.0989622241844842,0.132786699227001,0.986191751482874));
#39801=DIRECTION('center_axis',(-0.643311851218355,0.0453228721401247,0.764261538573663));
#39802=DIRECTION('ref_axis',(0.734064765060376,0.320083161313605,0.59891208915862));
#39803=DIRECTION('center_axis',(-0.645613117725507,0.00688651525632543,
0.763633602016291));
#39804=DIRECTION('ref_axis',(0.724253375877135,0.322609208678801,0.609409834188956));
#39805=DIRECTION('center_axis',(-1.,-3.05924483389283E-12,-3.74625528149392E-12));
#39806=DIRECTION('ref_axis',(-4.80001061146564E-12,0.722902978576062,0.690949552113508));
#39807=DIRECTION('center_axis',(-0.64561315170571,-0.00688562442483218,
-0.763633581320845));
#39808=DIRECTION('ref_axis',(-0.724253155294373,0.322609253942205,0.609410072379017));
#39809=DIRECTION('center_axis',(-0.643311852237848,-0.0453228719224639,
-0.76426153772842));
#39810=DIRECTION('ref_axis',(-0.734064763730816,0.320083163451923,0.598912089645409));
#39811=DIRECTION('center_axis',(-0.0855523090148687,-0.062489382877931,
-0.994372103113196));
#39812=DIRECTION('ref_axis',(0.0924776252402706,0.993224761345867,-0.0703737328792845));
#39813=DIRECTION('center_axis',(-0.065578227090674,0.0412186963935417,-0.996995744825052));
#39814=DIRECTION('ref_axis',(0.269393661471009,0.962776887229459,0.0220843966636586));
#39815=DIRECTION('center_axis',(0.979394141707147,-0.188333569461664,-0.0729217512375316));
#39816=DIRECTION('ref_axis',(-0.0989622241844842,-0.132786699227001,-0.986191751482874));
#39817=DIRECTION('center_axis',(-0.0656099521672813,0.0267416358010699,
-0.997486951840118));
#39818=DIRECTION('ref_axis',(-0.827048250379497,0.557836147395209,0.0693543380293116));
#39819=DIRECTION('center_axis',(-0.0594793722313762,0.422789020794831,-0.904274100134638));
#39820=DIRECTION('ref_axis',(0.998229534866085,0.025191826794196,-0.0538810503220736));
#39821=DIRECTION('center_axis',(-0.631948690569006,-0.772532669185509,-0.0619203321150045));
#39822=DIRECTION('ref_axis',(0.212600461685972,-0.249632918685971,0.944713951203874));
#39823=DIRECTION('center_axis',(-0.629471273307508,-0.456899628845233,-0.628497132246213));
#39824=DIRECTION('ref_axis',(-0.745283693861492,0.583835272272019,0.322007128050339));
#39825=DIRECTION('center_axis',(-0.703545043437849,-0.00327462087547922,
-0.710643123313071));
#39826=DIRECTION('ref_axis',(-0.595295187901339,0.548876942737332,0.58682002436252));
#39827=DIRECTION('center_axis',(0.126798015387979,0.0184102004931597,-0.991757696119103));
#39828=DIRECTION('ref_axis',(-0.674494684978775,0.734701710295614,-0.0725969477601046));
#39829=DIRECTION('center_axis',(0.337389367637308,-0.0208194531308848,-0.941134934521415));
#39830=DIRECTION('ref_axis',(-0.637783115038796,0.730279423602685,-0.244795142177984));
#39831=DIRECTION('',(0.70749274103932,0.681076592669504,0.188649665502934));
#39832=DIRECTION('',(-0.70749274103932,0.681076592669504,0.188649665502934));
#39833=DIRECTION('',(-0.724633338758358,0.67760887776062,0.125509892597787));
#39834=DIRECTION('center_axis',(4.6699357595302E-12,-1.,-1.22734079440797E-12));
#39835=DIRECTION('ref_axis',(-0.937281717636962,-3.94796067924408E-12,-0.348572778316818));
#39836=DIRECTION('',(-0.549972007288369,0.810772660219186,-0.20044571494623));
#39837=DIRECTION('center_axis',(0.,-1.,0.));
#39838=DIRECTION('ref_axis',(-0.845128221450091,0.,-0.534563643833553));
#39839=DIRECTION('',(-0.532777339634286,0.817212408304852,-0.219800332312754));
#39840=DIRECTION('center_axis',(0.,1.,0.));
#39841=DIRECTION('ref_axis',(-0.845112251565906,0.,-0.534588890880839));
#39842=DIRECTION('',(-0.158243927826022,0.930070177257986,-0.331554406819593));
#39843=DIRECTION('',(-0.126460756662279,0.930954528604445,-0.342536629713202));
#39844=DIRECTION('center_axis',(0.,-1.,0.));
#39845=DIRECTION('ref_axis',(0.633622560519774,0.,-0.773642327435854));
#39846=DIRECTION('',(-3.46493233997901E-14,0.690868651664906,-0.722980294438731));
#39847=DIRECTION('center_axis',(0.,-1.,0.));
#39848=DIRECTION('ref_axis',(-0.633782984477245,0.,-0.773510910451247));
#39849=DIRECTION('',(0.126460756667282,0.930954528602216,-0.342536629717412));
#39850=DIRECTION('center_axis',(-2.44519893085839E-16,1.,-2.75686781185422E-14));
#39851=DIRECTION('ref_axis',(0.633782984477227,-2.12111638737612E-14,-0.773510910451261));
#39852=DIRECTION('',(0.158243927826291,0.930070177257933,-0.331554406819613));
#39853=DIRECTION('center_axis',(0.,1.,0.));
#39854=DIRECTION('ref_axis',(0.633622560519774,0.,0.773642327435854));
#39855=DIRECTION('',(0.532777339638841,0.817212408301779,-0.219800332313137));
#39856=DIRECTION('',(0.54997200729065,0.810772660217083,-0.200445714948479));
#39857=DIRECTION('center_axis',(0.,-1.,0.));
#39858=DIRECTION('ref_axis',(0.845112251565906,0.,-0.534588890880839));
#39859=DIRECTION('',(0.724633338767814,0.677608877750319,0.125509892598804));
#39860=DIRECTION('center_axis',(0.,1.,0.));
#39861=DIRECTION('ref_axis',(0.845128221450091,0.,-0.534563643833553));
#39862=DIRECTION('center_axis',(4.6699357595302E-12,1.,1.22734079440797E-12));
#39863=DIRECTION('ref_axis',(0.937281717636962,-3.94796067924408E-12,-0.348572778316818));
#39864=DIRECTION('center_axis',(-2.44929359829E-16,-1.,1.22464679915E-16));
#39865=DIRECTION('ref_axis',(-1.,2.44929359829E-16,0.));
#39866=DIRECTION('center_axis',(-2.44929359829E-16,-1.,1.22464679915E-16));
#39867=DIRECTION('ref_axis',(1.,-2.44929359829E-16,2.99951956532443E-32));
#39868=DIRECTION('center_axis',(-2.44929359829E-16,-1.,1.22464679915E-16));
#39869=DIRECTION('ref_axis',(1.,-2.44929359829E-16,-2.25001164789147E-32));
#39870=DIRECTION('center_axis',(-2.44929359829E-16,-1.,1.22464679915E-16));
#39871=DIRECTION('ref_axis',(1.,-2.44929359829E-16,-2.35882174039441E-33));
#39872=DIRECTION('center_axis',(-2.44929359829E-16,-1.,1.22464679915E-16));
#39873=DIRECTION('ref_axis',(1.,-2.44929359829E-16,2.99951956532443E-32));
#39874=DIRECTION('center_axis',(2.44929359829E-16,1.,-1.22464679915E-16));
#39875=DIRECTION('ref_axis',(1.,-2.44929359829E-16,2.99951956532443E-32));
#39876=DIRECTION('center_axis',(2.44929359829E-16,1.,-1.22464679915E-16));
#39877=DIRECTION('ref_axis',(1.,-2.44929359829E-16,-2.35882174039442E-33));
#39878=DIRECTION('center_axis',(2.44929359829E-16,1.,-1.22464679915E-16));
#39879=DIRECTION('ref_axis',(1.,-2.44929359829E-16,-2.25001164789147E-32));
#39880=DIRECTION('center_axis',(-2.44929359829289E-16,-1.,1.22464679914817E-16));
#39881=DIRECTION('ref_axis',(-0.844952619998974,1.41454552433996E-16,-0.534841163296983));
#39882=DIRECTION('center_axis',(3.20197585381547E-15,-1.,5.00923523856943E-15));
#39883=DIRECTION('ref_axis',(-0.254396783383164,-5.76114676938621E-15,-0.967099931033138));
#39884=DIRECTION('',(0.,-1.,1.13869028167E-16));
#39885=DIRECTION('',(-3.9650822308E-16,-1.,0.));
#39886=DIRECTION('center_axis',(-2.44929359829546E-16,-1.,1.22464679915124E-16));
#39887=DIRECTION('ref_axis',(-0.975256647866936,2.65942952836982E-16,0.221075712802985));
#39888=DIRECTION('',(-4.55476112667E-16,-1.,2.27738056333E-16));
#39889=DIRECTION('center_axis',(1.27286491546545E-14,-1.,-7.63214849541229E-16));
#39890=DIRECTION('ref_axis',(-0.994685788780406,-1.25120668655344E-14,-0.102957183325405));
#39891=DIRECTION('center_axis',(-2.44929359828997E-16,-1.,1.22464679914357E-16));
#39892=DIRECTION('ref_axis',(-0.00535506551034943,1.23774536725987E-16,
0.999985661533894));
#39893=DIRECTION('',(-2.41971684854E-16,-1.,0.));
#39894=DIRECTION('center_axis',(1.42571546068487E-15,-1.,-2.56729319960534E-15));
#39895=DIRECTION('ref_axis',(-0.846038107384351,-2.53200862645747E-15,0.533122425764951));
#39896=DIRECTION('center_axis',(2.44929359829001E-16,1.,-1.22464679914941E-16));
#39897=DIRECTION('ref_axis',(0.00535506551034943,1.21151311191987E-16,0.999985661533894));
#39898=DIRECTION('center_axis',(0.,1.,0.));
#39899=DIRECTION('ref_axis',(0.846038107384351,0.,0.533122425764951));
#39900=DIRECTION('',(0.,-1.,0.));
#39901=DIRECTION('center_axis',(2.4492935982935E-16,1.,-1.22464679914921E-16));
#39902=DIRECTION('ref_axis',(0.975256647866936,-2.11795020025986E-16,0.221075712802985));
#39903=DIRECTION('center_axis',(-6.33314902666E-15,1.,-9.01543124247796E-16));
#39904=DIRECTION('ref_axis',(0.994685788780406,6.25603343276713E-15,-0.10295718332541));
#39905=DIRECTION('',(0.,-1.,0.));
#39906=DIRECTION('center_axis',(2.44929359829233E-16,1.,-1.22464679915147E-16));
#39907=DIRECTION('ref_axis',(0.844952619998974,-2.72452856170991E-16,-0.534841163296983));
#39908=DIRECTION('center_axis',(0.,1.,0.));
#39909=DIRECTION('ref_axis',(0.254396783383163,0.,-0.967099931033138));
#39910=DIRECTION('',(-3.9650822308E-16,-1.,0.));
#39911=DIRECTION('center_axis',(2.44929359828916E-16,1.,-1.22464679914681E-16));
#39912=DIRECTION('ref_axis',(0.254396783383044,-1.80744824796032E-16,-0.967099931033169));
#39913=DIRECTION('center_axis',(0.,1.,0.));
#39914=DIRECTION('ref_axis',(-0.254396783384328,0.,-0.967099931032832));
#39915=DIRECTION('center_axis',(-2.44929359829E-16,-1.,1.22464679915E-16));
#39916=DIRECTION('ref_axis',(-1.,2.44929359829E-16,0.));
#49130=CARTESIAN_POINT('',(0.,0.,0.));
#49131=CARTESIAN_POINT('Origin',(-3.46627170195,-36.1242356128,2.26279399804));
#49132=CARTESIAN_POINT('',(-3.16691857253,-35.4710616262,2.28248419619));
#49133=CARTESIAN_POINT('',(-3.16691857253,-36.3742356128,2.28248419619));
#49134=CARTESIAN_POINT('',(-3.16691857253,-35.9226486195,2.28248419619));
#49135=CARTESIAN_POINT('',(-3.25430421882,-35.4710616254,2.47509045608));
#49136=CARTESIAN_POINT('Origin',(-3.46627170195,-35.4710616258,2.26279399804));
#49137=CARTESIAN_POINT('',(-3.25430421882,-36.3742356128,2.47509045608));
#49138=CARTESIAN_POINT('',(-3.25430421882,-36.1242356128,2.47509045608));
#49139=CARTESIAN_POINT('Origin',(-3.46627170195,-36.3742356128,2.26279399804));
#49140=CARTESIAN_POINT('Origin',(-1.57756236842E-15,-36.3742356128,4.77612251667E-16));
#49141=CARTESIAN_POINT('',(-14.1514385284,-36.3742356128,6.93238331308));
#49142=CARTESIAN_POINT('',(-14.1514385284,-36.3742356128,-6.93238331308));
#49143=CARTESIAN_POINT('',(-14.1514385284,-36.3742356128,-3.5527136788E-15));
#49144=CARTESIAN_POINT('',(-14.1086187499,-36.3742356128,-7.11244521731));
#49145=CARTESIAN_POINT('Origin',(-13.7514385284,-36.3742356128,-6.93238331308));
#49146=CARTESIAN_POINT('',(-13.1408443824,-36.3742356128,-8.77258279628));
#49147=CARTESIAN_POINT('Origin',(5.52786498918E-15,-36.3742356128,2.25396909107E-15));
#49148=CARTESIAN_POINT('',(-12.8348977878,-36.3742356128,-8.80475037519));
#49149=CARTESIAN_POINT('Origin',(-12.9745045801,-36.3742356128,-8.66153744443));
#49150=CARTESIAN_POINT('',(-11.686904291,-36.3742356128,-7.68566365004));
#49151=CARTESIAN_POINT('',(-0.45986885604,-36.3742356128,3.25867214427));
#49152=CARTESIAN_POINT('',(-11.1212648448,-36.3742356128,-7.69287592692));
#49153=CARTESIAN_POINT('Origin',(-11.4076907064,-36.3742356128,-7.97208951156));
#49154=CARTESIAN_POINT('',(-8.11331856237,-36.3742356128,-10.7785195086));
#49155=CARTESIAN_POINT('',(-8.43647932171,-36.3742356128,-10.447011287));
#49156=CARTESIAN_POINT('',(-8.12053083925,-36.3742356128,-11.3441589548));
#49157=CARTESIAN_POINT('Origin',(-8.39974442389,-36.3742356128,-11.0577330933));
#49158=CARTESIAN_POINT('',(-9.29417531907,-36.3742356128,-12.4882507647));
#49159=CARTESIAN_POINT('',(0.316839226711,-36.3742356128,-3.11924403781));
#49160=CARTESIAN_POINT('',(-9.27193478991,-36.3742356128,-12.7934055377));
#49161=CARTESIAN_POINT('Origin',(-9.15456852675,-36.3742356128,-12.6314636954));
#49162=CARTESIAN_POINT('',(9.27193478991,-36.3742356128,-12.7934055377));
#49163=CARTESIAN_POINT('Origin',(1.97515131038E-15,-36.3742356128,2.25396909107E-15));
#49164=CARTESIAN_POINT('',(9.29417531907,-36.3742356128,-12.4882507647));
#49165=CARTESIAN_POINT('Origin',(9.15456852675,-36.3742356128,-12.6314636954));
#49166=CARTESIAN_POINT('',(8.12053083925,-36.3742356128,-11.3441589548));
#49167=CARTESIAN_POINT('',(-0.316839226711,-36.3742356128,-3.11924403781));
#49168=CARTESIAN_POINT('',(8.11331856237,-36.3742356128,-10.7785195086));
#49169=CARTESIAN_POINT('Origin',(8.39974442389,-36.3742356128,-11.0577330933));
#49170=CARTESIAN_POINT('',(11.1212648448,-36.3742356128,-7.69287592692));
#49171=CARTESIAN_POINT('',(8.43647932171,-36.3742356128,-10.447011287));
#49172=CARTESIAN_POINT('',(11.686904291,-36.3742356128,-7.68566365004));
#49173=CARTESIAN_POINT('Origin',(11.4076907064,-36.3742356128,-7.97208951156));
#49174=CARTESIAN_POINT('',(12.8348977878,-36.3742356128,-8.80475037519));
#49175=CARTESIAN_POINT('',(0.45986885604,-36.3742356128,3.25867214427));
#49176=CARTESIAN_POINT('',(13.1408443824,-36.3742356128,-8.77258279628));
#49177=CARTESIAN_POINT('Origin',(12.9745045801,-36.3742356128,-8.66153744443));
#49178=CARTESIAN_POINT('',(14.1086187499,-36.3742356128,-7.11244521731));
#49179=CARTESIAN_POINT('Origin',(1.98794470979E-16,-36.3742356128,4.77612251667E-16));
#49180=CARTESIAN_POINT('',(14.1514385284,-36.3742356128,-6.93238331308));
#49181=CARTESIAN_POINT('Origin',(13.7514385284,-36.3742356128,-6.93238331308));
#49182=CARTESIAN_POINT('',(14.1514385284,-36.3742356128,6.93238331308));
#49183=CARTESIAN_POINT('',(14.1514385284,-36.3742356128,7.1054273576E-15));
#49184=CARTESIAN_POINT('',(14.1086187499,-36.3742356128,7.11244521731));
#49185=CARTESIAN_POINT('Origin',(13.7514385284,-36.3742356128,6.93238331308));
#49186=CARTESIAN_POINT('',(13.1408443824,-36.3742356128,8.77258279628));
#49187=CARTESIAN_POINT('Origin',(5.04684136861E-13,-36.3742356128,3.05122810209E-13));
#49188=CARTESIAN_POINT('',(12.8348977878,-36.3742356128,8.80475037519));
#49189=CARTESIAN_POINT('Origin',(12.9745045801,-36.3742356128,8.66153744443));
#49190=CARTESIAN_POINT('',(11.686904291,-36.3742356128,7.68566365004));
#49191=CARTESIAN_POINT('',(0.45986885604,-36.3742356128,-3.25867214427));
#49192=CARTESIAN_POINT('',(11.1212648448,-36.3742356128,7.69287592692));
#49193=CARTESIAN_POINT('Origin',(11.4076907064,-36.3742356128,7.97208951156));
#49194=CARTESIAN_POINT('',(8.11331856237,-36.3742356128,10.7785195086));
#49195=CARTESIAN_POINT('',(8.43647932171,-36.3742356128,10.447011287));
#49196=CARTESIAN_POINT('',(8.12053083925,-36.3742356128,11.3441589548));
#49197=CARTESIAN_POINT('Origin',(8.39974442389,-36.3742356128,11.0577330933));
#49198=CARTESIAN_POINT('',(9.29417531907,-36.3742356128,12.4882507647));
#49199=CARTESIAN_POINT('',(-0.316839226711,-36.3742356128,3.11924403781));
#49200=CARTESIAN_POINT('',(9.27193478991,-36.3742356128,12.7934055377));
#49201=CARTESIAN_POINT('Origin',(9.15456852675,-36.3742356128,12.6314636954));
#49202=CARTESIAN_POINT('',(-8.84971102033,-36.3742356128,13.0890265053));
#49203=CARTESIAN_POINT('Origin',(-5.13027604722E-15,-36.3742356128,-1.29874458773E-15));
#49204=CARTESIAN_POINT('',(-8.87729615416,-36.3742356128,12.7801296947));
#49205=CARTESIAN_POINT('Origin',(-8.73768936184,-36.3742356128,12.9233426255));
#49206=CARTESIAN_POINT('',(-7.77151385845,-36.3742356128,11.7021912817));
#49207=CARTESIAN_POINT('',(0.67498798988,-36.3742356128,3.46837452298));
#49208=CARTESIAN_POINT('',(-7.76430158156,-36.3742356128,11.1365518355));
#49209=CARTESIAN_POINT('Origin',(-8.05072744309,-36.3742356128,11.4157654202));
#49210=CARTESIAN_POINT('',(-11.4702818256,-36.3742356128,7.33484360001));
#49211=CARTESIAN_POINT('',(-8.43647932171,-36.3742356128,10.447011287));
#49212=CARTESIAN_POINT('',(-12.0359212718,-36.3742356128,7.32763132313));
#49213=CARTESIAN_POINT('Origin',(-11.7567076872,-36.3742356128,7.61405718465));
#49214=CARTESIAN_POINT('',(-13.1112015384,-36.3742356128,8.37583575597));
#49215=CARTESIAN_POINT('',(-0.818017619209,-36.3742356128,-3.60780262944));
#49216=CARTESIAN_POINT('',(-13.4206904888,-36.3742356128,8.33816927169));
#49217=CARTESIAN_POINT('Origin',(-13.2508083307,-36.3742356128,8.23262282521));
#49218=CARTESIAN_POINT('',(-14.1086187499,-36.3742356128,7.11244521731));
#49219=CARTESIAN_POINT('Origin',(5.79112209092E-12,-36.3742356128,-3.26979532908E-12));
#49220=CARTESIAN_POINT('Origin',(-13.7514385284,-36.3742356128,6.93238331308));
#49221=CARTESIAN_POINT('',(3.51985615629,-36.3742356128,-3.20601908088));
#49222=CARTESIAN_POINT('',(3.67755401867,-36.3742356128,-3.05915055738));
#49223=CARTESIAN_POINT('Origin',(3.78952269078,-36.3742356128,-3.33747234321));
#49224=CARTESIAN_POINT('',(7.07911993306,-36.3742356128,1.41233341424));
#49225=CARTESIAN_POINT('Ctrl Pts',(7.07911993306,-36.3742356128,1.41233341424));
#49226=CARTESIAN_POINT('Ctrl Pts',(7.02062825816,-36.3742356128,0.811131443794));
#49227=CARTESIAN_POINT('Ctrl Pts',(6.765884240706,-36.3742356128,-0.388148698646161));
#49228=CARTESIAN_POINT('Ctrl Pts',(6.23382280728197,-36.3742356128,-1.38868983255432));
#49229=CARTESIAN_POINT('Ctrl Pts',(5.42444395807881,-36.3742356128,-2.19049195793964));
#49230=CARTESIAN_POINT('Ctrl Pts',(4.33774769283,-36.3742356128,-2.79355507478));
#49231=CARTESIAN_POINT('Ctrl Pts',(3.67755401867,-36.3742356128,-3.05915055738));
#49232=CARTESIAN_POINT('',(7.21384189758,-36.3742356128,2.18958432614));
#49233=CARTESIAN_POINT('Ctrl Pts',(7.21384189758,-36.3742356128,2.18958432614));
#49234=CARTESIAN_POINT('Ctrl Pts',(7.13908599018,-36.3742356128,2.05065155888));
#49235=CARTESIAN_POINT('Ctrl Pts',(7.08904524264,-36.3742356128,1.89842024269));
#49236=CARTESIAN_POINT('Ctrl Pts',(7.10533215541,-36.3742356128,1.72680915639));
#49237=CARTESIAN_POINT('Ctrl Pts',(7.09439724612,-36.3742356128,1.56936004643));
#49238=CARTESIAN_POINT('Ctrl Pts',(7.07911993306,-36.3742356128,1.41233341424));
#49239=CARTESIAN_POINT('',(8.75956299023,-36.3742356128,2.0634404101));
#49240=CARTESIAN_POINT('Ctrl Pts',(8.75956299023,-36.3742356128,2.0634404101));
#49241=CARTESIAN_POINT('Ctrl Pts',(8.72637376563,-36.3742356128,2.11781888978));
#49242=CARTESIAN_POINT('Ctrl Pts',(8.6915484,-36.3742356128,2.17268982337));
#49243=CARTESIAN_POINT('Ctrl Pts',(8.65506636668,-36.3742356128,2.22762960985));
#49244=CARTESIAN_POINT('Ctrl Pts',(8.53055023262,-36.3742356128,2.40503324452));
#49245=CARTESIAN_POINT('Ctrl Pts',(8.26494430118178,-36.3742356128,2.70523539119787));
#49246=CARTESIAN_POINT('Ctrl Pts',(7.96786455664539,-36.3742356128,2.8806545502764));
#49247=CARTESIAN_POINT('Ctrl Pts',(7.60100727895793,-36.3742356128,2.68829057805622));
#49248=CARTESIAN_POINT('Ctrl Pts',(7.33749157791351,-36.3742356128,2.40256623079952));
#49249=CARTESIAN_POINT('Ctrl Pts',(7.2297761181,-36.3742356128,2.21919784335));
#49250=CARTESIAN_POINT('Ctrl Pts',(7.21384189758,-36.3742356128,2.18958432614));
#49251=CARTESIAN_POINT('',(9.23698117862,-36.3742356128,0.509886547139));
#49252=CARTESIAN_POINT('Ctrl Pts',(8.75956299023,-36.3742356128,2.0634404101));
#49253=CARTESIAN_POINT('Ctrl Pts',(8.92890465395,-36.3742356128,1.78598462948));
#49254=CARTESIAN_POINT('Ctrl Pts',(9.07291332076,-36.3742356128,1.49306717121));
#49255=CARTESIAN_POINT('Ctrl Pts',(9.12674872803,-36.3742356128,1.15064845916));
#49256=CARTESIAN_POINT('Ctrl Pts',(9.18664865847,-36.3742356128,0.831017278590001));
#49257=CARTESIAN_POINT('Ctrl Pts',(9.23698117862,-36.3742356128,0.509886547135));
#49258=CARTESIAN_POINT('',(1.87043161103,-36.3742356128,-8.24476960824));
#49259=CARTESIAN_POINT('Ctrl Pts',(1.87043161103,-36.3742356128,-8.24476960824));
#49260=CARTESIAN_POINT('Ctrl Pts',(2.47265813357,-36.3742356128,-8.13634296351));
#49261=CARTESIAN_POINT('Ctrl Pts',(3.05192283465,-36.3742356128,-7.98771609515));
#49262=CARTESIAN_POINT('Ctrl Pts',(4.33873711989964,-36.3742356128,-7.55106216307255));
#49263=CARTESIAN_POINT('Ctrl Pts',(5.96679547826005,-36.3742356128,-6.64390177065611));
#49264=CARTESIAN_POINT('Ctrl Pts',(7.82299194608668,-36.3742356128,-5.03608217876813));
#49265=CARTESIAN_POINT('Ctrl Pts',(9.32974836502124,-36.3742356128,-3.47204744400302));
#49266=CARTESIAN_POINT('Ctrl Pts',(9.44907784606298,-36.3742356128,-1.45170212295927));
#49267=CARTESIAN_POINT('Ctrl Pts',(9.34900416387435,-36.3742356128,-0.255886314382252));
#49268=CARTESIAN_POINT('Ctrl Pts',(9.25795835827,-36.3742356128,0.376048284641));
#49269=CARTESIAN_POINT('Ctrl Pts',(9.23698117862,-36.3742356128,0.509886547139));
#49270=CARTESIAN_POINT('',(1.51727342606,-36.3742356128,-7.9495168227));
#49271=CARTESIAN_POINT('Origin',(1.81727342606,-36.3742356128,-7.9495168227));
#49272=CARTESIAN_POINT('',(1.51727342606,-36.3742356128,-5.3088808072));
#49273=CARTESIAN_POINT('',(1.51727342606,-36.3742356128,-6.62919881495));
#49274=CARTESIAN_POINT('',(1.68475792039,-36.3742356128,-5.03973467448));
#49275=CARTESIAN_POINT('Origin',(1.81727342606,-36.3742356128,-5.3088808072));
#49276=CARTESIAN_POINT('Ctrl Pts',(3.51985615629,-36.3742356128,-3.20601908088));
#49277=CARTESIAN_POINT('Ctrl Pts',(3.41903503516,-36.3742356128,-3.4128460691));
#49278=CARTESIAN_POINT('Ctrl Pts',(3.30675917974,-36.3742356128,-3.60871163219));
#49279=CARTESIAN_POINT('Ctrl Pts',(3.01387620630693,-36.3742356128,-4.04639865742235));
#49280=CARTESIAN_POINT('Ctrl Pts',(2.65681036718069,-36.3742356128,-4.42266691385755));
#49281=CARTESIAN_POINT('Ctrl Pts',(2.23556166242,-36.3742356128,-4.73751640159));
#49282=CARTESIAN_POINT('Ctrl Pts',(1.97086406258,-36.3742356128,-4.89886881947));
#49283=CARTESIAN_POINT('Ctrl Pts',(1.68475792039,-36.3742356128,-5.03973467448));
#49284=CARTESIAN_POINT('',(3.0462613877,-36.3742356128,0.448114344193));
#49285=CARTESIAN_POINT('',(2.97642257165,-36.3742356128,0.274612461872));
#49286=CARTESIAN_POINT('Origin',(2.74690825827,-36.3742356128,0.467804542343));
#49287=CARTESIAN_POINT('',(-2.97642257165,-36.3742356128,0.274612461872));
#49288=CARTESIAN_POINT('Origin',(-1.14807003446E-14,-36.3742356128,2.77999550541));
#49289=CARTESIAN_POINT('',(-3.0462613877,-36.3742356128,0.448114344193));
#49290=CARTESIAN_POINT('Origin',(-2.74690825827,-36.3742356128,0.467804542343));
#49291=CARTESIAN_POINT('',(-3.10658998011,-36.3742356128,1.36529927019));
#49292=CARTESIAN_POINT('',(8.77076189454E-15,-36.3742356128,9.2896999221));
#49293=CARTESIAN_POINT('Origin',(-0.425321894002,-36.3742356128,5.30846337982));
#49294=CARTESIAN_POINT('',(3.25430421882,-36.3742356128,2.47509045608));
#49295=CARTESIAN_POINT('Origin',(0.425321894002,-36.3742356128,5.30846337982));
#49296=CARTESIAN_POINT('',(3.16691857253,-36.3742356128,2.28248419619));
#49297=CARTESIAN_POINT('Origin',(3.46627170195,-36.3742356128,2.26279399804));
#49298=CARTESIAN_POINT('',(3.10658998011,-36.3742356128,1.36529927019));
#49299=CARTESIAN_POINT('',(-1.51727342606,-36.3742356128,-5.3088808072));
#49300=CARTESIAN_POINT('',(-1.51727342606,-36.3742356128,-7.9495168227));
#49301=CARTESIAN_POINT('',(-1.51727342606,-36.3742356128,-6.62919881495));
#49302=CARTESIAN_POINT('',(-1.87043161103,-36.3742356128,-8.24476960824));
#49303=CARTESIAN_POINT('Origin',(-1.81727342606,-36.3742356128,-7.9495168227));
#49304=CARTESIAN_POINT('',(-9.23698117862,-36.3742356128,0.509886547139));
#49305=CARTESIAN_POINT('Ctrl Pts',(-1.87043161103,-36.3742356128,-8.24476960824));
#49306=CARTESIAN_POINT('Ctrl Pts',(-2.47265813357,-36.3742356128,-8.13634296351));
#49307=CARTESIAN_POINT('Ctrl Pts',(-3.05192283465,-36.3742356128,-7.98771609515));
#49308=CARTESIAN_POINT('Ctrl Pts',(-3.608285111,-36.3742356128,-7.79892601222));
#49309=CARTESIAN_POINT('Ctrl Pts',(-4.84313848674,-36.3742356128,-7.27000777732));
#49310=CARTESIAN_POINT('Ctrl Pts',(-5.97499470659,-36.3742356128,-6.53839758248));
#49311=CARTESIAN_POINT('Ctrl Pts',(-6.59156749188,-36.3742356128,-6.06232184959));
#49312=CARTESIAN_POINT('Ctrl Pts',(-7.62010012329,-36.3742356128,-5.1678005996));
#49313=CARTESIAN_POINT('Ctrl Pts',(-8.47746400168,-36.3742356128,-4.11735171219));
#49314=CARTESIAN_POINT('Ctrl Pts',(-8.78407978672,-36.3742356128,-3.65866522624));
#49315=CARTESIAN_POINT('Ctrl Pts',(-9.22504359392,-36.3742356128,-2.71647636201));
#49316=CARTESIAN_POINT('Ctrl Pts',(-9.38605456704,-36.3742356128,-1.68617604095));
#49317=CARTESIAN_POINT('Ctrl Pts',(-9.40005841918,-36.3742356128,-1.17735235373));
#49318=CARTESIAN_POINT('Ctrl Pts',(-9.36972184244,-36.3742356128,-0.530817230024));
#49319=CARTESIAN_POINT('Ctrl Pts',(-9.2950327654,-36.3742356128,0.106470788818));
#49320=CARTESIAN_POINT('Ctrl Pts',(-9.27733443288,-36.3742356128,0.241562002067001));
#49321=CARTESIAN_POINT('Ctrl Pts',(-9.25795835827,-36.3742356128,0.376048284641));
#49322=CARTESIAN_POINT('Ctrl Pts',(-9.23698117862397,-36.3742356128,0.509886547139624));
#49323=CARTESIAN_POINT('',(-8.75956299023,-36.3742356128,2.0634404101));
#49324=CARTESIAN_POINT('Ctrl Pts',(-8.75956299023,-36.3742356128,2.0634404101));
#49325=CARTESIAN_POINT('Ctrl Pts',(-8.92890465395,-36.3742356128,1.78598462948));
#49326=CARTESIAN_POINT('Ctrl Pts',(-9.07291332076,-36.3742356128,1.49306717121));
#49327=CARTESIAN_POINT('Ctrl Pts',(-9.12674872803,-36.3742356128,1.15064845916));
#49328=CARTESIAN_POINT('Ctrl Pts',(-9.18664865847,-36.3742356128,0.831017278590001));
#49329=CARTESIAN_POINT('Ctrl Pts',(-9.23698117862,-36.3742356128,0.509886547135));
#49330=CARTESIAN_POINT('',(-7.21384189759,-36.3742356128,2.18958432614));
#49331=CARTESIAN_POINT('Ctrl Pts',(-8.75956299024,-36.3742356128,2.0634404101));
#49332=CARTESIAN_POINT('Ctrl Pts',(-8.72637376563,-36.3742356128,2.11781888978));
#49333=CARTESIAN_POINT('Ctrl Pts',(-8.6915484,-36.3742356128,2.17268982337));
#49334=CARTESIAN_POINT('Ctrl Pts',(-8.65506636668,-36.3742356128,2.22762960985));
#49335=CARTESIAN_POINT('Ctrl Pts',(-8.53055023262,-36.3742356128,2.40503324452));
#49336=CARTESIAN_POINT('Ctrl Pts',(-8.3876008666,-36.3742356128,2.56660232663));
#49337=CARTESIAN_POINT('Ctrl Pts',(-8.27908544119,-36.3742356128,2.66027026629));
#49338=CARTESIAN_POINT('Ctrl Pts',(-8.01327762974,-36.3742356128,2.78696551824));
#49339=CARTESIAN_POINT('Ctrl Pts',(-7.71906576509,-36.3742356128,2.71717075777));
#49340=CARTESIAN_POINT('Ctrl Pts',(-7.55641153588,-36.3742356128,2.61428156978));
#49341=CARTESIAN_POINT('Ctrl Pts',(-7.38865661676,-36.3742356128,2.45617777771));
#49342=CARTESIAN_POINT('Ctrl Pts',(-7.26550535688,-36.3742356128,2.27753774962));
#49343=CARTESIAN_POINT('Ctrl Pts',(-7.24701042964,-36.3742356128,2.24853650952));
#49344=CARTESIAN_POINT('Ctrl Pts',(-7.2297761181,-36.3742356128,2.21919784335));
#49345=CARTESIAN_POINT('Ctrl Pts',(-7.21384189758642,-36.3742356128,2.18958432614193));
#49346=CARTESIAN_POINT('',(-7.07911993306,-36.3742356128,1.41233341424));
#49347=CARTESIAN_POINT('Ctrl Pts',(-7.21384189759,-36.3742356128,2.18958432614));
#49348=CARTESIAN_POINT('Ctrl Pts',(-7.13908599018,-36.3742356128,2.05065155888));
#49349=CARTESIAN_POINT('Ctrl Pts',(-7.08904524264,-36.3742356128,1.89842024269));
#49350=CARTESIAN_POINT('Ctrl Pts',(-7.10533215541,-36.3742356128,1.72680915639));
#49351=CARTESIAN_POINT('Ctrl Pts',(-7.09439724612,-36.3742356128,1.56936004643));
#49352=CARTESIAN_POINT('Ctrl Pts',(-7.07911993306,-36.3742356128,1.41233341424));
#49353=CARTESIAN_POINT('',(-3.67755401867,-36.3742356128,-3.05915055738));
#49354=CARTESIAN_POINT('Ctrl Pts',(-7.07911993306,-36.3742356128,1.41233341424));
#49355=CARTESIAN_POINT('Ctrl Pts',(-6.86965601460853,-36.3742356128,-0.740624604739125));
#49356=CARTESIAN_POINT('Ctrl Pts',(-5.73580070981187,-36.3742356128,-2.23111926194579));
#49357=CARTESIAN_POINT('Ctrl Pts',(-3.67755401867,-36.3742356128,-3.05915055738));
#49358=CARTESIAN_POINT('',(-3.51985615629,-36.3742356128,-3.20601908088));
#49359=CARTESIAN_POINT('Origin',(-3.78952269078,-36.3742356128,-3.33747234321));
#49360=CARTESIAN_POINT('',(-1.68475792039,-36.3742356128,-5.03973467448));
#49361=CARTESIAN_POINT('Ctrl Pts',(-3.51985615629,-36.3742356128,-3.20601908088));
#49362=CARTESIAN_POINT('Ctrl Pts',(-3.12209962985425,-36.3742356128,-4.0219868412465));
#49363=CARTESIAN_POINT('Ctrl Pts',(-2.51040021788758,-36.3742356128,-4.6332253724465));
#49364=CARTESIAN_POINT('Ctrl Pts',(-1.68475792039,-36.3742356128,-5.03973467448));
#49365=CARTESIAN_POINT('Origin',(-1.81727342606,-36.3742356128,-5.3088808072));
#49366=CARTESIAN_POINT('Ctrl Pts',(-9.23698117862,-35.3742356128,0.509886547138));
#49367=CARTESIAN_POINT('Ctrl Pts',(-9.85462053301,-32.4742356128,2.00920484002));
#49368=CARTESIAN_POINT('Ctrl Pts',(-9.29448486778,-35.3742356128,0.14300248283));
#49369=CARTESIAN_POINT('Ctrl Pts',(-9.89942675021,-32.4742356128,1.54440936128));
#49370=CARTESIAN_POINT('Ctrl Pts',(-9.33952412131,-35.3742356128,-0.225988266205));
#49371=CARTESIAN_POINT('Ctrl Pts',(-9.93347655148,-32.4742356128,1.07876884298));
#49372=CARTESIAN_POINT('Ctrl Pts',(-9.37147906182,-35.3742356128,-0.598052135313));
#49373=CARTESIAN_POINT('Ctrl Pts',(-9.95684539874,-32.4742356128,0.6105872463));
#49374=CARTESIAN_POINT('Ctrl Pts',(-9.39776085185,-35.3742356128,-1.34354990637));
#49375=CARTESIAN_POINT('Ctrl Pts',(-9.98182966629,-32.4742356128,-0.323612218818));
#49376=CARTESIAN_POINT('Ctrl Pts',(-9.31944120585,-35.3742356128,-2.08553948714));
#49377=CARTESIAN_POINT('Ctrl Pts',(-9.96363436978,-32.4742356128,-1.25779968708));
#49378=CARTESIAN_POINT('Ctrl Pts',(-9.24709061054,-35.3742356128,-2.45151005123));
#49379=CARTESIAN_POINT('Ctrl Pts',(-9.943864011,-32.4742356128,-1.72215443881));
#49380=CARTESIAN_POINT('Ctrl Pts',(-9.13406983882,-35.3742356128,-2.80846571914));
#49381=CARTESIAN_POINT('Ctrl Pts',(-9.91319925962,-32.4742356128,-2.18875096266));
#49382=CARTESIAN_POINT('Ctrl Pts',(-8.98669828191,-35.3742356128,-3.15062625521));
#49383=CARTESIAN_POINT('Ctrl Pts',(-9.87176476169,-32.4742356128,-2.65438916225));
#49384=CARTESIAN_POINT('',(-9.01911881647387,-35.2680071588898,-3.13244858247421));
#49385=CARTESIAN_POINT('',(-9.87176476169,-32.4742356128,-2.65438916225));
#49386=CARTESIAN_POINT('',(-9.01911869317,-35.2680072167,-3.13244885159));
#49387=CARTESIAN_POINT('',(-9.85462053301,-32.4742356128,2.00920484002));
#49388=CARTESIAN_POINT('Ctrl Pts',(-9.87176476169,-32.4742356128,-2.65438916225));
#49389=CARTESIAN_POINT('Ctrl Pts',(-9.91319925961983,-32.4742356128006,
-2.18875096266014));
#49390=CARTESIAN_POINT('Ctrl Pts',(-9.94386401099985,-32.4742356128006,
-1.72215443881016));
#49391=CARTESIAN_POINT('Ctrl Pts',(-9.96363436977986,-32.4742356128006,
-1.25779968708018));
#49392=CARTESIAN_POINT('Ctrl Pts',(-9.98182966628987,-32.4742356128006,
-0.323612218818225));
#49393=CARTESIAN_POINT('Ctrl Pts',(-9.95684539873987,-32.4742356128006,
0.610587246299733));
#49394=CARTESIAN_POINT('Ctrl Pts',(-9.93347655147987,-32.4742356128006,
1.07876884297971));
#49395=CARTESIAN_POINT('Ctrl Pts',(-9.89942675020987,-32.4742356128006,
1.54440936127969));
#49396=CARTESIAN_POINT('Ctrl Pts',(-9.85462053301,-32.4742356128,2.00920484002));
#49397=CARTESIAN_POINT('',(-9.26569106343796,-35.2394341085959,0.579579885999344));
#49398=CARTESIAN_POINT('',(-9.26569107792,-35.2394341184,0.579579770069));
#49399=CARTESIAN_POINT('',(-9.27386188271847,-35.2408046524422,0.522899877211487));
#49400=CARTESIAN_POINT('Ctrl Pts',(-9.27386188241726,-35.2408046523711,
0.522899878102206));
#49401=CARTESIAN_POINT('Ctrl Pts',(-9.272854956216,-35.2406369805721,0.529976427463772));
#49402=CARTESIAN_POINT('Ctrl Pts',(-9.27184238659432,-35.240469340988,0.537055008970363));
#49403=CARTESIAN_POINT('Ctrl Pts',(-9.27082740815912,-35.2403006245684,
0.544116409517216));
#49404=CARTESIAN_POINT('Ctrl Pts',(-9.26952133291424,-35.2400835201144,
0.553203026659481));
#49405=CARTESIAN_POINT('Ctrl Pts',(-9.26821080810748,-35.2398633916849,
0.562266670796889));
#49406=CARTESIAN_POINT('Ctrl Pts',(-9.26689225647901,-35.2396388881584,
0.571334399836343));
#49407=CARTESIAN_POINT('Ctrl Pts',(-9.26649252516074,-35.2395708278044,
0.574083367115571));
#49408=CARTESIAN_POINT('Ctrl Pts',(-9.26609219211384,-35.2395024442855,
0.576831669736027));
#49409=CARTESIAN_POINT('Ctrl Pts',(-9.26569107942698,-35.2394341188372,
0.579579770121116));
#49410=CARTESIAN_POINT('Ctrl Pts',(-9.01911901239593,-35.2680072483449,
-3.13244806238356));
#49411=CARTESIAN_POINT('Ctrl Pts',(-9.04725342339902,-35.2707959773529,
-3.06289434530028));
#49412=CARTESIAN_POINT('Ctrl Pts',(-9.0738646799152,-35.2732630041589,-2.99276671560158));
#49413=CARTESIAN_POINT('Ctrl Pts',(-9.09886532753374,-35.2754096171468,
-2.9220854676137));
#49414=CARTESIAN_POINT('Ctrl Pts',(-9.12517964497291,-35.2776690248407,
-2.84769024294082));
#49415=CARTESIAN_POINT('Ctrl Pts',(-9.14970966431518,-35.2795734922357,
-2.77268175024793));
#49416=CARTESIAN_POINT('Ctrl Pts',(-9.17240841720282,-35.2811368888824,
-2.69710071226188));
#49417=CARTESIAN_POINT('Ctrl Pts',(-9.19600438692266,-35.2827620821306,
-2.61853217184287));
#49418=CARTESIAN_POINT('Ctrl Pts',(-9.21762169379382,-35.2840187974798,
-2.5393450744354));
#49419=CARTESIAN_POINT('Ctrl Pts',(-9.23726341419725,-35.2849346746476,
-2.45960149213306));
#49420=CARTESIAN_POINT('Ctrl Pts',(-9.25786492376434,-35.2858953059899,
-2.37596125390682));
#49421=CARTESIAN_POINT('Ctrl Pts',(-9.27629335665372,-35.2864810937416,
-2.29170901187452));
#49422=CARTESIAN_POINT('Ctrl Pts',(-9.29260846387214,-35.2867353478736,
-2.2069313808944));
#49423=CARTESIAN_POINT('Ctrl Pts',(-9.31079942565656,-35.2870188352658,
-2.11240631129561));
#49424=CARTESIAN_POINT('Ctrl Pts',(-9.32636317658767,-35.2868902870952,
-2.01722832593922));
#49425=CARTESIAN_POINT('Ctrl Pts',(-9.33944913890977,-35.2864218830791,
-1.92153248339109));
#49426=CARTESIAN_POINT('Ctrl Pts',(-9.35381931851821,-35.2859075112908,
-1.81644533646613));
#49427=CARTESIAN_POINT('Ctrl Pts',(-9.36520238713606,-35.2849836925435,
-1.71073435590058));
#49428=CARTESIAN_POINT('Ctrl Pts',(-9.37386541799886,-35.2837558348772,
-1.60458838444502));
#49429=CARTESIAN_POINT('Ctrl Pts',(-9.38474687491737,-35.2822135478291,
-1.47126058800049));
#49430=CARTESIAN_POINT('Ctrl Pts',(-9.39133885899346,-35.2801929029209,
-1.3372488789615));
#49431=CARTESIAN_POINT('Ctrl Pts',(-9.39425596414206,-35.2779042511112,
-1.20291850223005));
#49432=CARTESIAN_POINT('Ctrl Pts',(-9.39511004211027,-35.2772341734184,
-1.16358888969212));
#49433=CARTESIAN_POINT('Ctrl Pts',(-9.39564939677077,-35.2765410404658,
-1.12423175686172));
#49434=CARTESIAN_POINT('Ctrl Pts',(-9.39588979120016,-35.2758298198528,
-1.08485559963608));
#49435=CARTESIAN_POINT('Ctrl Pts',(-9.396596184031,-35.2737399164243,-0.969149777163249));
#49436=CARTESIAN_POINT('Ctrl Pts',(-9.39472508784569,-35.2714936022906,
-0.853280252617673));
#49437=CARTESIAN_POINT('Ctrl Pts',(-9.39066660958969,-35.2691363044524,
-0.737398533363237));
#49438=CARTESIAN_POINT('Ctrl Pts',(-9.38695087508032,-35.2669780834706,
-0.631303175429051));
#49439=CARTESIAN_POINT('Ctrl Pts',(-9.38140163564093,-35.2647271155357,
-0.525197961588922));
#49440=CARTESIAN_POINT('Ctrl Pts',(-9.37427716929374,-35.2624161741734,
-0.41918685381147));
#49441=CARTESIAN_POINT('Ctrl Pts',(-9.36741419186441,-35.2601900511717,
-0.317066666210076));
#49442=CARTESIAN_POINT('Ctrl Pts',(-9.3590897311375,-35.2579084833464,-0.215034122490352));
#49443=CARTESIAN_POINT('Ctrl Pts',(-9.34949252196957,-35.2555953326665,
-0.113165335408674));
#49444=CARTESIAN_POINT('Ctrl Pts',(-9.34019666058181,-35.2533548138122,
-0.0144951795455671));
#49445=CARTESIAN_POINT('Ctrl Pts',(-9.32970691361629,-35.2510848261654,
0.0840210909909912));
#49446=CARTESIAN_POINT('Ctrl Pts',(-9.31815142540981,-35.2487992164153,
0.182334480492819));
#49447=CARTESIAN_POINT('Ctrl Pts',(-9.30702365779603,-35.2465982073623,
0.277008849255942));
#49448=CARTESIAN_POINT('Ctrl Pts',(-9.29490766568224,-35.2443828222107,
0.371494917639165));
#49449=CARTESIAN_POINT('Ctrl Pts',(-9.28187516958525,-35.2421561121088,
0.465770832179655));
#49450=CARTESIAN_POINT('Ctrl Pts',(-9.27924152669378,-35.2417061323668,
0.484822369990843));
#49451=CARTESIAN_POINT('Ctrl Pts',(-9.27657030962703,-35.2412556556506,
0.503865404015155));
#49452=CARTESIAN_POINT('Ctrl Pts',(-9.27386188313803,-35.2408046525553,
0.522899876806236));
#49453=CARTESIAN_POINT('Origin',(-3.46627170195,-35.4710616254,2.26279399804));
#49454=CARTESIAN_POINT('',(-3.24268782378383,-35.295907687595,2.35939289985189));
#49455=CARTESIAN_POINT('Origin',(-3.46628339291417,-35.4710655417899,2.26279140790743));
#49456=CARTESIAN_POINT('Origin',(-3.46628278031483,-35.4710655875802,2.26278688734025));
#49457=CARTESIAN_POINT('Origin',(12.7514385284,-32.4742356128,7.05028367309));
#49458=CARTESIAN_POINT('',(12.7514385284,-32.4742356128,6.7682619245));
#49459=CARTESIAN_POINT('',(12.7514385284,-32.4742356128,-6.7682619245));
#49460=CARTESIAN_POINT('',(12.7514385284,-32.4742356128,3.5527136788E-15));
#49461=CARTESIAN_POINT('',(12.7514385284,-32.8742356128,-6.7682619245));
#49462=CARTESIAN_POINT('',(12.7514385284,-33.6742356128,-6.7682619245));
#49463=CARTESIAN_POINT('',(12.7514385284,-32.8742356128,6.7682619245));
#49464=CARTESIAN_POINT('',(12.7514385284,-32.8742356128,5.3290705182E-15));
#49465=CARTESIAN_POINT('',(12.7514385284,-33.6742356128,6.7682619245));
#49466=CARTESIAN_POINT('Ctrl Pts',(3.51985615629,-36.3742356128,-3.20601908088));
#49467=CARTESIAN_POINT('Ctrl Pts',(3.51985615629,-35.2912304609806,-3.20601908088));
#49468=CARTESIAN_POINT('Ctrl Pts',(3.41903503516,-36.3742356128,-3.4128460691));
#49469=CARTESIAN_POINT('Ctrl Pts',(3.41903503516,-35.2912304609806,-3.4128460691));
#49470=CARTESIAN_POINT('Ctrl Pts',(3.30675917974,-36.3742356128,-3.60871163219));
#49471=CARTESIAN_POINT('Ctrl Pts',(3.30675917974,-35.2912304609806,-3.60871163219));
#49472=CARTESIAN_POINT('Ctrl Pts',(3.18302859005,-36.3742356128,-3.79361577017));
#49473=CARTESIAN_POINT('Ctrl Pts',(3.18302859005,-35.2912304609806,-3.79361577017));
#49474=CARTESIAN_POINT('Ctrl Pts',(2.86303108781,-36.3742356128,-4.20535597988));
#49475=CARTESIAN_POINT('Ctrl Pts',(2.86303108781,-35.2912304609806,-4.20535597988));
#49476=CARTESIAN_POINT('Ctrl Pts',(2.47885071991,-36.3742356128,-4.55567742084));
#49477=CARTESIAN_POINT('Ctrl Pts',(2.47885071991,-35.2912304609806,-4.55567742084));
#49478=CARTESIAN_POINT('Ctrl Pts',(2.23556166242,-36.3742356128,-4.73751640159));
#49479=CARTESIAN_POINT('Ctrl Pts',(2.23556166242,-35.2912304609806,-4.73751640159));
#49480=CARTESIAN_POINT('Ctrl Pts',(1.97086406258,-36.3742356128,-4.89886881947));
#49481=CARTESIAN_POINT('Ctrl Pts',(1.97086406258,-35.2912304609806,-4.89886881947));
#49482=CARTESIAN_POINT('Ctrl Pts',(1.68475792038,-36.3742356128,-5.03973467448));
#49483=CARTESIAN_POINT('Ctrl Pts',(1.68475792038,-35.2912304609806,-5.03973467448));
#49484=CARTESIAN_POINT('',(1.68475791952077,-35.4771141863372,-5.03973467240991));
#49485=CARTESIAN_POINT('',(1.68475792039,-36.1242356128,-5.03973467448));
#49486=CARTESIAN_POINT('',(3.51985615455486,-35.4822398766,-3.20601908003418));
#49487=CARTESIAN_POINT('Ctrl Pts',(3.51985615629,-35.4822398766,-3.20601908088));
#49488=CARTESIAN_POINT('Ctrl Pts',(3.48180288665517,-35.4888161519969,-3.28408251701604));
#49489=CARTESIAN_POINT('Ctrl Pts',(3.44134140954082,-35.4947135960524,-3.36118600277347));
#49490=CARTESIAN_POINT('Ctrl Pts',(3.39844886475906,-35.4999359868531,-3.4370172166045));
#49491=CARTESIAN_POINT('Ctrl Pts',(3.35616498680118,-35.5050842692967,-3.51177234730016));
#49492=CARTESIAN_POINT('Ctrl Pts',(3.31151851954779,-35.5095765212415,-3.58529103121342));
#49493=CARTESIAN_POINT('Ctrl Pts',(3.26452422693521,-35.5134163622067,-3.65730914068904));
#49494=CARTESIAN_POINT('Ctrl Pts',(3.21779936995671,-35.5172341879456,-3.72891434374746));
#49495=CARTESIAN_POINT('Ctrl Pts',(3.16875348688733,-35.5204070622853,-3.79903608623969));
#49496=CARTESIAN_POINT('Ctrl Pts',(3.11743821539015,-35.5229385428452,-3.86745028487632));
#49497=CARTESIAN_POINT('Ctrl Pts',(3.06637753705852,-35.525457463837,-3.93552505653747));
#49498=CARTESIAN_POINT('Ctrl Pts',(3.01306991419488,-35.5273413396226,-4.00190916785641));
#49499=CARTESIAN_POINT('Ctrl Pts',(2.95760356691231,-35.528593675132,-4.06641759311961));
#49500=CARTESIAN_POINT('Ctrl Pts',(2.93904343249216,-35.5290127313081,-4.08800338527602));
#49501=CARTESIAN_POINT('Ctrl Pts',(2.92024189659838,-35.5293610736877,-4.10937945444489));
#49502=CARTESIAN_POINT('Ctrl Pts',(2.90120320780892,-35.5296388335917,-4.13053977074822));
#49503=CARTESIAN_POINT('Ctrl Pts',(2.84438099451083,-35.5304678262125,-4.19369412028033));
#49504=CARTESIAN_POINT('Ctrl Pts',(2.78544352061609,-35.5306680961798,-4.25492395294756));
#49505=CARTESIAN_POINT('Ctrl Pts',(2.72452890068556,-35.5302431347145,-4.31409304263514));
#49506=CARTESIAN_POINT('Ctrl Pts',(2.66349205332807,-35.5298173205484,-4.373380857279));
#49507=CARTESIAN_POINT('Ctrl Pts',(2.60047012309514,-35.5287637633326,-4.43059965604713));
#49508=CARTESIAN_POINT('Ctrl Pts',(2.53563992629681,-35.5270859753459,-4.48564862898242));
#49509=CARTESIAN_POINT('Ctrl Pts',(2.47028724896019,-35.525394665704,-4.54114125346331));
#49510=CARTESIAN_POINT('Ctrl Pts',(2.40309703862138,-35.523069023126,-4.59442893453327));
#49511=CARTESIAN_POINT('Ctrl Pts',(2.33428890096677,-35.5201126454955,-4.64544522784908));
#49512=CARTESIAN_POINT('Ctrl Pts',(2.26501486437094,-35.5171362502732,-4.69680695177601));
#49513=CARTESIAN_POINT('Ctrl Pts',(2.19410095479911,-35.5135205496852,-4.74586646153125));
#49514=CARTESIAN_POINT('Ctrl Pts',(2.12180983582931,-35.5092692151946,-4.79259285979375));
#49515=CARTESIAN_POINT('Ctrl Pts',(2.04834448774971,-35.5049488260153,-4.84007823782884));
#49516=CARTESIAN_POINT('Ctrl Pts',(1.97345684281429,-35.4999719859482,-4.88515411046425));
#49517=CARTESIAN_POINT('Ctrl Pts',(1.89746194913474,-35.4943425482858,-4.92782573054381));
#49518=CARTESIAN_POINT('Ctrl Pts',(1.82740924757862,-35.4891532875684,-4.9671607716448));
#49519=CARTESIAN_POINT('Ctrl Pts',(1.75641620304805,-35.483409495094,-5.00445334434491));
#49520=CARTESIAN_POINT('Ctrl Pts',(1.68475792038805,-35.4771141891,-5.03973467447604));
#49521=CARTESIAN_POINT('',(3.51985615629,-36.1242356128,-3.20601908088));
#49522=CARTESIAN_POINT('Origin',(1.81727342606,-36.1242356128,-5.3088808072));
#49523=CARTESIAN_POINT('',(1.51727374257837,-35.5445459414522,-5.30854202326636));
#49524=CARTESIAN_POINT('',(1.51727342606,-35.9593880834,-5.3088808072));
#49525=CARTESIAN_POINT('',(1.67696448374633,-35.4768981244436,-5.04371406601353));
#49526=CARTESIAN_POINT('Ctrl Pts',(1.67696448325,-35.4768981249,-5.04371406613));
#49527=CARTESIAN_POINT('Ctrl Pts',(1.64455688984,-35.4917317677,-5.06086202998));
#49528=CARTESIAN_POINT('Ctrl Pts',(1.61513825447,-35.505058041,-5.08277314744));
#49529=CARTESIAN_POINT('Ctrl Pts',(1.58873141496,-35.5179848719,-5.10914094848));
#49530=CARTESIAN_POINT('Ctrl Pts',(1.54998925981,-35.5347051565,-5.16293840519));
#49531=CARTESIAN_POINT('Ctrl Pts',(1.52721834654,-35.5426195859,-5.22486268019));
#49532=CARTESIAN_POINT('Ctrl Pts',(1.52071813077,-35.5443146003,-5.25227472437));
#49533=CARTESIAN_POINT('Ctrl Pts',(1.51732687674,-35.5452006575,-5.27999548691));
#49534=CARTESIAN_POINT('Ctrl Pts',(1.51727394979,-35.5445470238,-5.30832023528));
#49535=CARTESIAN_POINT('Origin',(1.6862492552706,-35.5734099629681,-5.04271729832598));
#49536=CARTESIAN_POINT('Origin',(1.51727342606,-32.4742356128,-5.11808633804));
#49537=CARTESIAN_POINT('',(1.51727342288,-35.544540501139,-7.94951682269995));
#49538=CARTESIAN_POINT('',(1.51727342606,-36.1242356128,-7.9495168227));
#49539=CARTESIAN_POINT('',(1.51727342606,-35.544540554,-5.3083202352798));
#49540=CARTESIAN_POINT('Origin',(1.81727342606,-36.1242356128,-7.9495168227));
#49541=CARTESIAN_POINT('',(1.8704316154347,-35.4944687624331,-8.24476961257036));
#49542=CARTESIAN_POINT('',(1.87043161103,-36.1242356128,-8.24476960824));
#49543=CARTESIAN_POINT('',(1.85568221013649,-35.4970690565643,-8.24704793966574));
#49544=CARTESIAN_POINT('Origin',(1.86844266437558,-35.7037699017498,-8.22958286354931));
#49545=CARTESIAN_POINT('',(1.51739959473689,-35.5460990323408,-7.95821664298045));
#49546=CARTESIAN_POINT('Ctrl Pts',(1.51739959739202,-35.5460990330595,-7.95821664354419));
#49547=CARTESIAN_POINT('Ctrl Pts',(1.51784040157713,-35.551544433581,-7.9734107080064));
#49548=CARTESIAN_POINT('Ctrl Pts',(1.51944015474546,-35.5564624662645,-7.98865298821528));
#49549=CARTESIAN_POINT('Ctrl Pts',(1.52221396870495,-35.5607753418337,-8.00374326615405));
#49550=CARTESIAN_POINT('Ctrl Pts',(1.52508034792987,-35.5652321428706,-8.01933712349758));
#49551=CARTESIAN_POINT('Ctrl Pts',(1.52920035542674,-35.5690427768125,-8.03476806671595));
#49552=CARTESIAN_POINT('Ctrl Pts',(1.53454083399218,-35.5721488750417,-8.04981508926192));
#49553=CARTESIAN_POINT('Ctrl Pts',(1.53985832132163,-35.5752416012412,-8.06479733303534));
#49554=CARTESIAN_POINT('Ctrl Pts',(1.54638538066407,-35.577636071276,-8.07939834280623));
#49555=CARTESIAN_POINT('Ctrl Pts',(1.55404503872652,-35.579299076886,-8.09340906153831));
#49556=CARTESIAN_POINT('Ctrl Pts',(1.56199623962116,-35.5810253800168,-8.10795305794244));
#49557=CARTESIAN_POINT('Ctrl Pts',(1.57116678649342,-35.581963465072,-8.12185869749068));
#49558=CARTESIAN_POINT('Ctrl Pts',(1.58142798632441,-35.5821006264457,-8.13491533384685));
#49559=CARTESIAN_POINT('Ctrl Pts',(1.59149584448517,-35.5822352034228,-8.14772595687882));
#49560=CARTESIAN_POINT('Ctrl Pts',(1.602613595017,-35.5815989923742,-8.15971912255805));
#49561=CARTESIAN_POINT('Ctrl Pts',(1.61462398371853,-35.5801988565566,-8.17072375022459));
#49562=CARTESIAN_POINT('Ctrl Pts',(1.62401123170297,-35.5791045187746,-8.17932490139875));
#49563=CARTESIAN_POINT('Ctrl Pts',(1.63394272185038,-35.5775439293429,-8.18732229002714));
#49564=CARTESIAN_POINT('Ctrl Pts',(1.64432960286547,-35.5755276116623,-8.19465032514282));
#49565=CARTESIAN_POINT('Ctrl Pts',(1.65751223624117,-35.5729685781358,-8.20395078792408));
#49566=CARTESIAN_POINT('Ctrl Pts',(1.67143040403805,-35.5696742607946,-8.21217315079081));
#49567=CARTESIAN_POINT('Ctrl Pts',(1.68587374540741,-35.565686430912,-8.2192114954254));
#49568=CARTESIAN_POINT('Ctrl Pts',(1.70041483395494,-35.5616716128756,-8.22629747296635));
#49569=CARTESIAN_POINT('Ctrl Pts',(1.7154879825108,-35.5569536553932,-8.23218342574401));
#49570=CARTESIAN_POINT('Ctrl Pts',(1.7308718665687,-35.5515942287824,-8.23681029394356));
#49571=CARTESIAN_POINT('Ctrl Pts',(1.74453974665183,-35.5468326224185,-8.24092105553498));
#49572=CARTESIAN_POINT('Ctrl Pts',(1.75845269437942,-35.5415648512774,-8.24403870478297));
#49573=CARTESIAN_POINT('Ctrl Pts',(1.77245352352828,-35.5358486074623,-8.24615310101329));
#49574=CARTESIAN_POINT('Ctrl Pts',(1.78937968978829,-35.5289380100849,-8.24870927977624));
#49575=CARTESIAN_POINT('Ctrl Pts',(1.8064255637685,-35.521374841914,-8.24979779098238));
#49576=CARTESIAN_POINT('Ctrl Pts',(1.82333732775558,-35.5132798883306,-8.24945548954978));
#49577=CARTESIAN_POINT('Ctrl Pts',(1.83055847689705,-35.5098234264757,-8.24930933036154));
#49578=CARTESIAN_POINT('Ctrl Pts',(1.83775521093275,-35.5062703565462,-8.2489028379445));
#49579=CARTESIAN_POINT('Ctrl Pts',(1.84490789334748,-35.5026317912376,-8.24824123808703));
#49580=CARTESIAN_POINT('Ctrl Pts',(1.84751151403415,-35.5013073309362,-8.24800041164245));
#49581=CARTESIAN_POINT('Ctrl Pts',(1.85010944922896,-35.499971478242,-8.24772578323896));
#49582=CARTESIAN_POINT('Ctrl Pts',(1.85270080612586,-35.4986247745774,-8.24741763123874));
#49583=CARTESIAN_POINT('Ctrl Pts',(1.8536955086597,-35.4981078370806,-8.24729934588183));
#49584=CARTESIAN_POINT('Ctrl Pts',(1.85468986954109,-35.4975889712202,-8.24717603800027));
#49585=CARTESIAN_POINT('Ctrl Pts',(1.85568130399,-35.4970695389,-8.24704805785));
#49586=CARTESIAN_POINT('Origin',(1.88128360390313,-40.0416488169456,-7.95002524253046));
#49587=CARTESIAN_POINT('Ctrl Pts',(1.87043161103,-36.3742356128,-8.24476960824));
#49588=CARTESIAN_POINT('Ctrl Pts',(1.87043161103,-35.2215351205278,-8.24476960824));
#49589=CARTESIAN_POINT('Ctrl Pts',(2.47265813357,-36.3742356128,-8.13634296351));
#49590=CARTESIAN_POINT('Ctrl Pts',(2.47265813357,-35.2215351205278,-8.13634296351));
#49591=CARTESIAN_POINT('Ctrl Pts',(3.05192283465,-36.3742356128,-7.98771609515));
#49592=CARTESIAN_POINT('Ctrl Pts',(3.05192283465,-35.2215351205278,-7.98771609515));
#49593=CARTESIAN_POINT('Ctrl Pts',(3.608285111,-36.3742356128,-7.79892601222));
#49594=CARTESIAN_POINT('Ctrl Pts',(3.608285111,-35.2215351205278,-7.79892601222));
#49595=CARTESIAN_POINT('Ctrl Pts',(4.84313848674,-36.3742356128,-7.27000777732));
#49596=CARTESIAN_POINT('Ctrl Pts',(4.84313848674,-35.2215351205278,-7.27000777732));
#49597=CARTESIAN_POINT('Ctrl Pts',(5.97499470659,-36.3742356128,-6.53839758248));
#49598=CARTESIAN_POINT('Ctrl Pts',(5.97499470659,-35.2215351205278,-6.53839758248));
#49599=CARTESIAN_POINT('Ctrl Pts',(6.59156749188,-36.3742356128,-6.06232184959));
#49600=CARTESIAN_POINT('Ctrl Pts',(6.59156749188,-35.2215351205278,-6.06232184959));
#49601=CARTESIAN_POINT('Ctrl Pts',(7.62010012329,-36.3742356128,-5.1678005996));
#49602=CARTESIAN_POINT('Ctrl Pts',(7.62010012329,-35.2215351205278,-5.1678005996));
#49603=CARTESIAN_POINT('Ctrl Pts',(8.47746400168,-36.3742356128,-4.11735171219));
#49604=CARTESIAN_POINT('Ctrl Pts',(8.47746400168,-35.2215351205278,-4.11735171219));
#49605=CARTESIAN_POINT('Ctrl Pts',(8.78407978672,-36.3742356128,-3.65866522624));
#49606=CARTESIAN_POINT('Ctrl Pts',(8.78407978672,-35.2215351205278,-3.65866522624));
#49607=CARTESIAN_POINT('Ctrl Pts',(9.22504359392,-36.3742356128,-2.71647636201));
#49608=CARTESIAN_POINT('Ctrl Pts',(9.22504359392,-35.2215351205278,-2.71647636201));
#49609=CARTESIAN_POINT('Ctrl Pts',(9.38605456704,-36.3742356128,-1.68617604095));
#49610=CARTESIAN_POINT('Ctrl Pts',(9.38605456704,-35.2215351205278,-1.68617604095));
#49611=CARTESIAN_POINT('Ctrl Pts',(9.40005841918,-36.3742356128,-1.17735235373));
#49612=CARTESIAN_POINT('Ctrl Pts',(9.40005841918,-35.2215351205278,-1.17735235373));
#49613=CARTESIAN_POINT('Ctrl Pts',(9.36972184244,-36.3742356128,-0.530817230024));
#49614=CARTESIAN_POINT('Ctrl Pts',(9.36972184244,-35.2215351205278,-0.530817230024));
#49615=CARTESIAN_POINT('Ctrl Pts',(9.2950327654,-36.3742356128,0.106470788818));
#49616=CARTESIAN_POINT('Ctrl Pts',(9.2950327654,-35.2215351205278,0.106470788818));
#49617=CARTESIAN_POINT('Ctrl Pts',(9.27733443288,-36.3742356128,0.241562002067001));
#49618=CARTESIAN_POINT('Ctrl Pts',(9.27733443288,-35.2215351205278,0.241562002067001));
#49619=CARTESIAN_POINT('Ctrl Pts',(9.25795835827,-36.3742356128,0.376048284641));
#49620=CARTESIAN_POINT('Ctrl Pts',(9.25795835827,-35.2215351205278,0.376048284641));
#49621=CARTESIAN_POINT('Ctrl Pts',(9.23698117862,-36.3742356128,0.509886547165));
#49622=CARTESIAN_POINT('Ctrl Pts',(9.23698117862,-35.2215351205278,0.509886547165));
#49623=CARTESIAN_POINT('',(9.23698117854899,-35.5153448503988,0.509886547089956));
#49624=CARTESIAN_POINT('',(9.23698117862,-36.1242356128,0.509886547139));
#49625=CARTESIAN_POINT('',(9.00070981177086,-35.4796534480026,-3.11774626039934));
#49626=CARTESIAN_POINT('Ctrl Pts',(9.00070981177086,-35.4796534480026,-3.11774626039934));
#49627=CARTESIAN_POINT('Ctrl Pts',(9.02957171740057,-35.4769219470675,-3.04928528637033));
#49628=CARTESIAN_POINT('Ctrl Pts',(9.05680199238443,-35.4745170641086,-2.98008474679654));
#49629=CARTESIAN_POINT('Ctrl Pts',(9.08232187979775,-35.4724444037653,-2.910198820275));
#49630=CARTESIAN_POINT('Ctrl Pts',(9.10927225564361,-35.4702555627901,-2.83639551716526));
#49631=CARTESIAN_POINT('Ctrl Pts',(9.13431510786021,-35.4684371095379,-2.76182792423961));
#49632=CARTESIAN_POINT('Ctrl Pts',(9.15741235945346,-35.4669762581242,-2.68657232100095));
#49633=CARTESIAN_POINT('Ctrl Pts',(9.18148566903293,-35.4654536731453,-2.60813651979576));
#49634=CARTESIAN_POINT('Ctrl Pts',(9.20344567588574,-35.4643193005489,-2.52895350431998));
#49635=CARTESIAN_POINT('Ctrl Pts',(9.22330541366417,-35.4635411664201,-2.44912073619115));
#49636=CARTESIAN_POINT('Ctrl Pts',(9.24419465191341,-35.4627226949283,-2.36514955126694));
#49637=CARTESIAN_POINT('Ctrl Pts',(9.26276050520176,-35.4622980003227,-2.28045974660158));
#49638=CARTESIAN_POINT('Ctrl Pts',(9.27907531337767,-35.4622156178015,-2.19517351658305));
#49639=CARTESIAN_POINT('Ctrl Pts',(9.29723571129714,-35.4621239158735,-2.10023940166805));
#49640=CARTESIAN_POINT('Ctrl Pts',(9.31260699943646,-35.4624557836193,-2.00456669258708));
#49641=CARTESIAN_POINT('Ctrl Pts',(9.32535642051477,-35.4631302190584,-1.90832945811796));
#49642=CARTESIAN_POINT('Ctrl Pts',(9.33904599640173,-35.463854388028,-1.80499559563723));
#49643=CARTESIAN_POINT('Ctrl Pts',(9.34971379577462,-35.4649723642263,-1.70101166885288));
#49644=CARTESIAN_POINT('Ctrl Pts',(9.35763181221748,-35.4663868382239,-1.59658955684038));
#49645=CARTESIAN_POINT('Ctrl Pts',(9.36576400690357,-35.4678395730105,-1.48934288078885));
#49646=CARTESIAN_POINT('Ctrl Pts',(9.37099761991728,-35.4696036037748,-1.38163498160731));
#49647=CARTESIAN_POINT('Ctrl Pts',(9.37366922576191,-35.471596964129,-1.27367781011332));
#49648=CARTESIAN_POINT('Ctrl Pts',(9.37519483192013,-35.4727352618453,-1.21202944758001));
#49649=CARTESIAN_POINT('Ctrl Pts',(9.37588558818129,-35.4739488889969,-1.15029939791678));
#49650=CARTESIAN_POINT('Ctrl Pts',(9.37580612763427,-35.4752287322034,-1.08852272605951));
#49651=CARTESIAN_POINT('Ctrl Pts',(9.3756771929251,-35.4773054384155,-0.988282323516714));
#49652=CARTESIAN_POINT('Ctrl Pts',(9.37352221687252,-35.4795545444975,-0.887915672555842));
#49653=CARTESIAN_POINT('Ctrl Pts',(9.36960764020662,-35.4818966426587,-0.787510754476126));
#49654=CARTESIAN_POINT('Ctrl Pts',(9.3656030093745,-35.4842926203873,-0.684796038440355));
#49655=CARTESIAN_POINT('Ctrl Pts',(9.35975775607616,-35.486786172115,-0.582042878943941));
#49656=CARTESIAN_POINT('Ctrl Pts',(9.3523252340311,-35.4893296612911,-0.479365968570074));
#49657=CARTESIAN_POINT('Ctrl Pts',(9.34529365064581,-35.4917359449351,-0.382227843360345));
#49658=CARTESIAN_POINT('Ctrl Pts',(9.33684172327988,-35.4941875092004,-0.28515935974196));
#49659=CARTESIAN_POINT('Ctrl Pts',(9.32714804515724,-35.4966702396909,-0.18825370987044));
#49660=CARTESIAN_POINT('Ctrl Pts',(9.31792029758086,-35.4990336367396,-0.0960058691202795));
#49661=CARTESIAN_POINT('Ctrl Pts',(9.30756748520679,-35.5014256840601,-0.00390652794974493));
#49662=CARTESIAN_POINT('Ctrl Pts',(9.29620682473956,-35.5038517559769,0.0879838265690647));
#49663=CARTESIAN_POINT('Ctrl Pts',(9.28558220327457,-35.5061206465787,0.173920752143267));
#49664=CARTESIAN_POINT('Ctrl Pts',(9.27407606940699,-35.5084196106949,0.259674395231827));
#49665=CARTESIAN_POINT('Ctrl Pts',(9.26175043835322,-35.5107637359109,0.345222825128153));
#49666=CARTESIAN_POINT('Ctrl Pts',(9.25383028777107,-35.5122700137326,0.400194164436453));
#49667=CARTESIAN_POINT('Ctrl Pts',(9.24557108699713,-35.5137951391701,0.455081343764294));
#49668=CARTESIAN_POINT('Ctrl Pts',(9.23698117833998,-35.5153448508951,0.509886546917127));
#49669=CARTESIAN_POINT('',(8.91162791630276,-35.4775418018592,-3.31601642789431));
#49670=CARTESIAN_POINT('Origin',(8.92974789374037,-35.4242646256046,-3.20847971418429));
#49671=CARTESIAN_POINT('',(2.02993009745,-35.4952697797,-8.21479904026));
#49672=CARTESIAN_POINT('Ctrl Pts',(2.02993009745,-35.4952697797,-8.21479904026));
#49673=CARTESIAN_POINT('Ctrl Pts',(2.1975178934536,-35.4899768112507,-8.1819801957285));
#49674=CARTESIAN_POINT('Ctrl Pts',(2.36364233174554,-35.4848180347522,-8.14522817489977));
#49675=CARTESIAN_POINT('Ctrl Pts',(2.52813765848659,-35.4798773000524,-8.10448244801098));
#49676=CARTESIAN_POINT('Ctrl Pts',(2.68928215337265,-35.4750372099821,-8.06456672694862));
#49677=CARTESIAN_POINT('Ctrl Pts',(2.84886323116559,-35.4704064674222,-8.02081818934416));
#49678=CARTESIAN_POINT('Ctrl Pts',(3.00675547641862,-35.4660483132631,-7.97321492935763));
#49679=CARTESIAN_POINT('Ctrl Pts',(3.16170539309467,-35.4617713734886,-7.92649875810679));
#49680=CARTESIAN_POINT('Ctrl Pts',(3.3150288310632,-35.4577570434877,-7.8760700511927));
#49681=CARTESIAN_POINT('Ctrl Pts',(3.46663688737487,-35.4540485714109,-7.82194436965912));
#49682=CARTESIAN_POINT('Ctrl Pts',(3.61564458295988,-35.4504037065419,-7.76874704444108));
#49683=CARTESIAN_POINT('Ctrl Pts',(3.76299523221431,-35.4470543738175,-7.71197835196257));
#49684=CARTESIAN_POINT('Ctrl Pts',(3.90863338135848,-35.4440243272187,-7.65169038609799));
#49685=CARTESIAN_POINT('Ctrl Pts',(4.05084484294492,-35.4410655739112,-7.5928209223479));
#49686=CARTESIAN_POINT('Ctrl Pts',(4.19142347414132,-35.438411301993,-7.53059578517629));
#49687=CARTESIAN_POINT('Ctrl Pts',(4.33034523746524,-35.4360661416366,-7.46510065395307));
#49688=CARTESIAN_POINT('Ctrl Pts',(4.46756230134255,-35.4337497585825,-7.40040920900103));
#49689=CARTESIAN_POINT('Ctrl Pts',(4.60316289372039,-35.4317350148565,-7.33252741469367));
#49690=CARTESIAN_POINT('Ctrl Pts',(4.73715106390426,-35.4300082452412,-7.26157592932336));
#49691=CARTESIAN_POINT('Ctrl Pts',(4.86874877422086,-35.4283122826252,-7.19189027718346));
#49692=CARTESIAN_POINT('Ctrl Pts',(4.99879109554046,-35.4268941515193,-7.11924342586109));
#49693=CARTESIAN_POINT('Ctrl Pts',(5.12730826788093,-35.4257225409936,-7.04378791082896));
#49694=CARTESIAN_POINT('Ctrl Pts',(5.21963571122407,-35.4248808495491,-6.98958025388953));
#49695=CARTESIAN_POINT('Ctrl Pts',(5.311176557266,-35.4241660139734,-6.93392380881406));
#49696=CARTESIAN_POINT('Ctrl Pts',(5.40195064262958,-35.423560213071,-6.87688796232893));
#49697=CARTESIAN_POINT('Ctrl Pts',(5.57266510194519,-35.4224209124316,-6.76962338725426));
#49698=CARTESIAN_POINT('Ctrl Pts',(5.74066892757427,-35.4216668875503,-6.65748707456149));
#49699=CARTESIAN_POINT('Ctrl Pts',(5.90607489885303,-35.4211448538569,-6.54086756734377));
#49700=CARTESIAN_POINT('Ctrl Pts',(6.02322228246083,-35.4207751278979,-6.45827278528984));
#49701=CARTESIAN_POINT('Ctrl Pts',(6.13906856601719,-35.4205205600216,-6.3734289106523));
#49702=CARTESIAN_POINT('Ctrl Pts',(6.25362891329586,-35.4203360786063,-6.28645115877483));
#49703=CARTESIAN_POINT('Ctrl Pts',(6.35123185698643,-35.4201789044216,-6.21234799113884));
#49704=CARTESIAN_POINT('Ctrl Pts',(6.44790169045711,-35.4200724071828,-6.13669582147483));
#49705=CARTESIAN_POINT('Ctrl Pts',(6.54361636231053,-35.4200029704147,-6.05954834485368));
#49706=CARTESIAN_POINT('Ctrl Pts',(6.63435282649732,-35.4199371451165,-5.98641337908524));
#49707=CARTESIAN_POINT('Ctrl Pts',(6.72423135978761,-35.4199043868614,-5.91193471524081));
#49708=CARTESIAN_POINT('Ctrl Pts',(6.81319693299893,-35.4199101028679,-5.83614049502093));
#49709=CARTESIAN_POINT('Ctrl Pts',(6.90000716025135,-35.4199156803943,-5.76218252179369));
#49710=CARTESIAN_POINT('Ctrl Pts',(6.98594861911178,-35.4199576407568,-5.68697211269862));
#49711=CARTESIAN_POINT('Ctrl Pts',(7.07092770952919,-35.4200612492516,-5.61051622553605));
#49712=CARTESIAN_POINT('Ctrl Pts',(7.15069751739736,-35.4201585064673,-5.53874714211339));
#49713=CARTESIAN_POINT('Ctrl Pts',(7.22961939495362,-35.4203100434311,-5.46588058088319));
#49714=CARTESIAN_POINT('Ctrl Pts',(7.30757463585883,-35.4205566121551,-5.39190447875861));
#49715=CARTESIAN_POINT('Ctrl Pts',(7.31266542004049,-35.4205727140637,-5.38707354800728));
#49716=CARTESIAN_POINT('Ctrl Pts',(7.31775206621492,-35.4205892288169,-5.38223787887034));
#49717=CARTESIAN_POINT('Ctrl Pts',(7.32283453462144,-35.4206061710013,-5.37739746516443));
#49718=CARTESIAN_POINT('Ctrl Pts',(7.38569118267643,-35.4208157008674,-5.31753439147313));
#49719=CARTESIAN_POINT('Ctrl Pts',(7.44791297110117,-35.4210888089051,-5.25694587282929));
#49720=CARTESIAN_POINT('Ctrl Pts',(7.50945481532502,-35.4214338225053,-5.19559372525316));
#49721=CARTESIAN_POINT('Ctrl Pts',(7.57397402407752,-35.4217955276959,-5.13127339058004));
#49722=CARTESIAN_POINT('Ctrl Pts',(7.63774567323264,-35.4222365134176,-5.06611357288604));
#49723=CARTESIAN_POINT('Ctrl Pts',(7.70066498678859,-35.4227880797105,-5.00006853898814));
#49724=CARTESIAN_POINT('Ctrl Pts',(7.76988847984058,-35.4233949100029,-4.92740614509402));
#49725=CARTESIAN_POINT('Ctrl Pts',(7.8380802462688,-35.4241358884641,-4.8536719426947));
#49726=CARTESIAN_POINT('Ctrl Pts',(7.90503975752188,-35.4250742536816,-4.77880693738246));
#49727=CARTESIAN_POINT('Ctrl Pts',(7.97788603307253,-35.4260951155417,-4.69736015403509));
#49728=CARTESIAN_POINT('Ctrl Pts',(8.04927322937182,-35.4273503513893,-4.61457442442277));
#49729=CARTESIAN_POINT('Ctrl Pts',(8.11887950897483,-35.4289372554664,-4.53038316516456));
#49730=CARTESIAN_POINT('Ctrl Pts',(8.19656257649718,-35.4307082964886,-4.43642274499775));
#49731=CARTESIAN_POINT('Ctrl Pts',(8.27202600384564,-35.4328940611376,-4.34071049739949));
#49732=CARTESIAN_POINT('Ctrl Pts',(8.34476245153336,-35.4356296730107,-4.24317952523622));
#49733=CARTESIAN_POINT('Ctrl Pts',(8.4121335395811,-35.4381634941448,-4.15284286566765));
#49734=CARTESIAN_POINT('Ctrl Pts',(8.47716266034837,-35.4411702157103,-4.06094562941393));
#49735=CARTESIAN_POINT('Ctrl Pts',(8.53942996026822,-35.4447364851622,-3.96746489499558));
#49736=CARTESIAN_POINT('Ctrl Pts',(8.59656003661319,-35.4480085275715,-3.88169657838349));
#49737=CARTESIAN_POINT('Ctrl Pts',(8.65136388597018,-35.4517521215922,-3.79459524998933));
#49738=CARTESIAN_POINT('Ctrl Pts',(8.70352740691122,-35.4560050698587,-3.70617136906099));
#49739=CARTESIAN_POINT('Ctrl Pts',(8.75100223690881,-35.4598757440827,-3.62569542267033));
#49740=CARTESIAN_POINT('Ctrl Pts',(8.79628946802519,-35.4641684489054,-3.54412410061856));
#49741=CARTESIAN_POINT('Ctrl Pts',(8.83917328519815,-35.4688825330422,-3.46148888657376));
#49742=CARTESIAN_POINT('Ctrl Pts',(8.86415243523348,-35.4716284130196,-3.41335517213549));
#49743=CARTESIAN_POINT('Ctrl Pts',(8.88831657813022,-35.4745166981789,-3.36486093276358));
#49744=CARTESIAN_POINT('Ctrl Pts',(8.91162790031208,-35.4775418017954,-3.31601642164564));
#49745=CARTESIAN_POINT('Origin',(1.87573872781907,-33.3311293309267,-7.7757813654712));
#49746=CARTESIAN_POINT('Ctrl Pts',(8.75956299023,-36.3742356128,2.0634404101));
#49747=CARTESIAN_POINT('Ctrl Pts',(8.75956299023,-35.3373826802055,2.0634404101));
#49748=CARTESIAN_POINT('Ctrl Pts',(8.92890465395,-36.3742356128,1.78598462948));
#49749=CARTESIAN_POINT('Ctrl Pts',(8.92890465395,-35.3373826802055,1.78598462948));
#49750=CARTESIAN_POINT('Ctrl Pts',(9.07291332076,-36.3742356128,1.49306717121));
#49751=CARTESIAN_POINT('Ctrl Pts',(9.07291332076,-35.3373826802055,1.49306717121));
#49752=CARTESIAN_POINT('Ctrl Pts',(9.12674872803,-36.3742356128,1.15064845916));
#49753=CARTESIAN_POINT('Ctrl Pts',(9.12674872803,-35.3373826802055,1.15064845916));
#49754=CARTESIAN_POINT('Ctrl Pts',(9.18664865847,-36.3742356128,0.831017278590001));
#49755=CARTESIAN_POINT('Ctrl Pts',(9.18664865847,-35.3373826802055,0.831017278590001));
#49756=CARTESIAN_POINT('Ctrl Pts',(9.23698117862,-36.3742356128,0.509886547135));
#49757=CARTESIAN_POINT('Ctrl Pts',(9.23698117862,-35.3373826802055,0.509886547135));
#49758=CARTESIAN_POINT('',(8.75956299007003,-35.6438772168027,2.06344041036242));
#49759=CARTESIAN_POINT('',(8.75956299023,-36.1242356128,2.0634404101));
#49760=CARTESIAN_POINT('',(9.22799880548,-35.5169181946,0.566467047115));
#49761=CARTESIAN_POINT('Ctrl Pts',(9.22799880548,-35.5169181946,0.566467047115));
#49762=CARTESIAN_POINT('Ctrl Pts',(9.22709573015,-35.5170698741,0.572088224967));
#49763=CARTESIAN_POINT('Ctrl Pts',(9.22618896279,-35.5172202096,0.57771674331));
#49764=CARTESIAN_POINT('Ctrl Pts',(9.22528372099,-35.5173684625,0.58332051525));
#49765=CARTESIAN_POINT('Ctrl Pts',(9.21064489493,-35.5197392711,0.67370187071));
#49766=CARTESIAN_POINT('Ctrl Pts',(9.19547141468,-35.5218042907,0.763606652472));
#49767=CARTESIAN_POINT('Ctrl Pts',(9.18087022532,-35.5239641094,0.847743194451));
#49768=CARTESIAN_POINT('Ctrl Pts',(9.1488371776,-35.5298747429,1.02282666839));
#49769=CARTESIAN_POINT('Ctrl Pts',(9.1112963015,-35.5399157471,1.19686722852));
#49770=CARTESIAN_POINT('Ctrl Pts',(9.08965016934,-35.5466085932,1.28690888429));
#49771=CARTESIAN_POINT('Ctrl Pts',(9.04054093324,-35.5631550729,1.46510383868));
#49772=CARTESIAN_POINT('Ctrl Pts',(8.97813093642,-35.5847442368,1.63735111856));
#49773=CARTESIAN_POINT('Ctrl Pts',(8.94306195143,-35.596524942,1.72177132487));
#49774=CARTESIAN_POINT('Ctrl Pts',(8.89434925659,-35.6115263375,1.82461373716));
#49775=CARTESIAN_POINT('Ctrl Pts',(8.84001654494,-35.6256966309,1.92519756404));
#49776=CARTESIAN_POINT('Ctrl Pts',(8.82896553279,-35.6284769797,1.94517168962));
#49777=CARTESIAN_POINT('Ctrl Pts',(8.80877742677,-35.6333588617,1.98085549694));
#49778=CARTESIAN_POINT('Ctrl Pts',(8.78793522997,-35.6380188734,2.01638522454));
#49779=CARTESIAN_POINT('Ctrl Pts',(8.77859596185,-35.6400309319,2.03207294823));
#49780=CARTESIAN_POINT('Ctrl Pts',(8.76913081737,-35.641984033,2.04776380401));
#49781=CARTESIAN_POINT('Ctrl Pts',(8.75956299023,-35.6438772164,2.0634404101));
#49782=CARTESIAN_POINT('Ctrl Pts',(9.23698117862,-35.5153448509,0.509886547139));
#49783=CARTESIAN_POINT('Ctrl Pts',(9.23547079661,-35.5156173384,0.519523062039));
#49784=CARTESIAN_POINT('Ctrl Pts',(9.23395444171,-35.5158907435,0.529141367463));
#49785=CARTESIAN_POINT('Ctrl Pts',(9.2324173579,-35.5161611506,0.538838588998));
#49786=CARTESIAN_POINT('Ctrl Pts',(9.2306125394,-35.5164751965,0.550165758707));
#49787=CARTESIAN_POINT('Ctrl Pts',(9.22879492211,-35.5167839497,0.561507557195));
#49788=CARTESIAN_POINT('Ctrl Pts',(9.22852978607,-35.5168288241,0.563160610681));
#49789=CARTESIAN_POINT('Ctrl Pts',(9.22826440991,-35.5168735732,0.564813796021));
#49790=CARTESIAN_POINT('Ctrl Pts',(9.22799880548,-35.5169181946,0.566467047115));
#49791=CARTESIAN_POINT('Ctrl Pts',(8.75956299024,-36.3742356128,2.0634404101));
#49792=CARTESIAN_POINT('Ctrl Pts',(8.75956299024,-35.2767450158758,2.0634404101));
#49793=CARTESIAN_POINT('Ctrl Pts',(8.72637376563,-36.3742356128,2.11781888978));
#49794=CARTESIAN_POINT('Ctrl Pts',(8.72637376563,-35.2767450158758,2.11781888978));
#49795=CARTESIAN_POINT('Ctrl Pts',(8.6915484,-36.3742356128,2.17268982337));
#49796=CARTESIAN_POINT('Ctrl Pts',(8.6915484,-35.2767450158758,2.17268982337));
#49797=CARTESIAN_POINT('Ctrl Pts',(8.65506636668,-36.3742356128,2.22762960985));
#49798=CARTESIAN_POINT('Ctrl Pts',(8.65506636668,-35.2767450158758,2.22762960985));
#49799=CARTESIAN_POINT('Ctrl Pts',(8.53055023262,-36.3742356128,2.40503324452));
#49800=CARTESIAN_POINT('Ctrl Pts',(8.53055023262,-35.2767450158758,2.40503324452));
#49801=CARTESIAN_POINT('Ctrl Pts',(8.3876008666,-36.3742356128,2.56660232663));
#49802=CARTESIAN_POINT('Ctrl Pts',(8.3876008666,-35.2767450158758,2.56660232663));
#49803=CARTESIAN_POINT('Ctrl Pts',(8.27908544119,-36.3742356128,2.66027026629));
#49804=CARTESIAN_POINT('Ctrl Pts',(8.27908544119,-35.2767450158758,2.66027026629));
#49805=CARTESIAN_POINT('Ctrl Pts',(8.01327762974,-36.3742356128,2.78696551824));
#49806=CARTESIAN_POINT('Ctrl Pts',(8.01327762974,-35.2767450158758,2.78696551824));
#49807=CARTESIAN_POINT('Ctrl Pts',(7.71906576509,-36.3742356128,2.71717075777));
#49808=CARTESIAN_POINT('Ctrl Pts',(7.71906576509,-35.2767450158758,2.71717075777));
#49809=CARTESIAN_POINT('Ctrl Pts',(7.55641153588,-36.3742356128,2.61428156978));
#49810=CARTESIAN_POINT('Ctrl Pts',(7.55641153588,-35.2767450158758,2.61428156978));
#49811=CARTESIAN_POINT('Ctrl Pts',(7.38865661676,-36.3742356128,2.45617777771));
#49812=CARTESIAN_POINT('Ctrl Pts',(7.38865661676,-35.2767450158758,2.45617777771));
#49813=CARTESIAN_POINT('Ctrl Pts',(7.26550535688,-36.3742356128,2.27753774962));
#49814=CARTESIAN_POINT('Ctrl Pts',(7.26550535688,-35.2767450158758,2.27753774962));
#49815=CARTESIAN_POINT('Ctrl Pts',(7.24701042964,-36.3742356128,2.24853650952));
#49816=CARTESIAN_POINT('Ctrl Pts',(7.24701042964,-35.2767450158758,2.24853650952));
#49817=CARTESIAN_POINT('Ctrl Pts',(7.2297761181,-36.3742356128,2.21919784335));
#49818=CARTESIAN_POINT('Ctrl Pts',(7.2297761181,-35.2767450158758,2.21919784335));
#49819=CARTESIAN_POINT('Ctrl Pts',(7.21384189758,-36.3742356128,2.18958432613));
#49820=CARTESIAN_POINT('Ctrl Pts',(7.21384189758,-35.2767450158758,2.18958432613));
#49821=CARTESIAN_POINT('',(7.21384189757838,-35.4651148398171,2.18958432618296));
#49822=CARTESIAN_POINT('',(7.21384189758,-36.1242356128,2.18958432614));
#49823=CARTESIAN_POINT('',(7.23334333080301,-35.4800020975,2.22433302562685));
#49824=CARTESIAN_POINT('Ctrl Pts',(7.23334333044,-35.4800020975,2.22433302572));
#49825=CARTESIAN_POINT('Ctrl Pts',(7.22937402512,-35.477126751,2.21754286118));
#49826=CARTESIAN_POINT('Ctrl Pts',(7.22542564343,-35.4742071929,2.21065452768));
#49827=CARTESIAN_POINT('Ctrl Pts',(7.22151371785,-35.4712377752,2.20368850558));
#49828=CARTESIAN_POINT('Ctrl Pts',(7.21764954964,-35.4682109676,2.19666066586));
#49829=CARTESIAN_POINT('Ctrl Pts',(7.21384189758,-35.46511484,2.18958432614));
#49830=CARTESIAN_POINT('',(8.49626470339955,-35.699502272635,2.43550539329785));
#49831=CARTESIAN_POINT('Ctrl Pts',(8.49626470706,-35.699502273,2.43550539877));
#49832=CARTESIAN_POINT('Ctrl Pts',(8.45240512852,-35.7099399342,2.48655698047));
#49833=CARTESIAN_POINT('Ctrl Pts',(8.40764108873,-35.7197613468,2.53363446576));
#49834=CARTESIAN_POINT('Ctrl Pts',(8.36047222003,-35.7299082045,2.5777319381));
#49835=CARTESIAN_POINT('Ctrl Pts',(8.24494252704,-35.7503872354,2.66806485365));
#49836=CARTESIAN_POINT('Ctrl Pts',(8.12018530542,-35.7590565367,2.723855906));
#49837=CARTESIAN_POINT('Ctrl Pts',(8.0441099093,-35.7553391142,2.74240669266));
#49838=CARTESIAN_POINT('Ctrl Pts',(7.81966214074,-35.7098598702,2.74888110871));
#49839=CARTESIAN_POINT('Ctrl Pts',(7.59696106493,-35.6321549665,2.64143245401));
#49840=CARTESIAN_POINT('Ctrl Pts',(7.45050807009,-35.5975831903,2.52611015512));
#49841=CARTESIAN_POINT('Ctrl Pts',(7.3239386903,-35.5456357901,2.37931366962));
#49842=CARTESIAN_POINT('Ctrl Pts',(7.23334333044,-35.4800020975,2.22433302572));
#49843=CARTESIAN_POINT('',(8.73000675245248,-35.6496340209958,2.1111701504857));
#49844=CARTESIAN_POINT('Ctrl Pts',(8.73000528472,-35.6496341999,2.11117245845));
#49845=CARTESIAN_POINT('Ctrl Pts',(8.71278579373065,-35.6529734545507,2.13857243132976));
#49846=CARTESIAN_POINT('Ctrl Pts',(8.69523611065439,-35.656418433528,2.16578280028398));
#49847=CARTESIAN_POINT('Ctrl Pts',(8.67736328843596,-35.6599993397373,2.19267530487441));
#49848=CARTESIAN_POINT('Ctrl Pts',(8.65990881423403,-35.6634964279019,2.21893833831492));
#49849=CARTESIAN_POINT('Ctrl Pts',(8.64214969971165,-35.6671228124049,2.24489443760551));
#49850=CARTESIAN_POINT('Ctrl Pts',(8.6240892075043,-35.6709094567015,2.27040574861869));
#49851=CARTESIAN_POINT('Ctrl Pts',(8.60885152877019,-35.6741042571869,2.29192970028301));
#49852=CARTESIAN_POINT('Ctrl Pts',(8.59340033381773,-35.6774130775882,2.31313561363373));
#49853=CARTESIAN_POINT('Ctrl Pts',(8.57770836660362,-35.6808587827496,2.33395912375569));
#49854=CARTESIAN_POINT('Ctrl Pts',(8.57480139519109,-35.6814971072033,2.33781672476946));
#49855=CARTESIAN_POINT('Ctrl Pts',(8.57188604813872,-35.6821401439685,2.3416612893117));
#49856=CARTESIAN_POINT('Ctrl Pts',(8.56896198405368,-35.6827880598152,2.34549254173609));
#49857=CARTESIAN_POINT('Ctrl Pts',(8.56143090936174,-35.6844567997929,2.35536012580152));
#49858=CARTESIAN_POINT('Ctrl Pts',(8.55384786331649,-35.6861566070827,2.36513232166256));
#49859=CARTESIAN_POINT('Ctrl Pts',(8.54621303383084,-35.6878884842043,2.37479733602594));
#49860=CARTESIAN_POINT('Ctrl Pts',(8.53873858847129,-35.6895839799504,2.38425931836546));
#49861=CARTESIAN_POINT('Ctrl Pts',(8.53121142039016,-35.6913109462438,2.39362216719067));
#49862=CARTESIAN_POINT('Ctrl Pts',(8.52362054975123,-35.6930722906216,2.40288673572145));
#49863=CARTESIAN_POINT('Ctrl Pts',(8.51695920442706,-35.6946179529959,2.41101682951418));
#49864=CARTESIAN_POINT('Ctrl Pts',(8.51024738112154,-35.6961904182621,2.41907287662946));
#49865=CARTESIAN_POINT('Ctrl Pts',(8.50349797791776,-35.6977863767698,2.42703115952841));
#49866=CARTESIAN_POINT('Ctrl Pts',(8.50255616499077,-35.6980090771046,2.42814165974369));
#49867=CARTESIAN_POINT('Ctrl Pts',(8.50161367399323,-35.6982322214535,2.42925019294274));
#49868=CARTESIAN_POINT('Ctrl Pts',(8.50067059768458,-35.6984557864418,2.43035662659535));
#49869=CARTESIAN_POINT('Ctrl Pts',(8.49920411912565,-35.6988034287893,2.43207712494054));
#49870=CARTESIAN_POINT('Ctrl Pts',(8.49773226797996,-35.6991530223845,2.43379716100814));
#49871=CARTESIAN_POINT('Ctrl Pts',(8.49626469608749,-35.6995022721787,2.43550538236112));
#49872=CARTESIAN_POINT('Origin',(8.8025233360182,-35.5994617475288,1.55277754717549));
#49873=CARTESIAN_POINT('Ctrl Pts',(7.21384189758,-36.3742356128,2.18958432614));
#49874=CARTESIAN_POINT('Ctrl Pts',(7.21384189758,-35.1742356128,2.18958432614));
#49875=CARTESIAN_POINT('Ctrl Pts',(7.13908599018,-36.3742356128,2.05065155888));
#49876=CARTESIAN_POINT('Ctrl Pts',(7.13908599018,-35.1742356128,2.05065155888));
#49877=CARTESIAN_POINT('Ctrl Pts',(7.08904524264,-36.3742356128,1.89842024269));
#49878=CARTESIAN_POINT('Ctrl Pts',(7.08904524264,-35.1742356128,1.89842024269));
#49879=CARTESIAN_POINT('Ctrl Pts',(7.10533215541,-36.3742356128,1.72680915639));
#49880=CARTESIAN_POINT('Ctrl Pts',(7.10533215541,-35.1742356128,1.72680915639));
#49881=CARTESIAN_POINT('Ctrl Pts',(7.09439724612,-36.3742356128,1.56936004643));
#49882=CARTESIAN_POINT('Ctrl Pts',(7.09439724612,-35.1742356128,1.56936004643));
#49883=CARTESIAN_POINT('Ctrl Pts',(7.07911993306,-36.3742356128,1.41233341424));
#49884=CARTESIAN_POINT('Ctrl Pts',(7.07911993306,-35.1742356128,1.41233341424));
#49885=CARTESIAN_POINT('',(7.07911993306,-35.3742356128,1.41233341424));
#49886=CARTESIAN_POINT('',(7.07911993306,-36.1242356128,1.41233341424));
#49887=CARTESIAN_POINT('',(7.1397347564578,-35.374237430427,2.0065547463937));
#49888=CARTESIAN_POINT('Ctrl Pts',(7.07911993306,-35.3742356128,1.41233341424));
#49889=CARTESIAN_POINT('Ctrl Pts',(7.08088379359945,-35.3742356128,1.43046208289637));
#49890=CARTESIAN_POINT('Ctrl Pts',(7.08257391393288,-35.3742355920726,1.44859911701881));
#49891=CARTESIAN_POINT('Ctrl Pts',(7.08413990039285,-35.3742355563688,1.46677978317043));
#49892=CARTESIAN_POINT('Ctrl Pts',(7.0857719589442,-35.3742355191587,1.48572752787993));
#49893=CARTESIAN_POINT('Ctrl Pts',(7.08726945163805,-35.3742354656818,1.50472259826732));
#49894=CARTESIAN_POINT('Ctrl Pts',(7.08862788994042,-35.3742354024484,1.52378297170932));
#49895=CARTESIAN_POINT('Ctrl Pts',(7.09010880652105,-35.3742353335137,1.54456184919967));
#49896=CARTESIAN_POINT('Ctrl Pts',(7.09142454145998,-35.3742352529839,1.56541838105122));
#49897=CARTESIAN_POINT('Ctrl Pts',(7.0926283564623,-35.3742351692935,1.58635022088257));
#49898=CARTESIAN_POINT('Ctrl Pts',(7.09392979130781,-35.3742350788164,1.60897946680883));
#49899=CARTESIAN_POINT('Ctrl Pts',(7.09510098835278,-35.3742349846454,1.63169662189142));
#49900=CARTESIAN_POINT('Ctrl Pts',(7.09627031081491,-35.374234897438,1.65447046219548));
#49901=CARTESIAN_POINT('Ctrl Pts',(7.09759721920307,-35.3742347984778,1.68031346163214));
#49902=CARTESIAN_POINT('Ctrl Pts',(7.09892280102895,-35.3742347084845,1.70622930734304));
#49903=CARTESIAN_POINT('Ctrl Pts',(7.10049797330183,-35.3742346430312,1.73213889512637));
#49904=CARTESIAN_POINT('Ctrl Pts',(7.10268355309499,-35.3742345522134,1.76808891309181));
#49905=CARTESIAN_POINT('Ctrl Pts',(7.10535563162098,-35.3742345086401,1.80402663896773));
#49906=CARTESIAN_POINT('Ctrl Pts',(7.10925382044881,-35.3742345539108,1.83967755757583));
#49907=CARTESIAN_POINT('Ctrl Pts',(7.11201818443795,-35.3742345860141,1.86495907161537));
#49908=CARTESIAN_POINT('Ctrl Pts',(7.11540160752117,-35.3742346627953,1.89009455114752));
#49909=CARTESIAN_POINT('Ctrl Pts',(7.11963758304748,-35.3742347990894,1.91498267217133));
#49910=CARTESIAN_POINT('Ctrl Pts',(7.12328042918059,-35.3742349162993,1.93638591089839));
#49911=CARTESIAN_POINT('Ctrl Pts',(7.12755425624601,-35.3742350775227,1.95760586664661));
#49912=CARTESIAN_POINT('Ctrl Pts',(7.13256782595141,-35.3742352921947,1.97858502102889));
#49913=CARTESIAN_POINT('Ctrl Pts',(7.13480768313481,-35.3742353881014,1.98795764620536));
#49914=CARTESIAN_POINT('Ctrl Pts',(7.13719457595005,-35.374235494676,1.99728233675496));
#49915=CARTESIAN_POINT('Ctrl Pts',(7.13973478937165,-35.37423561276,2.00655473739996));
#49916=CARTESIAN_POINT('Ctrl Pts',(7.21384189752768,-35.4651148399886,2.18958432613476));
#49917=CARTESIAN_POINT('Ctrl Pts',(7.20248970608986,-35.4558376974459,2.16852385244726));
#49918=CARTESIAN_POINT('Ctrl Pts',(7.19216154685804,-35.4455454559162,2.14764262477417));
#49919=CARTESIAN_POINT('Ctrl Pts',(7.18277070542258,-35.4348282931029,2.12663643219701));
#49920=CARTESIAN_POINT('Ctrl Pts',(7.17770336693684,-35.4290452658892,2.11530140020689));
#49921=CARTESIAN_POINT('Ctrl Pts',(7.17290922441346,-35.4231375971107,2.10393011818054));
#49922=CARTESIAN_POINT('Ctrl Pts',(7.16837646591349,-35.4171920851989,2.09247569166495));
#49923=CARTESIAN_POINT('Ctrl Pts',(7.1586926057656,-35.404489995321,2.06800426561125));
#49924=CARTESIAN_POINT('Ctrl Pts',(7.15020429789434,-35.3915941161304,2.04315346963811));
#49925=CARTESIAN_POINT('Ctrl Pts',(7.14282824899172,-35.3794131715241,2.01756660856244));
#49926=CARTESIAN_POINT('Ctrl Pts',(7.14201563347066,-35.37807120311,2.01474771721293));
#49927=CARTESIAN_POINT('Ctrl Pts',(7.14121690146011,-35.376735446728,2.01192135159036));
#49928=CARTESIAN_POINT('Ctrl Pts',(7.1404309617392,-35.3754137600701,2.0090835975648));
#49929=CARTESIAN_POINT('Ctrl Pts',(7.1401977511474,-35.375021578177,2.00824155551238));
#49930=CARTESIAN_POINT('Ctrl Pts',(7.13996568730528,-35.3746302925694,2.00739857926709));
#49931=CARTESIAN_POINT('Ctrl Pts',(7.13973478936,-35.3742392475,2.00655473738));
#49932=CARTESIAN_POINT('Ctrl Pts',(7.07911993306,-36.3742356128,1.41233341424));
#49933=CARTESIAN_POINT('Ctrl Pts',(7.07911993306,-35.17422421556,1.41233341424));
#49934=CARTESIAN_POINT('Ctrl Pts',(7.02062825816,-36.3742356128,0.811131443794));
#49935=CARTESIAN_POINT('Ctrl Pts',(7.02062825816,-35.17422421556,0.811131443794));
#49936=CARTESIAN_POINT('Ctrl Pts',(6.90206842567,-36.3742356128,0.252977206386));
#49937=CARTESIAN_POINT('Ctrl Pts',(6.90206842567,-35.17422421556,0.252977206386));
#49938=CARTESIAN_POINT('Ctrl Pts',(6.72344043556,-36.3742356128,-0.262129297982999));
#49939=CARTESIAN_POINT('Ctrl Pts',(6.72344043556,-35.17422421556,-0.262129297983));
#49940=CARTESIAN_POINT('Ctrl Pts',(6.21056508527,-36.3742356128,-1.27642010253));
#49941=CARTESIAN_POINT('Ctrl Pts',(6.21056508527,-35.17422421556,-1.27642010253));
#49942=CARTESIAN_POINT('Ctrl Pts',(5.42037231907,-36.3742356128,-2.09197189854));
#49943=CARTESIAN_POINT('Ctrl Pts',(5.42037231907,-35.17422421556,-2.09197189854));
#49944=CARTESIAN_POINT('Ctrl Pts',(4.91868712629,-36.3742356128,-2.4711621885));
#49945=CARTESIAN_POINT('Ctrl Pts',(4.91868712629,-35.17422421556,-2.4711621885));
#49946=CARTESIAN_POINT('Ctrl Pts',(4.33774769283,-36.3742356128,-2.79355507478));
#49947=CARTESIAN_POINT('Ctrl Pts',(4.33774769283,-35.17422421556,-2.79355507478));
#49948=CARTESIAN_POINT('Ctrl Pts',(3.67755401866,-36.3742356128,-3.05915055738));
#49949=CARTESIAN_POINT('Ctrl Pts',(3.67755401866,-35.17422421556,-3.05915055738));
#49950=CARTESIAN_POINT('',(3.67755401867,-35.5065774118,-3.05915055738));
#49951=CARTESIAN_POINT('',(3.67755401867,-36.1242356128,-3.05915055738));
#49952=CARTESIAN_POINT('',(7.05021190275089,-35.3742261150874,1.16209541224075));
#49953=CARTESIAN_POINT('Ctrl Pts',(7.05021190275,-35.3742261151,1.16209541223));
#49954=CARTESIAN_POINT('Ctrl Pts',(7.01549246939,-35.4131252568,0.903392902078));
#49955=CARTESIAN_POINT('Ctrl Pts',(6.96767646618,-35.4506441608,0.642127552041));
#49956=CARTESIAN_POINT('Ctrl Pts',(6.90349674466,-35.485563689,0.372787607728));
#49957=CARTESIAN_POINT('Ctrl Pts',(6.71982081074,-35.5526247648,-0.221149174844));
#49958=CARTESIAN_POINT('Ctrl Pts',(6.43798249823,-35.5965248091,-0.799107100072));
#49959=CARTESIAN_POINT('Ctrl Pts',(6.25293978467,-35.6126874115,-1.1016283265));
#49960=CARTESIAN_POINT('Ctrl Pts',(5.73382235555,-35.6343159234,-1.78819570677));
#49961=CARTESIAN_POINT('Ctrl Pts',(5.06131871348,-35.6148773502,-2.35107992573));
#49962=CARTESIAN_POINT('Ctrl Pts',(4.62352979415,-35.5904307331,-2.63143094545));
#49963=CARTESIAN_POINT('Ctrl Pts',(4.15886281142,-35.5534449291,-2.86552034537));
#49964=CARTESIAN_POINT('Ctrl Pts',(3.67755401867,-35.5065774118,-3.05915055738));
#49965=CARTESIAN_POINT('Ctrl Pts',(7.05021164825251,-35.3742261150622,1.16209544641769));
#49966=CARTESIAN_POINT('Ctrl Pts',(7.05298995234347,-35.3742266401801,1.18279723134882));
#49967=CARTESIAN_POINT('Ctrl Pts',(7.05571064340935,-35.3742477797274,1.20381716459059));
#49968=CARTESIAN_POINT('Ctrl Pts',(7.0582960532776,-35.3742431701946,1.22454392284646));
#49969=CARTESIAN_POINT('Ctrl Pts',(7.06089275591971,-35.3742385405279,1.24536121320582));
#49970=CARTESIAN_POINT('Ctrl Pts',(7.06339480482353,-35.3742375427219,1.26620204691362));
#49971=CARTESIAN_POINT('Ctrl Pts',(7.06580506972233,-35.3742369799114,1.28708281574342));
#49972=CARTESIAN_POINT('Ctrl Pts',(7.07061980686755,-35.3742358556428,1.32879417010786));
#49973=CARTESIAN_POINT('Ctrl Pts',(7.07505478224174,-35.3742356535495,1.37055008889877));
#49974=CARTESIAN_POINT('Ctrl Pts',(7.07911993306,-35.3742356128,1.41233341424));
#49975=CARTESIAN_POINT('Origin',(3.78952269078,-36.1242356128,-3.33747234321));
#49976=CARTESIAN_POINT('',(3.52268743213354,-35.4813642832762,-3.20036310945193));
#49977=CARTESIAN_POINT('Origin',(3.61904102711591,-42.5155158381654,-3.57476675253502));
#49978=CARTESIAN_POINT('',(3.67199242350841,-35.5050278513059,-3.06145306063948));
#49979=CARTESIAN_POINT('Ctrl Pts',(3.67199241167966,-35.5050281562424,-3.06145308005705));
#49980=CARTESIAN_POINT('Ctrl Pts',(3.6709074577687,-35.5049566525245,-3.06191505565046));
#49981=CARTESIAN_POINT('Ctrl Pts',(3.66982199759305,-35.5048835280257,-3.06238484334962));
#49982=CARTESIAN_POINT('Ctrl Pts',(3.66873907853604,-35.50480884055,-3.06286118186356));
#49983=CARTESIAN_POINT('Ctrl Pts',(3.66289150728548,-35.5044055413997,-3.06543332553541));
#49984=CARTESIAN_POINT('Ctrl Pts',(3.65709238413361,-35.5039531995699,-3.06820792066641));
#49985=CARTESIAN_POINT('Ctrl Pts',(3.65138326543097,-35.5034460774675,-3.07116933797591));
#49986=CARTESIAN_POINT('Ctrl Pts',(3.64385317118268,-35.5027772041395,-3.07507532637981));
#49987=CARTESIAN_POINT('Ctrl Pts',(3.63648014365973,-35.502013095345,-3.07930633742901));
#49988=CARTESIAN_POINT('Ctrl Pts',(3.62931742279077,-35.501179385654,-3.08383070640602));
#49989=CARTESIAN_POINT('Ctrl Pts',(3.62044924431927,-35.5001471680835,-3.08943233633033));
#49990=CARTESIAN_POINT('Ctrl Pts',(3.61190059299212,-35.4990131921254,-3.09548294507778));
#49991=CARTESIAN_POINT('Ctrl Pts',(3.60370943709272,-35.4978391465399,-3.10194452884521));
#49992=CARTESIAN_POINT('Ctrl Pts',(3.60239376448108,-35.4976505700263,-3.10298239564875));
#49993=CARTESIAN_POINT('Ctrl Pts',(3.60108727881218,-35.4974608692547,-3.10403091641481));
#49994=CARTESIAN_POINT('Ctrl Pts',(3.59979013424323,-35.4972701540212,-3.10508999234876));
#49995=CARTESIAN_POINT('Ctrl Pts',(3.59307320703001,-35.4962825845759,-3.11057414279112));
#49996=CARTESIAN_POINT('Ctrl Pts',(3.58660464543982,-35.4952699607466,-3.11634152422183));
#49997=CARTESIAN_POINT('Ctrl Pts',(3.58038951136343,-35.4942505186859,-3.12238406331074));
#49998=CARTESIAN_POINT('Ctrl Pts',(3.57282468603545,-35.4930096924983,-3.12973881257009));
#49999=CARTESIAN_POINT('Ctrl Pts',(3.56563464692084,-35.4917567679128,-3.13750357265183));
#50000=CARTESIAN_POINT('Ctrl Pts',(3.5588517837043,-35.490452932207,-3.14566041031418));
#50001=CARTESIAN_POINT('Ctrl Pts',(3.55802545675573,-35.4902940915308,-3.14665412263896));
#50002=CARTESIAN_POINT('Ctrl Pts',(3.55720520361751,-35.4901344532814,-3.14765361987113));
#50003=CARTESIAN_POINT('Ctrl Pts',(3.55639110831416,-35.4899739242682,-3.14865883467));
#50004=CARTESIAN_POINT('Ctrl Pts',(3.55057178146724,-35.4888264286467,-3.15584432443014));
#50005=CARTESIAN_POINT('Ctrl Pts',(3.54506529823488,-35.4876301819156,-3.1633259113768));
#50006=CARTESIAN_POINT('Ctrl Pts',(3.53991036414267,-35.4863565833647,-3.17105947667676));
#50007=CARTESIAN_POINT('Ctrl Pts',(3.53549626013491,-35.4852660172455,-3.17768162954511));
#50008=CARTESIAN_POINT('Ctrl Pts',(3.53134016454137,-35.4841178588891,-3.18448858769416));
#50009=CARTESIAN_POINT('Ctrl Pts',(3.52747469739242,-35.4829203077151,-3.19142278851816));
#50010=CARTESIAN_POINT('Ctrl Pts',(3.5261396778866,-35.4825067085007,-3.19381765904754));
#50011=CARTESIAN_POINT('Ctrl Pts',(3.52483939140283,-35.4820875246346,-3.19622741344477));
#50012=CARTESIAN_POINT('Ctrl Pts',(3.5235753914424,-35.481664210634,-3.1986486709718));
#50013=CARTESIAN_POINT('Ctrl Pts',(3.52327750749173,-35.4815644492014,-3.19921928313977));
#50014=CARTESIAN_POINT('Ctrl Pts',(3.52298214216414,-35.4814641936595,-3.19978955303356));
#50015=CARTESIAN_POINT('Ctrl Pts',(3.5226878028,-35.4813642944,-3.200362378));
#50016=CARTESIAN_POINT('Ctrl Pts',(3.67755401867,-35.5065774118,-3.05915055738));
#50017=CARTESIAN_POINT('Ctrl Pts',(3.67567292389694,-35.5056650882282,-3.05990732050017));
#50018=CARTESIAN_POINT('Ctrl Pts',(3.67381662092036,-35.5051480133643,-3.06067630953423));
#50019=CARTESIAN_POINT('Ctrl Pts',(3.67199243004608,-35.5050275473134,-3.06145302884574));
#50020=CARTESIAN_POINT('Origin',(-1.81727342606,-36.1242356128,-5.3088808072));
#50021=CARTESIAN_POINT('',(-1.68475791584498,-35.4771141120081,-5.0397346703217));
#50022=CARTESIAN_POINT('',(-1.68475792039,-36.1242356128,-5.03973467448));
#50023=CARTESIAN_POINT('',(-1.67696448377282,-35.4768981244436,-5.04371406606362));
#50024=CARTESIAN_POINT('Origin',(-1.6862492552706,-35.5734099629681,-5.04271729832598));
#50025=CARTESIAN_POINT('',(-1.51727373422622,-35.5445458978274,-5.30855096294675));
#50026=CARTESIAN_POINT('Ctrl Pts',(-1.67696448332951,-35.4768981249,-5.04371406628026));
#50027=CARTESIAN_POINT('Ctrl Pts',(-1.66756289682901,-35.4812014304152,
-5.04868876654869));
#50028=CARTESIAN_POINT('Ctrl Pts',(-1.65865341395941,-35.4852624079317,
-5.05404323411107));
#50029=CARTESIAN_POINT('Ctrl Pts',(-1.65022740097744,-35.4891142229921,
-5.05969253075887));
#50030=CARTESIAN_POINT('Ctrl Pts',(-1.63878500787594,-35.4943449272611,
-5.06736418675197));
#50031=CARTESIAN_POINT('Ctrl Pts',(-1.62823550640092,-35.4991871312493,
-5.07558040378508));
#50032=CARTESIAN_POINT('Ctrl Pts',(-1.61857496186333,-35.503616112498,-5.08412107360671));
#50033=CARTESIAN_POINT('Ctrl Pts',(-1.61461412195328,-35.5054320024432,
-5.08762276295316));
#50034=CARTESIAN_POINT('Ctrl Pts',(-1.61080272967728,-35.5071777837279,
-5.09117884037656));
#50035=CARTESIAN_POINT('Ctrl Pts',(-1.60714002108678,-35.5088508710531,
-5.09477352063633));
#50036=CARTESIAN_POINT('Ctrl Pts',(-1.59755275514454,-35.5132302347767,
-5.10418272007882));
#50037=CARTESIAN_POINT('Ctrl Pts',(-1.58896916888366,-35.5171365517006,
-5.11387017935044));
#50038=CARTESIAN_POINT('Ctrl Pts',(-1.58131204543875,-35.520569821731,-5.12362230218826));
#50039=CARTESIAN_POINT('Ctrl Pts',(-1.5784190059488,-35.5218669910727,-5.12730688121897));
#50040=CARTESIAN_POINT('Ctrl Pts',(-1.57579805519001,-35.523034690164,-5.13081589216099));
#50041=CARTESIAN_POINT('Ctrl Pts',(-1.57327569865429,-35.5241485245477,
-5.13434172428996));
#50042=CARTESIAN_POINT('Ctrl Pts',(-1.57079104913356,-35.5252457080857,
-5.1378148483251));
#50043=CARTESIAN_POINT('Ctrl Pts',(-1.5684020132668,-35.526290690752,-5.14130475228606));
#50044=CARTESIAN_POINT('Ctrl Pts',(-1.56597703365574,-35.5273357042058,
-5.14502335170683));
#50045=CARTESIAN_POINT('Ctrl Pts',(-1.56434809980794,-35.5280376720816,
-5.147521250013));
#50046=CARTESIAN_POINT('Ctrl Pts',(-1.56270356513962,-35.5287392753758,
-5.15012286969908));
#50047=CARTESIAN_POINT('Ctrl Pts',(-1.56101368681577,-35.5294504909325,
-5.15289878983892));
#50048=CARTESIAN_POINT('Ctrl Pts',(-1.557010778241,-35.5311351866944,-5.15947426593909));
#50049=CARTESIAN_POINT('Ctrl Pts',(-1.55321985384439,-35.5326854602331,
-5.16627227889667));
#50050=CARTESIAN_POINT('Ctrl Pts',(-1.54967548527541,-35.5340943103496,
-5.17326610846632));
#50051=CARTESIAN_POINT('Ctrl Pts',(-1.54469252990046,-35.5360749839517,
-5.18309859060448));
#50052=CARTESIAN_POINT('Ctrl Pts',(-1.54019901641157,-35.5377746196872,
-5.1933165367817));
#50053=CARTESIAN_POINT('Ctrl Pts',(-1.53626707299023,-35.5391855953774,
-5.20383985939881));
#50054=CARTESIAN_POINT('Ctrl Pts',(-1.53153200391583,-35.5408847722575,
-5.21651264080603));
#50055=CARTESIAN_POINT('Ctrl Pts',(-1.52761121680424,-35.5421688202375,
-5.22962559950965));
#50056=CARTESIAN_POINT('Ctrl Pts',(-1.52459023053592,-35.5430760811842,
-5.24305374223109));
#50057=CARTESIAN_POINT('Ctrl Pts',(-1.52222092663657,-35.5437876292376,
-5.25358518729078));
#50058=CARTESIAN_POINT('Ctrl Pts',(-1.52040370135698,-35.544270262472,-5.26431017256738));
#50059=CARTESIAN_POINT('Ctrl Pts',(-1.5191724082318,-35.5445240117425,-5.27519362838246));
#50060=CARTESIAN_POINT('Ctrl Pts',(-1.51811496284579,-35.544741933852,-5.28454043614104));
#50061=CARTESIAN_POINT('Ctrl Pts',(-1.517489253763,-35.5447918131442,-5.29400411313174));
#50062=CARTESIAN_POINT('Ctrl Pts',(-1.51732015056857,-35.5446392551355,
-5.30358506151032));
#50063=CARTESIAN_POINT('Ctrl Pts',(-1.51729234940888,-35.5446141740625,
-5.30516020310793));
#50064=CARTESIAN_POINT('Ctrl Pts',(-1.51727690525093,-35.5445835229505,
-5.30673857060276));
#50065=CARTESIAN_POINT('Ctrl Pts',(-1.51727394979,-35.5445470238,-5.30832023528));
#50066=CARTESIAN_POINT('',(-1.51727342606,-35.9593880834,-5.3088808072));
#50067=CARTESIAN_POINT('Ctrl Pts',(-3.51985615629,-36.3742356128,-3.20601908088));
#50068=CARTESIAN_POINT('Ctrl Pts',(-3.51985615629,-35.2912304609806,-3.20601908088));
#50069=CARTESIAN_POINT('Ctrl Pts',(-3.41903503516,-36.3742356128,-3.4128460691));
#50070=CARTESIAN_POINT('Ctrl Pts',(-3.41903503516,-35.2912304609806,-3.4128460691));
#50071=CARTESIAN_POINT('Ctrl Pts',(-3.30675917974,-36.3742356128,-3.60871163219));
#50072=CARTESIAN_POINT('Ctrl Pts',(-3.30675917974,-35.2912304609806,-3.60871163219));
#50073=CARTESIAN_POINT('Ctrl Pts',(-3.18302859005,-36.3742356128,-3.79361577017));
#50074=CARTESIAN_POINT('Ctrl Pts',(-3.18302859005,-35.2912304609806,-3.79361577017));
#50075=CARTESIAN_POINT('Ctrl Pts',(-2.86303108781,-36.3742356128,-4.20535597988));
#50076=CARTESIAN_POINT('Ctrl Pts',(-2.86303108781,-35.2912304609806,-4.20535597988));
#50077=CARTESIAN_POINT('Ctrl Pts',(-2.47885071991,-36.3742356128,-4.55567742084));
#50078=CARTESIAN_POINT('Ctrl Pts',(-2.47885071991,-35.2912304609806,-4.55567742084));
#50079=CARTESIAN_POINT('Ctrl Pts',(-2.23556166242,-36.3742356128,-4.73751640159));
#50080=CARTESIAN_POINT('Ctrl Pts',(-2.23556166242,-35.2912304609806,-4.73751640159));
#50081=CARTESIAN_POINT('Ctrl Pts',(-1.97086406258,-36.3742356128,-4.89886881947));
#50082=CARTESIAN_POINT('Ctrl Pts',(-1.97086406258,-35.2912304609806,-4.89886881947));
#50083=CARTESIAN_POINT('Ctrl Pts',(-1.68475792038,-36.3742356128,-5.03973467448));
#50084=CARTESIAN_POINT('Ctrl Pts',(-1.68475792038,-35.2912304609806,-5.03973467448));
#50085=CARTESIAN_POINT('',(-3.51985615281972,-35.4822398766,-3.20601907918835));
#50086=CARTESIAN_POINT('',(-3.51985615629,-36.1242356128,-3.20601908088));
#50087=CARTESIAN_POINT('Ctrl Pts',(-3.51985614934943,-35.4822398766,-3.2060190774967));
#50088=CARTESIAN_POINT('Ctrl Pts',(-3.47358259555133,-35.4902367502796,
-3.30094564082806));
#50089=CARTESIAN_POINT('Ctrl Pts',(-3.4242629704013,-35.4972659530676,-3.39340146700136));
#50090=CARTESIAN_POINT('Ctrl Pts',(-3.3718427520045,-35.503328318492,-3.48331166418977));
#50091=CARTESIAN_POINT('Ctrl Pts',(-3.31249447844996,-35.510191909156,-3.58510473452171));
#50092=CARTESIAN_POINT('Ctrl Pts',(-3.24917345130392,-35.5158169873826,
-3.68363701688898));
#50093=CARTESIAN_POINT('Ctrl Pts',(-3.18180390147332,-35.5202068551407,
-3.77885381081047));
#50094=CARTESIAN_POINT('Ctrl Pts',(-3.13358539867495,-35.5233488213748,
-3.84700346084822));
#50095=CARTESIAN_POINT('Ctrl Pts',(-3.08318941873635,-35.5258600003757,
-3.91359418324414));
#50096=CARTESIAN_POINT('Ctrl Pts',(-3.03070303605501,-35.527733093042,-3.97843169083073));
#50097=CARTESIAN_POINT('Ctrl Pts',(-2.97800189477388,-35.5296138498439,
-4.04353449413085));
#50098=CARTESIAN_POINT('Ctrl Pts',(-2.92319335516364,-35.530851377402,-4.10686950873771));
#50099=CARTESIAN_POINT('Ctrl Pts',(-2.86640625775876,-35.5314483764335,
-4.16827188132273));
#50100=CARTESIAN_POINT('Ctrl Pts',(-2.83093719259086,-35.5318212603899,
-4.20662363469999));
#50101=CARTESIAN_POINT('Ctrl Pts',(-2.7946970489135,-35.5319444556458,-4.24422206648277));
#50102=CARTESIAN_POINT('Ctrl Pts',(-2.75772481668771,-35.5318203627783,
-4.28103375340558));
#50103=CARTESIAN_POINT('Ctrl Pts',(-2.67048928304337,-35.531527567162,-4.36789048235417));
#50104=CARTESIAN_POINT('Ctrl Pts',(-2.57940688791399,-35.5298512045927,
-4.45014995560896));
#50105=CARTESIAN_POINT('Ctrl Pts',(-2.48455366341829,-35.5268238896998,
-4.52797607796499));
#50106=CARTESIAN_POINT('Ctrl Pts',(-2.39693745208812,-35.5240275497458,
-4.59986430337437));
#50107=CARTESIAN_POINT('Ctrl Pts',(-2.30610083339999,-35.5200781360858,
-4.66796989091402));
#50108=CARTESIAN_POINT('Ctrl Pts',(-2.21210582445137,-35.5149804585593,
-4.7323874423026));
#50109=CARTESIAN_POINT('Ctrl Pts',(-2.12903950494902,-35.5104754820199,
-4.78931524054483));
#50110=CARTESIAN_POINT('Ctrl Pts',(-2.04350466714415,-35.5050732914157,
-4.84336174171714));
#50111=CARTESIAN_POINT('Ctrl Pts',(-1.95557759183873,-35.4987661218997,
-4.89457253052966));
#50112=CARTESIAN_POINT('Ctrl Pts',(-1.87970413987643,-35.4933235807754,
-4.93876300668755));
#50113=CARTESIAN_POINT('Ctrl Pts',(-1.80204873908433,-35.487206903096,-4.98084109124512));
#50114=CARTESIAN_POINT('Ctrl Pts',(-1.72270160875273,-35.4804067652161,
-5.02083270682539));
#50115=CARTESIAN_POINT('Ctrl Pts',(-1.71009614007247,-35.4793264624413,
-5.02718596819179));
#50116=CARTESIAN_POINT('Ctrl Pts',(-1.69744808216162,-35.4782289048639,
-5.03348657861682));
#50117=CARTESIAN_POINT('Ctrl Pts',(-1.68475792683372,-35.4771140496188,
-5.03973465570198));
#50118=CARTESIAN_POINT('Origin',(-3.78952269078,-36.1242356128,-3.33747234321));
#50119=CARTESIAN_POINT('',(-3.67755401867,-35.5065774118,-3.05915055738));
#50120=CARTESIAN_POINT('',(-3.67755401867,-36.1242356128,-3.05915055738));
#50121=CARTESIAN_POINT('',(-3.67199242351697,-35.5050278513065,-3.06145306063582));
#50122=CARTESIAN_POINT('Ctrl Pts',(-3.67755401867,-35.5065774118,-3.05915055738));
#50123=CARTESIAN_POINT('Ctrl Pts',(-3.67567292389988,-35.5056650882297,
-3.05990732049898));
#50124=CARTESIAN_POINT('Ctrl Pts',(-3.67381662092617,-35.5051480133659,
-3.06067630953182));
#50125=CARTESIAN_POINT('Ctrl Pts',(-3.67199243005465,-35.505027547314,-3.06145302884209));
#50126=CARTESIAN_POINT('',(-3.52268743213354,-35.4813642832762,-3.20036310945193));
#50127=CARTESIAN_POINT('Ctrl Pts',(-3.67199241168822,-35.5050281562429,
-3.0614530800534));
#50128=CARTESIAN_POINT('Ctrl Pts',(-3.67090745777441,-35.5049566525248,
-3.06191505564798));
#50129=CARTESIAN_POINT('Ctrl Pts',(-3.6698219975959,-35.5048835280259,-3.06238484334836));
#50130=CARTESIAN_POINT('Ctrl Pts',(-3.66873907853603,-35.50480884055,-3.06286118186355));
#50131=CARTESIAN_POINT('Ctrl Pts',(-3.66289150728548,-35.5044055413997,
-3.06543332553541));
#50132=CARTESIAN_POINT('Ctrl Pts',(-3.65709238413361,-35.5039531995698,
-3.06820792066641));
#50133=CARTESIAN_POINT('Ctrl Pts',(-3.65138326543097,-35.5034460774675,
-3.0711693379759));
#50134=CARTESIAN_POINT('Ctrl Pts',(-3.64385317118269,-35.5027772041395,
-3.0750753263798));
#50135=CARTESIAN_POINT('Ctrl Pts',(-3.63648014365975,-35.502013095345,-3.079306337429));
#50136=CARTESIAN_POINT('Ctrl Pts',(-3.6293174227908,-35.501179385654,-3.083830706406));
#50137=CARTESIAN_POINT('Ctrl Pts',(-3.62044924431911,-35.5001471680835,
-3.08943233633042));
#50138=CARTESIAN_POINT('Ctrl Pts',(-3.6119005929918,-35.4990131921253,-3.09548294507801));
#50139=CARTESIAN_POINT('Ctrl Pts',(-3.60370943709224,-35.4978391465398,
-3.10194452884559));
#50140=CARTESIAN_POINT('Ctrl Pts',(-3.60239376448076,-35.4976505700263,
-3.10298239564901));
#50141=CARTESIAN_POINT('Ctrl Pts',(-3.60108727881202,-35.4974608692547,
-3.10403091641494));
#50142=CARTESIAN_POINT('Ctrl Pts',(-3.59979013424323,-35.4972701540212,
-3.10508999234876));
#50143=CARTESIAN_POINT('Ctrl Pts',(-3.59307320703006,-35.4962825845759,
-3.11057414279108));
#50144=CARTESIAN_POINT('Ctrl Pts',(-3.58660464543991,-35.4952699607466,
-3.11634152422175));
#50145=CARTESIAN_POINT('Ctrl Pts',(-3.58038951136356,-35.4942505186859,
-3.12238406331061));
#50146=CARTESIAN_POINT('Ctrl Pts',(-3.57282468603562,-35.4930096924983,
-3.12973881256992));
#50147=CARTESIAN_POINT('Ctrl Pts',(-3.56563464692104,-35.4917567679128,
-3.13750357265161));
#50148=CARTESIAN_POINT('Ctrl Pts',(-3.55885178370453,-35.4904529322071,
-3.14566041031391));
#50149=CARTESIAN_POINT('Ctrl Pts',(-3.55802545675588,-35.4902940915308,
-3.14665412263877));
#50150=CARTESIAN_POINT('Ctrl Pts',(-3.55720520361759,-35.4901344532814,
-3.14765361987103));
#50151=CARTESIAN_POINT('Ctrl Pts',(-3.55639110831416,-35.4899739242682,
-3.14865883467));
#50152=CARTESIAN_POINT('Ctrl Pts',(-3.55057178146725,-35.4888264286467,
-3.15584432443014));
#50153=CARTESIAN_POINT('Ctrl Pts',(-3.54506529823488,-35.4876301819156,
-3.16332591137679));
#50154=CARTESIAN_POINT('Ctrl Pts',(-3.53991036414268,-35.4863565833647,
-3.17105947667675));
#50155=CARTESIAN_POINT('Ctrl Pts',(-3.53549626013493,-35.4852660172455,
-3.17768162954508));
#50156=CARTESIAN_POINT('Ctrl Pts',(-3.53134016454139,-35.4841178588891,
-3.18448858769411));
#50157=CARTESIAN_POINT('Ctrl Pts',(-3.52747469739246,-35.4829203077152,
-3.1914227885181));
#50158=CARTESIAN_POINT('Ctrl Pts',(-3.52613967788663,-35.4825067085007,
-3.1938176590475));
#50159=CARTESIAN_POINT('Ctrl Pts',(-3.52483939140284,-35.4820875246346,
-3.19622741344476));
#50160=CARTESIAN_POINT('Ctrl Pts',(-3.5235753914424,-35.481664210634,-3.1986486709718));
#50161=CARTESIAN_POINT('Ctrl Pts',(-3.52327750749173,-35.4815644492014,
-3.19921928313977));
#50162=CARTESIAN_POINT('Ctrl Pts',(-3.52298214216414,-35.4814641936595,
-3.19978955303356));
#50163=CARTESIAN_POINT('Ctrl Pts',(-3.5226878028,-35.4813642944,-3.200362378));
#50164=CARTESIAN_POINT('Origin',(-3.61904102711591,-42.5155158381654,-3.57476675253502));
#50165=CARTESIAN_POINT('Ctrl Pts',(-7.07911993306,-36.3742356128,1.41233341424));
#50166=CARTESIAN_POINT('Ctrl Pts',(-7.07911993306,-35.17422421556,1.41233341424));
#50167=CARTESIAN_POINT('Ctrl Pts',(-7.02062825816,-36.3742356128,0.811131443794));
#50168=CARTESIAN_POINT('Ctrl Pts',(-7.02062825816,-35.17422421556,0.811131443794));
#50169=CARTESIAN_POINT('Ctrl Pts',(-6.90206842567,-36.3742356128,0.252977206386));
#50170=CARTESIAN_POINT('Ctrl Pts',(-6.90206842567,-35.17422421556,0.252977206386));
#50171=CARTESIAN_POINT('Ctrl Pts',(-6.72344043556,-36.3742356128,-0.262129297982999));
#50172=CARTESIAN_POINT('Ctrl Pts',(-6.72344043556,-35.17422421556,-0.262129297983));
#50173=CARTESIAN_POINT('Ctrl Pts',(-6.21056508527,-36.3742356128,-1.27642010253));
#50174=CARTESIAN_POINT('Ctrl Pts',(-6.21056508527,-35.17422421556,-1.27642010253));
#50175=CARTESIAN_POINT('Ctrl Pts',(-5.42037231907,-36.3742356128,-2.09197189854));
#50176=CARTESIAN_POINT('Ctrl Pts',(-5.42037231907,-35.17422421556,-2.09197189854));
#50177=CARTESIAN_POINT('Ctrl Pts',(-4.91868712629,-36.3742356128,-2.4711621885));
#50178=CARTESIAN_POINT('Ctrl Pts',(-4.91868712629,-35.17422421556,-2.4711621885));
#50179=CARTESIAN_POINT('Ctrl Pts',(-4.33774769283,-36.3742356128,-2.79355507478));
#50180=CARTESIAN_POINT('Ctrl Pts',(-4.33774769283,-35.17422421556,-2.79355507478));
#50181=CARTESIAN_POINT('Ctrl Pts',(-3.67755401866,-36.3742356128,-3.05915055738));
#50182=CARTESIAN_POINT('Ctrl Pts',(-3.67755401866,-35.17422421556,-3.05915055738));
#50183=CARTESIAN_POINT('',(-7.07911993306,-35.3742356128,1.41233341424));
#50184=CARTESIAN_POINT('',(-7.07911993306,-36.1242356128,1.41233341424));
#50185=CARTESIAN_POINT('',(-7.05021189233511,-35.3742261184909,1.16209533463037));
#50186=CARTESIAN_POINT('Ctrl Pts',(-7.05021164825251,-35.3742261150622,
1.16209544641768));
#50187=CARTESIAN_POINT('Ctrl Pts',(-7.05298995234368,-35.3742266401801,
1.18279723135034));
#50188=CARTESIAN_POINT('Ctrl Pts',(-7.05571064340917,-35.3742477797272,
1.20381716458915));
#50189=CARTESIAN_POINT('Ctrl Pts',(-7.05829605327761,-35.3742431701945,
1.22454392284656));
#50190=CARTESIAN_POINT('Ctrl Pts',(-7.0608927559198,-35.3742385405278,1.24536121320659));
#50191=CARTESIAN_POINT('Ctrl Pts',(-7.06339480482366,-35.3742375427218,
1.26620204691466));
#50192=CARTESIAN_POINT('Ctrl Pts',(-7.06580506972233,-35.3742369799112,
1.28708281574342));
#50193=CARTESIAN_POINT('Ctrl Pts',(-7.07061980686756,-35.3742358556427,
1.32879417010789));
#50194=CARTESIAN_POINT('Ctrl Pts',(-7.07505478224174,-35.3742356535494,
1.37055008889881));
#50195=CARTESIAN_POINT('Ctrl Pts',(-7.07911993306,-35.3742356128,1.41233341424));
#50196=CARTESIAN_POINT('Ctrl Pts',(-7.05021188141398,-35.3742261390046,
1.1620952532504));
#50197=CARTESIAN_POINT('Ctrl Pts',(-7.04352707146932,-35.381715700076,1.11228520069688));
#50198=CARTESIAN_POINT('Ctrl Pts',(-7.03635023271754,-35.3890407899385,
1.06303551389404));
#50199=CARTESIAN_POINT('Ctrl Pts',(-7.02867908891517,-35.3961811568166,
1.01427777377839));
#50200=CARTESIAN_POINT('Ctrl Pts',(-7.01997402407047,-35.404283906327,0.958948438242224));
#50201=CARTESIAN_POINT('Ctrl Pts',(-7.01063229140259,-35.4121485106884,
0.904253034225137));
#50202=CARTESIAN_POINT('Ctrl Pts',(-7.00066015753755,-35.4197633417748,
0.850158125696098));
#50203=CARTESIAN_POINT('Ctrl Pts',(-6.98968258670088,-35.4281459355899,
0.790609116595527));
#50204=CARTESIAN_POINT('Ctrl Pts',(-6.97794100473584,-35.4362257116211,
0.731789102718959));
#50205=CARTESIAN_POINT('Ctrl Pts',(-6.96545655070105,-35.4440111016219,
0.673714193997119));
#50206=CARTESIAN_POINT('Ctrl Pts',(-6.95155204539388,-35.4526820452036,
0.609033521996102));
#50207=CARTESIAN_POINT('Ctrl Pts',(-6.93672600539964,-35.4609877333797,
0.545278981739372));
#50208=CARTESIAN_POINT('Ctrl Pts',(-6.92102403957521,-35.4689702606657,
0.482517887121766));
#50209=CARTESIAN_POINT('Ctrl Pts',(-6.89588675441965,-35.4817494926992,
0.382043618503607));
#50210=CARTESIAN_POINT('Ctrl Pts',(-6.86846319411156,-35.4936186298441,
0.283938115251837));
#50211=CARTESIAN_POINT('Ctrl Pts',(-6.83883729901714,-35.5045777234444,
0.188140683587292));
#50212=CARTESIAN_POINT('Ctrl Pts',(-6.83670483057942,-35.5053665577103,
0.181245195745052));
#50213=CARTESIAN_POINT('Ctrl Pts',(-6.83456094047648,-35.5061506762736,
0.174361641847689));
#50214=CARTESIAN_POINT('Ctrl Pts',(-6.83240565405016,-35.5069300791112,
0.167489984676289));
#50215=CARTESIAN_POINT('Ctrl Pts',(-6.81635656074776,-35.5127338129942,
0.116320977281485));
#50216=CARTESIAN_POINT('Ctrl Pts',(-6.7996760330039,-35.518276096045,0.0658134591906613));
#50217=CARTESIAN_POINT('Ctrl Pts',(-6.78237703513777,-35.5235569279985,
0.0159579638384577));
#50218=CARTESIAN_POINT('Ctrl Pts',(-6.7737275362047,-35.5261973439752,-0.00896978383764373));
#50219=CARTESIAN_POINT('Ctrl Pts',(-6.76492343663421,-35.5287723971648,
-0.0337345291900959));
#50220=CARTESIAN_POINT('Ctrl Pts',(-6.75596652857811,-35.5312820875257,
-0.0583375110691009));
#50221=CARTESIAN_POINT('Ctrl Pts',(-6.75148807455006,-35.5325369327061,
-0.0706390020086038));
#50222=CARTESIAN_POINT('Ctrl Pts',(-6.74697142075146,-35.5337754371799,
-0.0829000529775413));
#50223=CARTESIAN_POINT('Ctrl Pts',(-6.74241680762996,-35.5349976009461,
-0.0951208255204967));
#50224=CARTESIAN_POINT('Ctrl Pts',(-6.73891429679059,-35.5359374484643,
-0.104518635423402));
#50225=CARTESIAN_POINT('Ctrl Pts',(-6.73570406504125,-35.5367853631935,
-0.113059445497894));
#50226=CARTESIAN_POINT('Ctrl Pts',(-6.73206100729518,-35.537731318041,-0.122665614285448));
#50227=CARTESIAN_POINT('Ctrl Pts',(-6.73096668680786,-35.5380154688401,
-0.125551164842593));
#50228=CARTESIAN_POINT('Ctrl Pts',(-6.72983298604664,-35.538308389363,-0.128532797850881));
#50229=CARTESIAN_POINT('Ctrl Pts',(-6.72863934124971,-35.538615014252,-0.131662481145629));
#50230=CARTESIAN_POINT('Ctrl Pts',(-6.7245761357129,-35.539658775302,-0.14231602441441));
#50231=CARTESIAN_POINT('Ctrl Pts',(-6.72047624723707,-35.5406929458301,
-0.152958731118445));
#50232=CARTESIAN_POINT('Ctrl Pts',(-6.71633948303299,-35.5417175400764,
-0.163590489490864));
#50233=CARTESIAN_POINT('Ctrl Pts',(-6.67755929772736,-35.5513226209492,
-0.263258137794542));
#50234=CARTESIAN_POINT('Ctrl Pts',(-6.63553882391724,-35.5600852051321,
-0.361959218829963));
#50235=CARTESIAN_POINT('Ctrl Pts',(-6.59009883490075,-35.5680052181569,
-0.459541970726329));
#50236=CARTESIAN_POINT('Ctrl Pts',(-6.54175602567053,-35.5764311814338,
-0.563358553018467));
#50237=CARTESIAN_POINT('Ctrl Pts',(-6.48954401475643,-35.5839042846034,
-0.665911252177743));
#50238=CARTESIAN_POINT('Ctrl Pts',(-6.43323009460924,-35.5904302877287,
-0.767062608930708));
#50239=CARTESIAN_POINT('Ctrl Pts',(-6.35567379192739,-35.5994179886802,
-0.906369643861105));
#50240=CARTESIAN_POINT('Ctrl Pts',(-6.2703500558032,-35.6066100934343,-1.04299798700632));
#50241=CARTESIAN_POINT('Ctrl Pts',(-6.17666402058228,-35.6119997299894,
-1.17652254193963));
#50242=CARTESIAN_POINT('Ctrl Pts',(-6.16625937752191,-35.6125982956609,
-1.19135159656446));
#50243=CARTESIAN_POINT('Ctrl Pts',(-6.15575156510111,-35.6131745884083,
-1.20614235116042));
#50244=CARTESIAN_POINT('Ctrl Pts',(-6.14513974492393,-35.6137285633824,
-1.22089421231661));
#50245=CARTESIAN_POINT('Ctrl Pts',(-6.12744585650583,-35.6146522476527,
-1.24549110341529));
#50246=CARTESIAN_POINT('Ctrl Pts',(-6.10918547518569,-35.6155271446915,
-1.27035748958776));
#50247=CARTESIAN_POINT('Ctrl Pts',(-6.09076485774616,-35.6163316064952,
-1.29492033009841));
#50248=CARTESIAN_POINT('Ctrl Pts',(-6.07234424030663,-35.6171360682989,
-1.31948317060907));
#50249=CARTESIAN_POINT('Ctrl Pts',(-6.05376357297037,-35.6178701284919,
-1.34374234998056));
#50250=CARTESIAN_POINT('Ctrl Pts',(-6.03547539301575,-35.6185238313854,
-1.3671556564777));
#50251=CARTESIAN_POINT('Ctrl Pts',(-5.96003196187137,-35.6212205234211,
-1.46374154862018));
#50252=CARTESIAN_POINT('Ctrl Pts',(-5.8806430282633,-35.6228887681904,-1.55747864373515));
#50253=CARTESIAN_POINT('Ctrl Pts',(-5.79732811347347,-35.6235530383653,
-1.64835399093985));
#50254=CARTESIAN_POINT('Ctrl Pts',(-5.71907262973099,-35.6241769696747,
-1.7337107877836));
#50255=CARTESIAN_POINT('Ctrl Pts',(-5.63735326506376,-35.6239144984006,
-1.81654508341693));
#50256=CARTESIAN_POINT('Ctrl Pts',(-5.55216217707629,-35.6227748437847,
-1.89687171823991));
#50257=CARTESIAN_POINT('Ctrl Pts',(-5.43288206744175,-35.6211791589456,
-2.00934087475155));
#50258=CARTESIAN_POINT('Ctrl Pts',(-5.30680750719591,-35.6178655165706,
-2.11688217438336));
#50259=CARTESIAN_POINT('Ctrl Pts',(-5.17395137625618,-35.6128041649775,
-2.21950506889937));
#50260=CARTESIAN_POINT('Ctrl Pts',(-5.13538698860863,-35.6113349973638,
-2.24929360073177));
#50261=CARTESIAN_POINT('Ctrl Pts',(-5.09625123076711,-35.609718224167,-2.27866769919633));
#50262=CARTESIAN_POINT('Ctrl Pts',(-5.05654447604708,-35.6079523441408,
-2.30762755684394));
#50263=CARTESIAN_POINT('Ctrl Pts',(-5.04054291620784,-35.6072407061561,
-2.31929818815974));
#50264=CARTESIAN_POINT('Ctrl Pts',(-5.02394560548748,-35.6064813720674,
-2.33126302911098));
#50265=CARTESIAN_POINT('Ctrl Pts',(-5.00770854202776,-35.6057181156694,
-2.34283175821588));
#50266=CARTESIAN_POINT('Ctrl Pts',(-4.9983604602823,-35.6052786899556,-2.34949216362922));
#50267=CARTESIAN_POINT('Ctrl Pts',(-4.98913243268586,-35.6048381769909,
-2.35602204061313));
#50268=CARTESIAN_POINT('Ctrl Pts',(-4.98021172600241,-35.6044065601333,
-2.36229557116517));
#50269=CARTESIAN_POINT('Ctrl Pts',(-4.83811928258686,-35.5975316009961,
-2.46222277610684));
#50270=CARTESIAN_POINT('Ctrl Pts',(-4.6899512138041,-35.5888504066531,-2.55634922532136));
#50271=CARTESIAN_POINT('Ctrl Pts',(-4.53605954555446,-35.5783538872027,
-2.64486936122386));
#50272=CARTESIAN_POINT('Ctrl Pts',(-4.40146233214111,-35.5691733884491,
-2.72229112004266));
#50273=CARTESIAN_POINT('Ctrl Pts',(-4.2624871398174,-35.558602765964,-2.79542528542047));
#50274=CARTESIAN_POINT('Ctrl Pts',(-4.11934100470481,-35.5466380561341,
-2.86442049917059));
#50275=CARTESIAN_POINT('Ctrl Pts',(-3.99031460571353,-35.5358535286782,
-2.92661012078217));
#50276=CARTESIAN_POINT('Ctrl Pts',(-3.85790038353982,-35.5239354720522,
-2.98543736793842));
#50277=CARTESIAN_POINT('Ctrl Pts',(-3.7222163946605,-35.5108977782426,-3.04101944174927));
#50278=CARTESIAN_POINT('Ctrl Pts',(-3.70736809901062,-35.5094710252861,
-3.04710195061117));
#50279=CARTESIAN_POINT('Ctrl Pts',(-3.6924806009018,-35.5080308900275,-3.0531456031268));
#50280=CARTESIAN_POINT('Ctrl Pts',(-3.67755401867,-35.5065774118,-3.05915055738));
#50281=CARTESIAN_POINT('Ctrl Pts',(-7.21384189759,-36.3742356128,2.18958432614));
#50282=CARTESIAN_POINT('Ctrl Pts',(-7.21384189759,-35.1742356128,2.18958432614));
#50283=CARTESIAN_POINT('Ctrl Pts',(-7.13908599018,-36.3742356128,2.05065155888));
#50284=CARTESIAN_POINT('Ctrl Pts',(-7.13908599018,-35.1742356128,2.05065155888));
#50285=CARTESIAN_POINT('Ctrl Pts',(-7.08904524264,-36.3742356128,1.89842024269));
#50286=CARTESIAN_POINT('Ctrl Pts',(-7.08904524264,-35.1742356128,1.89842024269));
#50287=CARTESIAN_POINT('Ctrl Pts',(-7.10533215541,-36.3742356128,1.72680915639));
#50288=CARTESIAN_POINT('Ctrl Pts',(-7.10533215541,-35.1742356128,1.72680915639));
#50289=CARTESIAN_POINT('Ctrl Pts',(-7.09439724612,-36.3742356128,1.56936004643));
#50290=CARTESIAN_POINT('Ctrl Pts',(-7.09439724612,-35.1742356128,1.56936004643));
#50291=CARTESIAN_POINT('Ctrl Pts',(-7.07911993306,-36.3742356128,1.41233341424));
#50292=CARTESIAN_POINT('Ctrl Pts',(-7.07911993306,-35.1742356128,1.41233341424));
#50293=CARTESIAN_POINT('',(-7.21384189758587,-35.4651148398172,2.18958432618295));
#50294=CARTESIAN_POINT('',(-7.21384189758,-36.1242356128,2.18958432614));
#50295=CARTESIAN_POINT('',(-7.13973478936,-35.3742392475,2.00655473738));
#50296=CARTESIAN_POINT('Ctrl Pts',(-7.21384189753719,-35.4651148399882,
2.18958432613386));
#50297=CARTESIAN_POINT('Ctrl Pts',(-7.20248970613278,-35.4558376974756,
2.16852385251479));
#50298=CARTESIAN_POINT('Ctrl Pts',(-7.19216154693066,-35.4455454559845,
2.14764262491228));
#50299=CARTESIAN_POINT('Ctrl Pts',(-7.18277070551959,-35.4348282932108,
2.12663643240788));
#50300=CARTESIAN_POINT('Ctrl Pts',(-7.17770336699823,-35.4290452659627,
2.11530140034788));
#50301=CARTESIAN_POINT('Ctrl Pts',(-7.17290922444295,-35.4231375971478,
2.10393011825159));
#50302=CARTESIAN_POINT('Ctrl Pts',(-7.16837646591434,-35.4171920851989,
2.09247569166461));
#50303=CARTESIAN_POINT('Ctrl Pts',(-7.15869260576572,-35.404489995321,2.06800426561123));
#50304=CARTESIAN_POINT('Ctrl Pts',(-7.15020429789435,-35.3915941161304,
2.04315346963811));
#50305=CARTESIAN_POINT('Ctrl Pts',(-7.14282824899172,-35.3794131715241,
2.01756660856243));
#50306=CARTESIAN_POINT('Ctrl Pts',(-7.14201563347066,-35.37807120311,2.01474771721293));
#50307=CARTESIAN_POINT('Ctrl Pts',(-7.14121690146011,-35.376735446728,2.01192135159036));
#50308=CARTESIAN_POINT('Ctrl Pts',(-7.1404309617392,-35.3754137600701,2.0090835975648));
#50309=CARTESIAN_POINT('Ctrl Pts',(-7.1401977511474,-35.375021578177,2.00824155551238));
#50310=CARTESIAN_POINT('Ctrl Pts',(-7.13996568730528,-35.3746302925694,
2.00739857926709));
#50311=CARTESIAN_POINT('Ctrl Pts',(-7.13973478936,-35.3742392475,2.00655473738));
#50312=CARTESIAN_POINT('Ctrl Pts',(-7.07911993306,-35.3742356128,1.41233341424));
#50313=CARTESIAN_POINT('Ctrl Pts',(-7.08088379359945,-35.3742356128,1.43046208289635));
#50314=CARTESIAN_POINT('Ctrl Pts',(-7.08257391393288,-35.3742355920726,
1.44859911701878));
#50315=CARTESIAN_POINT('Ctrl Pts',(-7.08413990039285,-35.3742355563689,
1.46677978317039));
#50316=CARTESIAN_POINT('Ctrl Pts',(-7.08577195894419,-35.3742355191587,
1.4857275278798));
#50317=CARTESIAN_POINT('Ctrl Pts',(-7.08726945163803,-35.3742354656818,
1.5047225982671));
#50318=CARTESIAN_POINT('Ctrl Pts',(-7.0886278899404,-35.3742354024484,1.52378297170902));
#50319=CARTESIAN_POINT('Ctrl Pts',(-7.09010880652101,-35.3742353335138,
1.54456184919918));
#50320=CARTESIAN_POINT('Ctrl Pts',(-7.09142454145993,-35.3742352529839,
1.56541838105054));
#50321=CARTESIAN_POINT('Ctrl Pts',(-7.09262835646224,-35.3742351692935,
1.58635022088169));
#50322=CARTESIAN_POINT('Ctrl Pts',(-7.09392979130774,-35.3742350788165,
1.60897946680765));
#50323=CARTESIAN_POINT('Ctrl Pts',(-7.0951009883527,-35.3742349846456,1.63169662188994));
#50324=CARTESIAN_POINT('Ctrl Pts',(-7.09627031081483,-35.3742348974381,
1.6544704621937));
#50325=CARTESIAN_POINT('Ctrl Pts',(-7.09759721920297,-35.3742347984779,
1.68031346162976));
#50326=CARTESIAN_POINT('Ctrl Pts',(-7.09892280102883,-35.3742347084847,
1.70622930734005));
#50327=CARTESIAN_POINT('Ctrl Pts',(-7.10049797330169,-35.3742346430313,
1.73213889512276));
#50328=CARTESIAN_POINT('Ctrl Pts',(-7.10268355309506,-35.3742345522136,
1.76808891309122));
#50329=CARTESIAN_POINT('Ctrl Pts',(-7.10535563162135,-35.3742345086403,
1.80402663897013));
#50330=CARTESIAN_POINT('Ctrl Pts',(-7.10925382044981,-35.374234553911,1.8396775575811));
#50331=CARTESIAN_POINT('Ctrl Pts',(-7.11201818443917,-35.3742345860143,
1.86495907162076));
#50332=CARTESIAN_POINT('Ctrl Pts',(-7.1154016075227,-35.3742346627955,1.890094551153));
#50333=CARTESIAN_POINT('Ctrl Pts',(-7.11963758304941,-35.3742347990895,
1.91498267217685));
#50334=CARTESIAN_POINT('Ctrl Pts',(-7.12328042918288,-35.3742349162994,
1.93638591090411));
#50335=CARTESIAN_POINT('Ctrl Pts',(-7.12755425624875,-35.3742350775228,
1.95760586665248));
#50336=CARTESIAN_POINT('Ctrl Pts',(-7.13256782595468,-35.3742352921948,
1.97858502103487));
#50337=CARTESIAN_POINT('Ctrl Pts',(-7.13480768313778,-35.3742353881014,
1.98795764620913));
#50338=CARTESIAN_POINT('Ctrl Pts',(-7.13719457595265,-35.3742354946761,
1.99728233675654));
#50339=CARTESIAN_POINT('Ctrl Pts',(-7.13973478937384,-35.37423561276,2.00655473739936));
#50340=CARTESIAN_POINT('Ctrl Pts',(-8.75956299024,-36.3742356128,2.0634404101));
#50341=CARTESIAN_POINT('Ctrl Pts',(-8.75956299024,-35.2767450158758,2.0634404101));
#50342=CARTESIAN_POINT('Ctrl Pts',(-8.72637376563,-36.3742356128,2.11781888978));
#50343=CARTESIAN_POINT('Ctrl Pts',(-8.72637376563,-35.2767450158758,2.11781888978));
#50344=CARTESIAN_POINT('Ctrl Pts',(-8.6915484,-36.3742356128,2.17268982337));
#50345=CARTESIAN_POINT('Ctrl Pts',(-8.6915484,-35.2767450158758,2.17268982337));
#50346=CARTESIAN_POINT('Ctrl Pts',(-8.65506636668,-36.3742356128,2.22762960985));
#50347=CARTESIAN_POINT('Ctrl Pts',(-8.65506636668,-35.2767450158758,2.22762960985));
#50348=CARTESIAN_POINT('Ctrl Pts',(-8.53055023262,-36.3742356128,2.40503324452));
#50349=CARTESIAN_POINT('Ctrl Pts',(-8.53055023262,-35.2767450158758,2.40503324452));
#50350=CARTESIAN_POINT('Ctrl Pts',(-8.3876008666,-36.3742356128,2.56660232663));
#50351=CARTESIAN_POINT('Ctrl Pts',(-8.3876008666,-35.2767450158758,2.56660232663));
#50352=CARTESIAN_POINT('Ctrl Pts',(-8.27908544119,-36.3742356128,2.66027026629));
#50353=CARTESIAN_POINT('Ctrl Pts',(-8.27908544119,-35.2767450158758,2.66027026629));
#50354=CARTESIAN_POINT('Ctrl Pts',(-8.01327762974,-36.3742356128,2.78696551824));
#50355=CARTESIAN_POINT('Ctrl Pts',(-8.01327762974,-35.2767450158758,2.78696551824));
#50356=CARTESIAN_POINT('Ctrl Pts',(-7.71906576509,-36.3742356128,2.71717075777));
#50357=CARTESIAN_POINT('Ctrl Pts',(-7.71906576509,-35.2767450158758,2.71717075777));
#50358=CARTESIAN_POINT('Ctrl Pts',(-7.55641153588,-36.3742356128,2.61428156978));
#50359=CARTESIAN_POINT('Ctrl Pts',(-7.55641153588,-35.2767450158758,2.61428156978));
#50360=CARTESIAN_POINT('Ctrl Pts',(-7.38865661676,-36.3742356128,2.45617777771));
#50361=CARTESIAN_POINT('Ctrl Pts',(-7.38865661676,-35.2767450158758,2.45617777771));
#50362=CARTESIAN_POINT('Ctrl Pts',(-7.26550535688,-36.3742356128,2.27753774962));
#50363=CARTESIAN_POINT('Ctrl Pts',(-7.26550535688,-35.2767450158758,2.27753774962));
#50364=CARTESIAN_POINT('Ctrl Pts',(-7.24701042964,-36.3742356128,2.24853650952));
#50365=CARTESIAN_POINT('Ctrl Pts',(-7.24701042964,-35.2767450158758,2.24853650952));
#50366=CARTESIAN_POINT('Ctrl Pts',(-7.2297761181,-36.3742356128,2.21919784335));
#50367=CARTESIAN_POINT('Ctrl Pts',(-7.2297761181,-35.2767450158758,2.21919784335));
#50368=CARTESIAN_POINT('Ctrl Pts',(-7.21384189758,-36.3742356128,2.18958432613));
#50369=CARTESIAN_POINT('Ctrl Pts',(-7.21384189758,-35.2767450158758,2.18958432613));
#50370=CARTESIAN_POINT('',(-8.75956299007003,-35.6438772168026,2.06344041036242));
#50371=CARTESIAN_POINT('',(-8.75956299023,-36.1242356128,2.0634404101));
#50372=CARTESIAN_POINT('',(-8.73000675245248,-35.6496340209958,2.1111701504857));
#50373=CARTESIAN_POINT('Origin',(-8.8025233360182,-35.5994617475288,1.55277754717549));
#50374=CARTESIAN_POINT('',(-8.49626470339955,-35.699502272635,2.43550539329785));
#50375=CARTESIAN_POINT('Ctrl Pts',(-8.73000528472,-35.6496341999,2.11117245845));
#50376=CARTESIAN_POINT('Ctrl Pts',(-8.71278579373065,-35.6529734545507,
2.13857243132976));
#50377=CARTESIAN_POINT('Ctrl Pts',(-8.69523611065439,-35.656418433528,2.16578280028398));
#50378=CARTESIAN_POINT('Ctrl Pts',(-8.67736328843596,-35.6599993397373,
2.19267530487441));
#50379=CARTESIAN_POINT('Ctrl Pts',(-8.65990881423403,-35.6634964279019,
2.21893833831492));
#50380=CARTESIAN_POINT('Ctrl Pts',(-8.64214969971165,-35.6671228124049,
2.24489443760551));
#50381=CARTESIAN_POINT('Ctrl Pts',(-8.6240892075043,-35.6709094567015,2.27040574861869));
#50382=CARTESIAN_POINT('Ctrl Pts',(-8.60885152877019,-35.6741042571869,
2.29192970028301));
#50383=CARTESIAN_POINT('Ctrl Pts',(-8.59340033381773,-35.6774130775882,
2.31313561363373));
#50384=CARTESIAN_POINT('Ctrl Pts',(-8.57770836660362,-35.6808587827496,
2.33395912375569));
#50385=CARTESIAN_POINT('Ctrl Pts',(-8.57480139519109,-35.6814971072033,
2.33781672476946));
#50386=CARTESIAN_POINT('Ctrl Pts',(-8.57188604813872,-35.6821401439685,
2.3416612893117));
#50387=CARTESIAN_POINT('Ctrl Pts',(-8.56896198405368,-35.6827880598152,
2.34549254173609));
#50388=CARTESIAN_POINT('Ctrl Pts',(-8.56143090936174,-35.6844567997929,
2.35536012580152));
#50389=CARTESIAN_POINT('Ctrl Pts',(-8.55384786331649,-35.6861566070827,
2.36513232166256));
#50390=CARTESIAN_POINT('Ctrl Pts',(-8.54621303383084,-35.6878884842043,
2.37479733602594));
#50391=CARTESIAN_POINT('Ctrl Pts',(-8.53873858847129,-35.6895839799504,
2.38425931836546));
#50392=CARTESIAN_POINT('Ctrl Pts',(-8.53121142039016,-35.6913109462438,
2.39362216719067));
#50393=CARTESIAN_POINT('Ctrl Pts',(-8.52362054975123,-35.6930722906216,
2.40288673572145));
#50394=CARTESIAN_POINT('Ctrl Pts',(-8.51695920442706,-35.6946179529959,
2.41101682951418));
#50395=CARTESIAN_POINT('Ctrl Pts',(-8.51024738112154,-35.6961904182621,
2.41907287662946));
#50396=CARTESIAN_POINT('Ctrl Pts',(-8.50349797791776,-35.6977863767698,
2.42703115952841));
#50397=CARTESIAN_POINT('Ctrl Pts',(-8.50255616499077,-35.6980090771046,
2.42814165974369));
#50398=CARTESIAN_POINT('Ctrl Pts',(-8.50161367399323,-35.6982322214535,
2.42925019294274));
#50399=CARTESIAN_POINT('Ctrl Pts',(-8.50067059768458,-35.6984557864418,
2.43035662659535));
#50400=CARTESIAN_POINT('Ctrl Pts',(-8.49920411912565,-35.6988034287893,
2.43207712494054));
#50401=CARTESIAN_POINT('Ctrl Pts',(-8.49773226797996,-35.6991530223845,
2.43379716100814));
#50402=CARTESIAN_POINT('Ctrl Pts',(-8.49626469608749,-35.6995022721787,
2.43550538236112));
#50403=CARTESIAN_POINT('',(-7.23334333080301,-35.4800020975,2.22433302562685));
#50404=CARTESIAN_POINT('Ctrl Pts',(-8.49626470705517,-35.699502273,2.43550539876585));
#50405=CARTESIAN_POINT('Ctrl Pts',(-8.48478738974076,-35.7022336299315,
2.44886473885747));
#50406=CARTESIAN_POINT('Ctrl Pts',(-8.47349630523902,-35.7048385205551,
2.46159463232704));
#50407=CARTESIAN_POINT('Ctrl Pts',(-8.46237222531038,-35.707344358481,2.4737420925269));
#50408=CARTESIAN_POINT('Ctrl Pts',(-8.44944563624108,-35.7102562341012,
2.48785788702376));
#50409=CARTESIAN_POINT('Ctrl Pts',(-8.43674458927482,-35.7130334581298,
2.50118599352194));
#50410=CARTESIAN_POINT('Ctrl Pts',(-8.42428045772585,-35.7156815003471,
2.51375562733581));
#50411=CARTESIAN_POINT('Ctrl Pts',(-8.40827473989147,-35.7190819632174,
2.52989682508521));
#50412=CARTESIAN_POINT('Ctrl Pts',(-8.39265963522996,-35.7222671863208,
2.54478430272951));
#50413=CARTESIAN_POINT('Ctrl Pts',(-8.37752566693042,-35.7252176514594,
2.55844769532221));
#50414=CARTESIAN_POINT('Ctrl Pts',(-8.36221547823891,-35.7282024719047,
2.57227018487816));
#50415=CARTESIAN_POINT('Ctrl Pts',(-8.34740012240277,-35.7309447120799,
2.58483721748327));
#50416=CARTESIAN_POINT('Ctrl Pts',(-8.33320903630987,-35.7334376491566,
2.59620216330057));
#50417=CARTESIAN_POINT('Ctrl Pts',(-8.33095938864949,-35.7338328430147,
2.59800379593114));
#50418=CARTESIAN_POINT('Ctrl Pts',(-8.32872546097848,-35.7342218324706,
2.59977530309741));
#50419=CARTESIAN_POINT('Ctrl Pts',(-8.32650779509264,-35.7346046636448,
2.60151699533483));
#50420=CARTESIAN_POINT('Ctrl Pts',(-8.31036047399732,-35.7373921430097,
2.61419864588754));
#50421=CARTESIAN_POINT('Ctrl Pts',(-8.29499932423798,-35.7398659334796,
2.62535730899568));
#50422=CARTESIAN_POINT('Ctrl Pts',(-8.28052173447358,-35.742015932203,2.63519468961952));
#50423=CARTESIAN_POINT('Ctrl Pts',(-8.27333546216802,-35.7430831316841,
2.64007769135439));
#50424=CARTESIAN_POINT('Ctrl Pts',(-8.26636661759111,-35.7440712201303,
2.64463574972307));
#50425=CARTESIAN_POINT('Ctrl Pts',(-8.25962499438878,-35.7449822598253,
2.64889600990654));
#50426=CARTESIAN_POINT('Ctrl Pts',(-8.25889069886849,-35.745081489988,2.64936003613199));
#50427=CARTESIAN_POINT('Ctrl Pts',(-8.25815909729571,-35.7451798077242,
2.64982053030333));
#50428=CARTESIAN_POINT('Ctrl Pts',(-8.25743019202015,-35.7452772092317,
2.65027752888441));
#50429=CARTESIAN_POINT('Ctrl Pts',(-8.24697862589458,-35.7466738218366,
2.65683030199446));
#50430=CARTESIAN_POINT('Ctrl Pts',(-8.23708400295828,-35.747879361664,2.66266250084632));
#50431=CARTESIAN_POINT('Ctrl Pts',(-8.22777710389026,-35.74889382729,2.66786953541919));
#50432=CARTESIAN_POINT('Ctrl Pts',(-8.22312365435624,-35.7494010601031,
2.67047305270562));
#50433=CARTESIAN_POINT('Ctrl Pts',(-8.21861717004876,-35.7498605244786,
2.67292030448637));
#50434=CARTESIAN_POINT('Ctrl Pts',(-8.21426118604618,-35.750272220593,2.67522322539416));
#50435=CARTESIAN_POINT('Ctrl Pts',(-8.21208319404489,-35.7504780686502,
2.67637468584805));
#50436=CARTESIAN_POINT('Ctrl Pts',(-8.20994282504322,-35.7506719746426,
2.67749005947097));
#50437=CARTESIAN_POINT('Ctrl Pts',(-8.20784050698368,-35.7508539385916,
2.67857080521581));
#50438=CARTESIAN_POINT('Ctrl Pts',(-8.20650579572473,-35.7509694631337,
2.6792569447403));
#50439=CARTESIAN_POINT('Ctrl Pts',(-8.20582892443352,-35.7510274346216,
2.67960206025779));
#50440=CARTESIAN_POINT('Ctrl Pts',(-8.20458681491374,-35.7511290070974,
2.6802314134196));
#50441=CARTESIAN_POINT('Ctrl Pts',(-8.20387246436933,-35.7511874225207,
2.680593361192));
#50442=CARTESIAN_POINT('Ctrl Pts',(-8.20297109329813,-35.7512601548331,
2.68104909082734));
#50443=CARTESIAN_POINT('Ctrl Pts',(-8.20164809435695,-35.7513630392347,
2.68171060399119));
#50444=CARTESIAN_POINT('Ctrl Pts',(-8.18485787866432,-35.7526687479855,
2.69010588561904));
#50445=CARTESIAN_POINT('Ctrl Pts',(-8.16817698260155,-35.7535209183249,
2.69748506803798));
#50446=CARTESIAN_POINT('Ctrl Pts',(-8.15163776364548,-35.7538884883522,
2.70389891515113));
#50447=CARTESIAN_POINT('Ctrl Pts',(-8.13962292624303,-35.7541555078605,
2.70855822405763));
#50448=CARTESIAN_POINT('Ctrl Pts',(-8.12768358697008,-35.7541679447663,
2.71270833239839));
#50449=CARTESIAN_POINT('Ctrl Pts',(-8.11583718940693,-35.7539295817332,
2.71637303718402));
#50450=CARTESIAN_POINT('Ctrl Pts',(-8.1017603154413,-35.7536463389703,2.7207277439304));
#50451=CARTESIAN_POINT('Ctrl Pts',(-8.08781260069513,-35.7529999537971,
2.72439784378331));
#50452=CARTESIAN_POINT('Ctrl Pts',(-8.07401645344997,-35.7520148983668,
2.72743067381259));
#50453=CARTESIAN_POINT('Ctrl Pts',(-8.06812797876998,-35.7515944567857,
2.72872514700998));
#50454=CARTESIAN_POINT('Ctrl Pts',(-8.06203309974918,-35.7510936806319,
2.72995126932923));
#50455=CARTESIAN_POINT('Ctrl Pts',(-8.05603177437216,-35.7505342564226,
2.73104354710272));
#50456=CARTESIAN_POINT('Ctrl Pts',(-8.04981368520668,-35.7499546261916,
2.73217527720604));
#50457=CARTESIAN_POINT('Ctrl Pts',(-8.04369619708462,-35.7493120766649,
2.73316328375298));
#50458=CARTESIAN_POINT('Ctrl Pts',(-8.03801937794833,-35.7486606699676,
2.73398364682132));
#50459=CARTESIAN_POINT('Ctrl Pts',(-8.03633851273534,-35.7484677931415,
2.73422655041055));
#50460=CARTESIAN_POINT('Ctrl Pts',(-8.03469631248028,-35.7482743247953,
2.73445506571509));
#50461=CARTESIAN_POINT('Ctrl Pts',(-8.03310166808097,-35.7480820929171,
2.73466929183492));
#50462=CARTESIAN_POINT('Ctrl Pts',(-8.01904331881673,-35.7463873809903,
2.73655790450332));
#50463=CARTESIAN_POINT('Ctrl Pts',(-8.00417431429791,-35.7442048206208,
2.73794428304994));
#50464=CARTESIAN_POINT('Ctrl Pts',(-7.98849033151252,-35.7414881426324,
2.73862510052901));
#50465=CARTESIAN_POINT('Ctrl Pts',(-7.97700158377802,-35.7394981361073,
2.73912380933132));
#50466=CARTESIAN_POINT('Ctrl Pts',(-7.96507585493778,-35.7372214968454,
2.739243343789));
#50467=CARTESIAN_POINT('Ctrl Pts',(-7.95271576416055,-35.73465776535,2.73890188665224));
#50468=CARTESIAN_POINT('Ctrl Pts',(-7.93982887381466,-35.7319847650257,
2.738545876267));
#50469=CARTESIAN_POINT('Ctrl Pts',(-7.92646901975442,-35.7290141149945,
2.73768804175695));
#50470=CARTESIAN_POINT('Ctrl Pts',(-7.91264398168322,-35.7257422917824,
2.7362414335458));
#50471=CARTESIAN_POINT('Ctrl Pts',(-7.91078813887005,-35.7253030894046,
2.73604724402977));
#50472=CARTESIAN_POINT('Ctrl Pts',(-7.90892391692481,-35.7248585353482,
2.73584246338455));
#50473=CARTESIAN_POINT('Ctrl Pts',(-7.90705133663703,-35.7244086969031,
2.73562690117746));
#50474=CARTESIAN_POINT('Ctrl Pts',(-7.90169678951765,-35.723122406982,2.73501051212189));
#50475=CARTESIAN_POINT('Ctrl Pts',(-7.89627373543874,-35.7217919098803,
2.73430590796455));
#50476=CARTESIAN_POINT('Ctrl Pts',(-7.89078303968402,-35.7204175849161,
2.73350900493847));
#50477=CARTESIAN_POINT('Ctrl Pts',(-7.8881614288968,-35.7197613939136,2.73312851225359));
#50478=CARTESIAN_POINT('Ctrl Pts',(-7.88552439629046,-35.7190952432039,
2.7327269889564));
#50479=CARTESIAN_POINT('Ctrl Pts',(-7.88287195037857,-35.7184189512514,
2.73230381816035));
#50480=CARTESIAN_POINT('Ctrl Pts',(-7.87876808903727,-35.7173725931006,
2.7316490887791));
#50481=CARTESIAN_POINT('Ctrl Pts',(-7.87462744214398,-35.7163022013537,
2.73094255475833));
#50482=CARTESIAN_POINT('Ctrl Pts',(-7.87045039924609,-35.715207775882,2.73018200139144));
#50483=CARTESIAN_POINT('Ctrl Pts',(-7.86836187779715,-35.7146605631461,
2.72980172470799));
#50484=CARTESIAN_POINT('Ctrl Pts',(-7.86626425749866,-35.7141073419777,
2.7294079434931));
#50485=CARTESIAN_POINT('Ctrl Pts',(-7.86415759379027,-35.7135481123587,
2.72900038410796));
#50486=CARTESIAN_POINT('Ctrl Pts',(-7.86263403344017,-35.7131436718821,
2.7287056330677));
#50487=CARTESIAN_POINT('Ctrl Pts',(-7.86043402929441,-35.7125561966667,
2.72826931136775));
#50488=CARTESIAN_POINT('Ctrl Pts',(-7.85901499360382,-35.7121757253659,
2.72798160782829));
#50489=CARTESIAN_POINT('Ctrl Pts',(-7.85847189435825,-35.7120301098062,
2.72787149673223));
#50490=CARTESIAN_POINT('Ctrl Pts',(-7.85804317970972,-35.7119149484461,
2.72778377381318));
#50491=CARTESIAN_POINT('Ctrl Pts',(-7.85781053033946,-35.7118523981339,
2.72773609981549));
#50492=CARTESIAN_POINT('Ctrl Pts',(-7.84994145632762,-35.7097367120469,
2.72612358646172));
#50493=CARTESIAN_POINT('Ctrl Pts',(-7.84068239994918,-35.7072048188565,
2.72406334905565));
#50494=CARTESIAN_POINT('Ctrl Pts',(-7.83005001361465,-35.7042419520675,
2.72135502913469));
#50495=CARTESIAN_POINT('Ctrl Pts',(-7.81915993834101,-35.7012072765635,
2.7185810697547));
#50496=CARTESIAN_POINT('Ctrl Pts',(-7.80682873097179,-35.6977199958601,
2.71512684077666));
#50497=CARTESIAN_POINT('Ctrl Pts',(-7.79308077972864,-35.6937771023739,
2.71072322623729));
#50498=CARTESIAN_POINT('Ctrl Pts',(-7.77861281360236,-35.6896277096106,
2.70608898329724));
#50499=CARTESIAN_POINT('Ctrl Pts',(-7.76257469854674,-35.6849738906446,
2.70040264847822));
#50500=CARTESIAN_POINT('Ctrl Pts',(-7.74501367358198,-35.6798298211235,
2.6932991938513));
#50501=CARTESIAN_POINT('Ctrl Pts',(-7.73986644545326,-35.6783220674823,
2.69121713420272));
#50502=CARTESIAN_POINT('Ctrl Pts',(-7.73458856949642,-35.6767722872443,
2.68901304949919));
#50503=CARTESIAN_POINT('Ctrl Pts',(-7.72918178710914,-35.675180990914,2.68667714192434));
#50504=CARTESIAN_POINT('Ctrl Pts',(-7.71231260111563,-35.6702161390217,
2.67938909951367));
#50505=CARTESIAN_POINT('Ctrl Pts',(-7.69419464788743,-35.6648336045937,
2.67082125009322));
#50506=CARTESIAN_POINT('Ctrl Pts',(-7.67493810743223,-35.6590387042651,
2.66069067140836));
#50507=CARTESIAN_POINT('Ctrl Pts',(-7.66080762111701,-35.6547863952909,
2.65325683334151));
#50508=CARTESIAN_POINT('Ctrl Pts',(-7.64606456718289,-35.6503122888981,
2.64498127475074));
#50509=CARTESIAN_POINT('Ctrl Pts',(-7.63076909921078,-35.6456126593791,
2.63575755957871));
#50510=CARTESIAN_POINT('Ctrl Pts',(-7.61363620758056,-35.6403484697904,
2.62542581211217));
#50511=CARTESIAN_POINT('Ctrl Pts',(-7.59581096096198,-35.6348035164443,
2.61390435324381));
#50512=CARTESIAN_POINT('Ctrl Pts',(-7.5774141102286,-35.6289786177062,2.60106619052009));
#50513=CARTESIAN_POINT('Ctrl Pts',(-7.57640807967092,-35.6286600835065,
2.60036413644617));
#50514=CARTESIAN_POINT('Ctrl Pts',(-7.57540034858448,-35.6283407047128,
2.59965815139513));
#50515=CARTESIAN_POINT('Ctrl Pts',(-7.57439093986371,-35.6280204787728,
2.59894821699336));
#50516=CARTESIAN_POINT('Ctrl Pts',(-7.56465692262456,-35.6249324483681,
2.59210211633733));
#50517=CARTESIAN_POINT('Ctrl Pts',(-7.55476669689201,-35.6217664170923,
2.58488857366488));
#50518=CARTESIAN_POINT('Ctrl Pts',(-7.54474277191305,-35.6185223831134,
2.57729276601061));
#50519=CARTESIAN_POINT('Ctrl Pts',(-7.53973080942357,-35.6169003661239,
2.57349486218347));
#50520=CARTESIAN_POINT('Ctrl Pts',(-7.53468542030573,-35.6152588484409,
2.56960139494148));
#50521=CARTESIAN_POINT('Ctrl Pts',(-7.52960981050698,-35.6135978298282,
2.56561085056718));
#50522=CARTESIAN_POINT('Ctrl Pts',(-7.52618192995733,-35.6124760388276,
2.56291578337612));
#50523=CARTESIAN_POINT('Ctrl Pts',(-7.52233273639884,-35.6112115631965,
2.55985046954054));
#50524=CARTESIAN_POINT('Ctrl Pts',(-7.51888963042791,-35.6100752410138,
2.55707291744137));
#50525=CARTESIAN_POINT('Ctrl Pts',(-7.51723458255391,-35.6095290284869,
2.55573779103647));
#50526=CARTESIAN_POINT('Ctrl Pts',(-7.51567307453838,-35.6090125180102,
2.55446999111925));
#50527=CARTESIAN_POINT('Ctrl Pts',(-7.51429555183542,-35.6085562709412,
2.55334652921959));
#50528=CARTESIAN_POINT('Ctrl Pts',(-7.49347539579041,-35.6016604606929,
2.53636629941192));
#50529=CARTESIAN_POINT('Ctrl Pts',(-7.47369655728357,-35.5948224054086,
2.51897852016351));
#50530=CARTESIAN_POINT('Ctrl Pts',(-7.45495956403958,-35.5880314450045,
2.50143384534816));
#50531=CARTESIAN_POINT('Ctrl Pts',(-7.43600847283916,-35.581162887799,2.48368869658401));
#50532=CARTESIAN_POINT('Ctrl Pts',(-7.41812311910607,-35.5743420635078,
2.46578288578056));
#50533=CARTESIAN_POINT('Ctrl Pts',(-7.40128135426698,-35.5675671484218,
2.44792790971538));
#50534=CARTESIAN_POINT('Ctrl Pts',(-7.38389671326328,-35.560573851239,2.42949739771213));
#50535=CARTESIAN_POINT('Ctrl Pts',(-7.36762388066498,-35.5536294822877,
2.41112096378186));
#50536=CARTESIAN_POINT('Ctrl Pts',(-7.35241586795669,-35.5467450555932,
2.39298218315277));
#50537=CARTESIAN_POINT('Ctrl Pts',(-7.3494232602091,-35.5453903494222,2.3894128637102));
#50538=CARTESIAN_POINT('Ctrl Pts',(-7.34647182064179,-35.5440380011469,
2.38585260191175));
#50539=CARTESIAN_POINT('Ctrl Pts',(-7.34356110202383,-35.5426881450861,
2.38230258867009));
#50540=CARTESIAN_POINT('Ctrl Pts',(-7.32870011786219,-35.5357963110845,
2.36417761766375));
#50541=CARTESIAN_POINT('Ctrl Pts',(-7.31489650839871,-35.5289775157615,
2.34631671551307));
#50542=CARTESIAN_POINT('Ctrl Pts',(-7.30207897807166,-35.5222043598003,
2.32884768056689));
#50543=CARTESIAN_POINT('Ctrl Pts',(-7.28834454310235,-35.514946684748,2.31012899464824));
#50544=CARTESIAN_POINT('Ctrl Pts',(-7.27574201356474,-35.5077416746932,
2.29186029304521));
#50545=CARTESIAN_POINT('Ctrl Pts',(-7.26416802488409,-35.5005907838209,
2.27414872095136));
#50546=CARTESIAN_POINT('Ctrl Pts',(-7.25296364227466,-35.4936682509291,
2.25700275374595));
#50547=CARTESIAN_POINT('Ctrl Pts',(-7.24272271209379,-35.4867971847728,
2.24037824521197));
#50548=CARTESIAN_POINT('Ctrl Pts',(-7.23334333153,-35.4800020975,2.22433302544));
#50549=CARTESIAN_POINT('Ctrl Pts',(-7.23334333044,-35.4800020975,2.22433302572));
#50550=CARTESIAN_POINT('Ctrl Pts',(-7.22937402512,-35.477126751,2.21754286118));
#50551=CARTESIAN_POINT('Ctrl Pts',(-7.22542564343,-35.4742071929,2.21065452768));
#50552=CARTESIAN_POINT('Ctrl Pts',(-7.22151371785,-35.4712377752,2.20368850558));
#50553=CARTESIAN_POINT('Ctrl Pts',(-7.21764954964,-35.4682109676,2.19666066586));
#50554=CARTESIAN_POINT('Ctrl Pts',(-7.21384189759,-35.46511484,2.18958432614));
#50555=CARTESIAN_POINT('Ctrl Pts',(-8.75956299023,-36.3742356128,2.0634404101));
#50556=CARTESIAN_POINT('Ctrl Pts',(-8.75956299023,-35.3373826802055,2.0634404101));
#50557=CARTESIAN_POINT('Ctrl Pts',(-8.92890465395,-36.3742356128,1.78598462948));
#50558=CARTESIAN_POINT('Ctrl Pts',(-8.92890465395,-35.3373826802055,1.78598462948));
#50559=CARTESIAN_POINT('Ctrl Pts',(-9.07291332076,-36.3742356128,1.49306717121));
#50560=CARTESIAN_POINT('Ctrl Pts',(-9.07291332076,-35.3373826802055,1.49306717121));
#50561=CARTESIAN_POINT('Ctrl Pts',(-9.12674872803,-36.3742356128,1.15064845916));
#50562=CARTESIAN_POINT('Ctrl Pts',(-9.12674872803,-35.3373826802055,1.15064845916));
#50563=CARTESIAN_POINT('Ctrl Pts',(-9.18664865847,-36.3742356128,0.831017278590001));
#50564=CARTESIAN_POINT('Ctrl Pts',(-9.18664865847,-35.3373826802055,0.831017278590001));
#50565=CARTESIAN_POINT('Ctrl Pts',(-9.23698117862,-36.3742356128,0.509886547135));
#50566=CARTESIAN_POINT('Ctrl Pts',(-9.23698117862,-35.3373826802055,0.509886547135));
#50567=CARTESIAN_POINT('',(-9.23698117854899,-35.5153448503988,0.509886547089706));
#50568=CARTESIAN_POINT('',(-9.23698117862,-36.1242356128,0.509886547138));
#50569=CARTESIAN_POINT('',(-9.22799880548,-35.5169181946,0.566467047115));
#50570=CARTESIAN_POINT('Ctrl Pts',(-9.23698117862,-35.5153448509,0.509886547139));
#50571=CARTESIAN_POINT('Ctrl Pts',(-9.23547079661,-35.5156173384,0.519523062039));
#50572=CARTESIAN_POINT('Ctrl Pts',(-9.23395444171,-35.5158907435,0.529141367463));
#50573=CARTESIAN_POINT('Ctrl Pts',(-9.2324173579,-35.5161611506,0.538838588998));
#50574=CARTESIAN_POINT('Ctrl Pts',(-9.2306125394,-35.5164751965,0.550165758707));
#50575=CARTESIAN_POINT('Ctrl Pts',(-9.22879492211,-35.5167839497,0.561507557195));
#50576=CARTESIAN_POINT('Ctrl Pts',(-9.22852978607,-35.5168288241,0.563160610681));
#50577=CARTESIAN_POINT('Ctrl Pts',(-9.22826440991,-35.5168735732,0.564813796021));
#50578=CARTESIAN_POINT('Ctrl Pts',(-9.22799880548,-35.5169181946,0.566467047115));
#50579=CARTESIAN_POINT('Ctrl Pts',(-9.22799880548,-35.5169181946,0.566467047115));
#50580=CARTESIAN_POINT('Ctrl Pts',(-9.22709573015,-35.5170698741,0.572088224967));
#50581=CARTESIAN_POINT('Ctrl Pts',(-9.22618896279,-35.5172202096,0.57771674331));
#50582=CARTESIAN_POINT('Ctrl Pts',(-9.22528372099,-35.5173684625,0.58332051525));
#50583=CARTESIAN_POINT('Ctrl Pts',(-9.21064489493,-35.5197392711,0.67370187071));
#50584=CARTESIAN_POINT('Ctrl Pts',(-9.19547141468,-35.5218042907,0.763606652472));
#50585=CARTESIAN_POINT('Ctrl Pts',(-9.18087022532,-35.5239641094,0.847743194451));
#50586=CARTESIAN_POINT('Ctrl Pts',(-9.1488371776,-35.5298747429,1.02282666839));
#50587=CARTESIAN_POINT('Ctrl Pts',(-9.1112963015,-35.5399157471,1.19686722852));
#50588=CARTESIAN_POINT('Ctrl Pts',(-9.08965016934,-35.5466085932,1.28690888429));
#50589=CARTESIAN_POINT('Ctrl Pts',(-9.04054093324,-35.5631550729,1.46510383868));
#50590=CARTESIAN_POINT('Ctrl Pts',(-8.97813093642,-35.5847442368,1.63735111856));
#50591=CARTESIAN_POINT('Ctrl Pts',(-8.94306195143,-35.596524942,1.72177132487));
#50592=CARTESIAN_POINT('Ctrl Pts',(-8.89434925659,-35.6115263375,1.82461373716));
#50593=CARTESIAN_POINT('Ctrl Pts',(-8.84001654494,-35.6256966309,1.92519756404));
#50594=CARTESIAN_POINT('Ctrl Pts',(-8.82896553279,-35.6284769797,1.94517168962));
#50595=CARTESIAN_POINT('Ctrl Pts',(-8.80877742677,-35.6333588617,1.98085549694));
#50596=CARTESIAN_POINT('Ctrl Pts',(-8.78793522997,-35.6380188734,2.01638522454));
#50597=CARTESIAN_POINT('Ctrl Pts',(-8.77859596185,-35.6400309319,2.03207294823));
#50598=CARTESIAN_POINT('Ctrl Pts',(-8.76913081737,-35.641984033,2.04776380401));
#50599=CARTESIAN_POINT('Ctrl Pts',(-8.75956299023,-35.6438772164,2.0634404101));
#50600=CARTESIAN_POINT('Ctrl Pts',(-1.87043161103,-36.3742356128,-8.24476960824));
#50601=CARTESIAN_POINT('Ctrl Pts',(-1.87043161103,-35.2215350722322,-8.24476960824));
#50602=CARTESIAN_POINT('Ctrl Pts',(-2.47265813357,-36.3742356128,-8.13634296351));
#50603=CARTESIAN_POINT('Ctrl Pts',(-2.47265813357,-35.2215350722322,-8.13634296351));
#50604=CARTESIAN_POINT('Ctrl Pts',(-3.05192283465,-36.3742356128,-7.98771609515));
#50605=CARTESIAN_POINT('Ctrl Pts',(-3.05192283465,-35.2215350722322,-7.98771609515));
#50606=CARTESIAN_POINT('Ctrl Pts',(-3.608285111,-36.3742356128,-7.79892601222));
#50607=CARTESIAN_POINT('Ctrl Pts',(-3.608285111,-35.2215350722322,-7.79892601222));
#50608=CARTESIAN_POINT('Ctrl Pts',(-4.84313848674,-36.3742356128,-7.27000777732));
#50609=CARTESIAN_POINT('Ctrl Pts',(-4.84313848674,-35.2215350722322,-7.27000777732));
#50610=CARTESIAN_POINT('Ctrl Pts',(-5.97499470659,-36.3742356128,-6.53839758248));
#50611=CARTESIAN_POINT('Ctrl Pts',(-5.97499470659,-35.2215350722322,-6.53839758248));
#50612=CARTESIAN_POINT('Ctrl Pts',(-6.59156749188,-36.3742356128,-6.06232184959));
#50613=CARTESIAN_POINT('Ctrl Pts',(-6.59156749188,-35.2215350722322,-6.06232184959));
#50614=CARTESIAN_POINT('Ctrl Pts',(-7.62010012329,-36.3742356128,-5.1678005996));
#50615=CARTESIAN_POINT('Ctrl Pts',(-7.62010012329,-35.2215350722322,-5.1678005996));
#50616=CARTESIAN_POINT('Ctrl Pts',(-8.47746400168,-36.3742356128,-4.11735171219));
#50617=CARTESIAN_POINT('Ctrl Pts',(-8.47746400168,-35.2215350722322,-4.11735171219));
#50618=CARTESIAN_POINT('Ctrl Pts',(-8.78407978672,-36.3742356128,-3.65866522624));
#50619=CARTESIAN_POINT('Ctrl Pts',(-8.78407978672,-35.2215350722322,-3.65866522624));
#50620=CARTESIAN_POINT('Ctrl Pts',(-9.22504359392,-36.3742356128,-2.71647636201));
#50621=CARTESIAN_POINT('Ctrl Pts',(-9.22504359392,-35.2215350722322,-2.71647636201));
#50622=CARTESIAN_POINT('Ctrl Pts',(-9.38605456704,-36.3742356128,-1.68617604095));
#50623=CARTESIAN_POINT('Ctrl Pts',(-9.38605456704,-35.2215350722322,-1.68617604095));
#50624=CARTESIAN_POINT('Ctrl Pts',(-9.40005841918,-36.3742356128,-1.17735235373));
#50625=CARTESIAN_POINT('Ctrl Pts',(-9.40005841918,-35.2215350722322,-1.17735235373));
#50626=CARTESIAN_POINT('Ctrl Pts',(-9.36972184244,-36.3742356128,-0.530817230024));
#50627=CARTESIAN_POINT('Ctrl Pts',(-9.36972184244,-35.2215350722322,-0.530817230024));
#50628=CARTESIAN_POINT('Ctrl Pts',(-9.2950327654,-36.3742356128,0.106470788818));
#50629=CARTESIAN_POINT('Ctrl Pts',(-9.2950327654,-35.2215350722322,0.106470788818));
#50630=CARTESIAN_POINT('Ctrl Pts',(-9.27733443288,-36.3742356128,0.241562002067001));
#50631=CARTESIAN_POINT('Ctrl Pts',(-9.27733443288,-35.2215350722322,0.241562002067001));
#50632=CARTESIAN_POINT('Ctrl Pts',(-9.25795835827,-36.3742356128,0.376048284641));
#50633=CARTESIAN_POINT('Ctrl Pts',(-9.25795835827,-35.2215350722322,0.376048284641));
#50634=CARTESIAN_POINT('Ctrl Pts',(-9.23698117862,-36.3742356128,0.509886547165));
#50635=CARTESIAN_POINT('Ctrl Pts',(-9.23698117862,-35.2215350722322,0.509886547165));
#50636=CARTESIAN_POINT('',(-1.8704316154347,-35.4944687624331,-8.24476961257036));
#50637=CARTESIAN_POINT('',(-1.87043161103,-36.1242356128,-8.24476960824));
#50638=CARTESIAN_POINT('',(-2.0299262428936,-35.4952698980321,-8.21479979569791));
#50639=CARTESIAN_POINT('Origin',(-1.87573872781909,-33.331129330927,-7.77578136547059));
#50640=CARTESIAN_POINT('',(-8.91162791630276,-35.4775418018593,-3.31601642789431));
#50641=CARTESIAN_POINT('Ctrl Pts',(-2.02993009745,-35.4952697797,-8.21479904026));
#50642=CARTESIAN_POINT('Ctrl Pts',(-2.18929689584727,-35.4902364571318,
-8.18359011989225));
#50643=CARTESIAN_POINT('Ctrl Pts',(-2.34325066281365,-35.4854550094663,
-8.14962872511168));
#50644=CARTESIAN_POINT('Ctrl Pts',(-2.49201818344239,-35.4809648403771,
-8.11335881534916));
#50645=CARTESIAN_POINT('Ctrl Pts',(-2.65136293418602,-35.4761554245094,
-8.0745101492816));
#50646=CARTESIAN_POINT('Ctrl Pts',(-2.80475858050197,-35.4716799045491,
-8.03301402245608));
#50647=CARTESIAN_POINT('Ctrl Pts',(-2.95252830755803,-35.4675538289942,
-7.98939303684412));
#50648=CARTESIAN_POINT('Ctrl Pts',(-3.02398660722482,-35.4655585465414,
-7.96829885521626));
#50649=CARTESIAN_POINT('Ctrl Pts',(-3.09412984908824,-35.463644537325,-7.94670735028006));
#50650=CARTESIAN_POINT('Ctrl Pts',(-3.16299705647906,-35.4618113955355,
-7.92467486461585));
#50651=CARTESIAN_POINT('Ctrl Pts',(-3.29831147262683,-35.4582095286912,
-7.88138411642247));
#50652=CARTESIAN_POINT('Ctrl Pts',(-3.42893430185573,-35.454884995394,-7.83631198095569));
#50653=CARTESIAN_POINT('Ctrl Pts',(-3.55481517329765,-35.4518612230206,
-7.7899762595127));
#50654=CARTESIAN_POINT('Ctrl Pts',(-3.69766906756152,-35.4484297432893,
-7.73739290688861));
#50655=CARTESIAN_POINT('Ctrl Pts',(-3.83441616439784,-35.4453853684485,
-7.68318308540026));
#50656=CARTESIAN_POINT('Ctrl Pts',(-3.96503125082369,-35.4427217611445,
-7.62813243602623));
#50657=CARTESIAN_POINT('Ctrl Pts',(-4.01212236679739,-35.4417614414456,
-7.60828483200867));
#50658=CARTESIAN_POINT('Ctrl Pts',(-4.05841681338306,-35.4408502938001,
-7.58832810721544));
#50659=CARTESIAN_POINT('Ctrl Pts',(-4.10391457658464,-35.4399870947724,
-7.56829943995679));
#50660=CARTESIAN_POINT('Ctrl Pts',(-4.25389323618712,-35.4371416486662,
-7.50227701472747));
#50661=CARTESIAN_POINT('Ctrl Pts',(-4.40819154727007,-35.4345650870246,
-7.42976069922605));
#50662=CARTESIAN_POINT('Ctrl Pts',(-4.56648104744728,-35.432294211752,-7.3498427515548));
#50663=CARTESIAN_POINT('Ctrl Pts',(-4.70676304345842,-35.4302816782892,
-7.27901651732014));
#50664=CARTESIAN_POINT('Ctrl Pts',(-4.85017801583353,-35.4285109316766,
-7.20237417174943));
#50665=CARTESIAN_POINT('Ctrl Pts',(-4.99649524902321,-35.4269957372856,
-7.11931649038508));
#50666=CARTESIAN_POINT('Ctrl Pts',(-5.11556507709157,-35.4257627045682,
-7.05172592962735));
#50667=CARTESIAN_POINT('Ctrl Pts',(-5.23656919882029,-35.4247157623198,
-6.97987983296062));
#50668=CARTESIAN_POINT('Ctrl Pts',(-5.35943588605315,-35.4238515670765,
-6.90346517638933));
#50669=CARTESIAN_POINT('Ctrl Pts',(-5.37358279482046,-35.4237520633661,
-6.89466676894996));
#50670=CARTESIAN_POINT('Ctrl Pts',(-5.3877544121134,-35.42365495475,-6.88580784316436));
#50671=CARTESIAN_POINT('Ctrl Pts',(-5.40195064262958,-35.423560213071,-6.87688796232893));
#50672=CARTESIAN_POINT('Ctrl Pts',(-5.5317365229437,-35.4226940583409,-6.7953399355338));
#50673=CARTESIAN_POINT('Ctrl Pts',(-5.66358167884288,-35.4220280565828,
-6.70869588257285));
#50674=CARTESIAN_POINT('Ctrl Pts',(-5.79738679233785,-35.4215214553207,
-6.61659013521258));
#50675=CARTESIAN_POINT('Ctrl Pts',(-5.83350781056089,-35.4213846970688,
-6.59172596304496));
#50676=CARTESIAN_POINT('Ctrl Pts',(-5.86977143199235,-35.4212594104568,
-6.56646389334973));
#50677=CARTESIAN_POINT('Ctrl Pts',(-5.90617504013701,-35.4211445378308,
-6.54079696194274));
#50678=CARTESIAN_POINT('Ctrl Pts',(-5.92159327159422,-35.4210958851608,
-6.52992609750379));
#50679=CARTESIAN_POINT('Ctrl Pts',(-5.93605165098445,-35.4210520297038,
-6.51968217529532));
#50680=CARTESIAN_POINT('Ctrl Pts',(-5.95172616209454,-35.4210060263787,
-6.5085204996939));
#50681=CARTESIAN_POINT('Ctrl Pts',(-5.95734063671402,-35.4209895483847,
-6.50452248381098));
#50682=CARTESIAN_POINT('Ctrl Pts',(-5.96311091048011,-35.4209728148743,
-6.50040632012766));
#50683=CARTESIAN_POINT('Ctrl Pts',(-5.9691361516031,-35.420955575595,-6.49609959272189));
#50684=CARTESIAN_POINT('Ctrl Pts',(-6.06908640339718,-35.4206696002674,
-6.42465705958041));
#50685=CARTESIAN_POINT('Ctrl Pts',(-6.16548414027397,-35.4204459918632,
-6.35344243759832));
#50686=CARTESIAN_POINT('Ctrl Pts',(-6.25844568390168,-35.4202640009878,
-6.28279230429464));
#50687=CARTESIAN_POINT('Ctrl Pts',(-6.35363024262543,-35.4200776581143,
-6.21045269481897));
#50688=CARTESIAN_POINT('Ctrl Pts',(-6.44521227760241,-35.4199348833781,
-6.1387046910448));
#50689=CARTESIAN_POINT('Ctrl Pts',(-6.53328629732009,-35.4198314487939,
-6.06786581553125));
#50690=CARTESIAN_POINT('Ctrl Pts',(-6.62786612394948,-35.4197203737565,
-5.99179424997572));
#50691=CARTESIAN_POINT('Ctrl Pts',(-6.71840025583166,-35.4196547552607,
-5.91677103106586));
#50692=CARTESIAN_POINT('Ctrl Pts',(-6.80497303596595,-35.419649997424,-5.84314099276948));
#50693=CARTESIAN_POINT('Ctrl Pts',(-6.84700206399384,-35.4196476876073,
-5.80739535842053));
#50694=CARTESIAN_POINT('Ctrl Pts',(-6.8880970092318,-35.4196600097299,-5.77197738755347));
#50695=CARTESIAN_POINT('Ctrl Pts',(-6.92826553348727,-35.419690092492,-5.73692300258239));
#50696=CARTESIAN_POINT('Ctrl Pts',(-7.02473825161427,-35.4197623422418,
-5.65273290939095));
#50697=CARTESIAN_POINT('Ctrl Pts',(-7.11586309787553,-35.4199125655208,
-5.5706480730014));
#50698=CARTESIAN_POINT('Ctrl Pts',(-7.20173998727502,-35.4201398128318,
-5.49111566364252));
#50699=CARTESIAN_POINT('Ctrl Pts',(-7.23835353620077,-35.4202366995565,
-5.45720707913734));
#50700=CARTESIAN_POINT('Ctrl Pts',(-7.27401300829813,-35.4203477035167,
-5.42376176294008));
#50701=CARTESIAN_POINT('Ctrl Pts',(-7.3087261154237,-35.4204728900179,-5.39081163268007));
#50702=CARTESIAN_POINT('Ctrl Pts',(-7.31344645414271,-35.4204899130601,
-5.38633102611551));
#50703=CARTESIAN_POINT('Ctrl Pts',(-7.31814930121898,-35.4205071935359,
-5.3818595672839));
#50704=CARTESIAN_POINT('Ctrl Pts',(-7.32283466808666,-35.4205247406587,
-5.37739734263404));
#50705=CARTESIAN_POINT('Ctrl Pts',(-7.37578536236207,-35.4207230457994,
-5.32696844348988));
#50706=CARTESIAN_POINT('Ctrl Pts',(-7.4265050614639,-35.4209546111681,-5.27771872821795));
#50707=CARTESIAN_POINT('Ctrl Pts',(-7.47503381051047,-35.4212195168391,
-5.22975918031341));
#50708=CARTESIAN_POINT('Ctrl Pts',(-7.50144522952509,-35.4213636898255,
-5.20365754488402));
#50709=CARTESIAN_POINT('Ctrl Pts',(-7.52720756230863,-35.4215177304207,
-5.1779379121768));
#50710=CARTESIAN_POINT('Ctrl Pts',(-7.55232793900539,-35.4216816385961,
-5.15261626108499));
#50711=CARTESIAN_POINT('Ctrl Pts',(-7.56488812735376,-35.4217635926838,
-5.13995543553908));
#50712=CARTESIAN_POINT('Ctrl Pts',(-7.57728782906225,-35.4218455841287,
-5.12739409426947));
#50713=CARTESIAN_POINT('Ctrl Pts',(-7.58952795253593,-35.4219285831362,
-5.11493418074097));
#50714=CARTESIAN_POINT('Ctrl Pts',(-7.59603051813133,-35.4219726763589,
-5.10831485167896));
#50715=CARTESIAN_POINT('Ctrl Pts',(-7.60248804511812,-35.422017468346,-5.10172414935278));
#50716=CARTESIAN_POINT('Ctrl Pts',(-7.60890067435508,-35.4220629582103,
-5.09516235913147));
#50717=CARTESIAN_POINT('Ctrl Pts',(-7.61200679164173,-35.4220849923633,
-5.09198399199302));
#50718=CARTESIAN_POINT('Ctrl Pts',(-7.61510237508418,-35.4221071902546,
-5.08881240815013));
#50719=CARTESIAN_POINT('Ctrl Pts',(-7.61818744096429,-35.4221295517926,
-5.08564763970962));
#50720=CARTESIAN_POINT('Ctrl Pts',(-7.61894665639572,-35.4221350548274,
-5.08486880997621));
#50721=CARTESIAN_POINT('Ctrl Pts',(-7.61970523486104,-35.4221405677729,
-5.08409039299812));
#50722=CARTESIAN_POINT('Ctrl Pts',(-7.62046317660273,-35.4221460906279,
-5.08331238925388));
#50723=CARTESIAN_POINT('Ctrl Pts',(-7.6206575511755,-35.422147506967,-5.08311286976962));
#50724=CARTESIAN_POINT('Ctrl Pts',(-7.62085188387294,-35.4221489239579,
-5.08291337746247));
#50725=CARTESIAN_POINT('Ctrl Pts',(-7.62104617469914,-35.4221503416005,
-5.08271391234048));
#50726=CARTESIAN_POINT('Ctrl Pts',(-7.62121633244005,-35.422151583156,-5.08253922300898));
#50727=CARTESIAN_POINT('Ctrl Pts',(-7.62138859966819,-35.4221528408801,
-5.08236235519101));
#50728=CARTESIAN_POINT('Ctrl Pts',(-7.62154789780562,-35.4221540045504,
-5.08219879236452));
#50729=CARTESIAN_POINT('Ctrl Pts',(-7.62225305804759,-35.4221591557344,
-5.08147475375261));
#50730=CARTESIAN_POINT('Ctrl Pts',(-7.6227731152015,-35.4221629636036,-5.08094062756502));
#50731=CARTESIAN_POINT('Ctrl Pts',(-7.62344669187689,-35.4221679057579,
-5.08024866069744));
#50732=CARTESIAN_POINT('Ctrl Pts',(-7.62378216463514,-35.4221703671823,
-5.07990402876144));
#50733=CARTESIAN_POINT('Ctrl Pts',(-7.62415571356334,-35.4221731105011,
-5.0795202395543));
#50734=CARTESIAN_POINT('Ctrl Pts',(-7.62460913497078,-35.422176446303,-5.07905429122528));
#50735=CARTESIAN_POINT('Ctrl Pts',(-7.62480121816504,-35.4221778594508,
-5.0788569012434));
#50736=CARTESIAN_POINT('Ctrl Pts',(-7.62500763509778,-35.4221793789766,
-5.07864476630863));
#50737=CARTESIAN_POINT('Ctrl Pts',(-7.62523156111189,-35.4221810287663,
-5.07841461473952));
#50738=CARTESIAN_POINT('Ctrl Pts',(-7.62538775764981,-35.4221821795546,
-5.07825407565059));
#50739=CARTESIAN_POINT('Ctrl Pts',(-7.62555247332383,-35.4221833937273,
-5.07808477041067));
#50740=CARTESIAN_POINT('Ctrl Pts',(-7.62572678528594,-35.4221846794553,
-5.07790558807117));
#50741=CARTESIAN_POINT('Ctrl Pts',(-7.62588995094337,-35.422185882968,-5.07773786347056));
#50742=CARTESIAN_POINT('Ctrl Pts',(-7.62605590764984,-35.4221871077609,
-5.07756725845795));
#50743=CARTESIAN_POINT('Ctrl Pts',(-7.62622054005713,-35.422188323481,-5.07739800334206));
#50744=CARTESIAN_POINT('Ctrl Pts',(-7.70695216467482,-35.422784482276,-4.99439951777019));
#50745=CARTESIAN_POINT('Ctrl Pts',(-7.78297578327702,-35.4235131623992,
-4.91349867411078));
#50746=CARTESIAN_POINT('Ctrl Pts',(-7.85437558442288,-35.424403953379,-4.83498231891968));
#50747=CARTESIAN_POINT('Ctrl Pts',(-7.9134915281878,-35.4251414897393,-4.76997417654936));
#50748=CARTESIAN_POINT('Ctrl Pts',(-7.96943659929543,-35.4259906431666,
-4.70660119463088));
#50749=CARTESIAN_POINT('Ctrl Pts',(-8.02227857318465,-35.4269587081494,
-4.6450340975051));
#50750=CARTESIAN_POINT('Ctrl Pts',(-8.08393265604328,-35.4280882109721,
-4.57319985990611));
#50751=CARTESIAN_POINT('Ctrl Pts',(-8.14136523220772,-35.4293803500542,
-4.50381970168519));
#50752=CARTESIAN_POINT('Ctrl Pts',(-8.19476584495109,-35.4308233199233,
-4.43713267964401));
#50753=CARTESIAN_POINT('Ctrl Pts',(-8.22146615132277,-35.4315448048578,
-4.40378916862343));
#50754=CARTESIAN_POINT('Ctrl Pts',(-8.24715933772014,-35.4323035759929,
-4.37111898073678));
#50755=CARTESIAN_POINT('Ctrl Pts',(-8.27187486588063,-35.4330958492025,
-4.33915071527316));
#50756=CARTESIAN_POINT('Ctrl Pts',(-8.28423262996087,-35.4334919858072,
-4.32316658254135));
#50757=CARTESIAN_POINT('Ctrl Pts',(-8.29634600764459,-35.4338964747233,
-4.30735795075904));
#50758=CARTESIAN_POINT('Ctrl Pts',(-8.30821901697159,-35.4343087198482,
-4.29172826253413));
#50759=CARTESIAN_POINT('Ctrl Pts',(-8.31415552163508,-35.4345148424107,
-4.28391341842168));
#50760=CARTESIAN_POINT('Ctrl Pts',(-8.32003193672778,-35.4347229028061,
-4.27614330971437));
#50761=CARTESIAN_POINT('Ctrl Pts',(-8.32584877735325,-35.4349328194777,
-4.2684183656988));
#50762=CARTESIAN_POINT('Ctrl Pts',(-8.32875719766598,-35.4350377778135,
-4.26455589369101));
#50763=CARTESIAN_POINT('Ctrl Pts',(-8.33165072448736,-35.4351432001474,
-4.26070471284826));
#50764=CARTESIAN_POINT('Ctrl Pts',(-8.33452942331843,-35.4352490758846,
-4.25686487626074));
#50765=CARTESIAN_POINT('Ctrl Pts',(-8.33477470837254,-35.4352580972298,
-4.25653769562102));
#50766=CARTESIAN_POINT('Ctrl Pts',(-8.33501937674538,-35.4352671032692,
-4.25621127527631));
#50767=CARTESIAN_POINT('Ctrl Pts',(-8.33525702577003,-35.4352758576722,
-4.25589416277902));
#50768=CARTESIAN_POINT('Ctrl Pts',(-8.33780845809389,-35.4353698461356,
-4.25248959978085));
#50769=CARTESIAN_POINT('Ctrl Pts',(-8.33979079821542,-35.4354432477629,
-4.24984122829577));
#50770=CARTESIAN_POINT('Ctrl Pts',(-8.34312110187758,-35.4355680524468,
-4.24537945221164));
#50771=CARTESIAN_POINT('Ctrl Pts',(-8.40612657614725,-35.4379292119982,
-4.16096783489886));
#50772=CARTESIAN_POINT('Ctrl Pts',(-8.46644700936824,-35.4406790565229,
-4.07605040377369));
#50773=CARTESIAN_POINT('Ctrl Pts',(-8.52390193196485,-35.4438618010421,
-3.99065934753446));
#50774=CARTESIAN_POINT('Ctrl Pts',(-8.57900386837241,-35.4469142007004,
-3.90876536285878));
#50775=CARTESIAN_POINT('Ctrl Pts',(-8.63146962841867,-35.4503649522411,
-3.82643584977495));
#50776=CARTESIAN_POINT('Ctrl Pts',(-8.68117225080198,-35.4542258470509,
-3.74371800949252));
#50777=CARTESIAN_POINT('Ctrl Pts',(-8.72917890183889,-35.4579549989736,
-3.66382269808739));
#50778=CARTESIAN_POINT('Ctrl Pts',(-8.7746075349702,-35.4620668174179,-3.58356521086298));
#50779=CARTESIAN_POINT('Ctrl Pts',(-8.81737998421833,-35.4665445123863,
-3.50300456770493));
#50780=CARTESIAN_POINT('Ctrl Pts',(-8.85038312017606,-35.4699994928333,
-3.44084413720063));
#50781=CARTESIAN_POINT('Ctrl Pts',(-8.88180556085801,-35.4736717653558,
-3.37850355041783));
#50782=CARTESIAN_POINT('Ctrl Pts',(-8.91162790031208,-35.4775418017954,
-3.31601642164564));
#50783=CARTESIAN_POINT('',(-9.00070817952036,-35.4796536185211,-3.11775012994394));
#50784=CARTESIAN_POINT('Origin',(-8.92974789374037,-35.4242646256046,-3.20847971418429));
#50785=CARTESIAN_POINT('Ctrl Pts',(-9.00070981177086,-35.4796534480026,
-3.11774626039934));
#50786=CARTESIAN_POINT('Ctrl Pts',(-9.03140777082974,-35.4767481961118,
-3.0449301336738));
#50787=CARTESIAN_POINT('Ctrl Pts',(-9.0605225219848,-35.4741877030414,-2.9706562389485));
#50788=CARTESIAN_POINT('Ctrl Pts',(-9.08787309691769,-35.4719966235732,
-2.89491150963051));
#50789=CARTESIAN_POINT('Ctrl Pts',(-9.11100123829071,-35.4701438071033,
-2.83086039508443));
#50790=CARTESIAN_POINT('Ctrl Pts',(-9.1328685889702,-35.4685547439761,-2.76575784469073));
#50791=CARTESIAN_POINT('Ctrl Pts',(-9.1533905300849,-35.4672329840956,-2.69960607538102));
#50792=CARTESIAN_POINT('Ctrl Pts',(-9.17578578500115,-35.4657905693992,
-2.62741574364917));
#50793=CARTESIAN_POINT('Ctrl Pts',(-9.19657795467695,-35.4646666084973,
-2.55397669769755));
#50794=CARTESIAN_POINT('Ctrl Pts',(-9.21568765704498,-35.4638527593822,
-2.4793089047899));
#50795=CARTESIAN_POINT('Ctrl Pts',(-9.230019933821,-35.4632423725458,-2.42330806010916));
#50796=CARTESIAN_POINT('Ctrl Pts',(-9.24340649218174,-35.4628061254186,
-2.36661637379091));
#50797=CARTESIAN_POINT('Ctrl Pts',(-9.25582614175848,-35.4625360683822,
-2.30924802224927));
#50798=CARTESIAN_POINT('Ctrl Pts',(-9.2569904839063,-35.462510750535,-2.30386973929224));
#50799=CARTESIAN_POINT('Ctrl Pts',(-9.25814633549059,-35.4624868908549,
-2.29848551281977));
#50800=CARTESIAN_POINT('Ctrl Pts',(-9.25929368381884,-35.4624644812833,
-2.29309535677824));
#50801=CARTESIAN_POINT('Ctrl Pts',(-9.25984943066533,-35.4624536266471,
-2.29048449994562));
#50802=CARTESIAN_POINT('Ctrl Pts',(-9.26040318249775,-35.4624431122304,
-2.28787225192695));
#50803=CARTESIAN_POINT('Ctrl Pts',(-9.26095493794436,-35.4624329370971,
-2.28525861433154));
#50804=CARTESIAN_POINT('Ctrl Pts',(-9.26119582484673,-35.4624284948096,
-2.28411754527979));
#50805=CARTESIAN_POINT('Ctrl Pts',(-9.26143633122959,-35.4624241171909,
-2.28297621136869));
#50806=CARTESIAN_POINT('Ctrl Pts',(-9.26167645698157,-35.4624198041622,
-2.28183461273309));
#50807=CARTESIAN_POINT('Ctrl Pts',(-9.26188214302222,-35.4624161097238,
-2.28085674633838));
#50808=CARTESIAN_POINT('Ctrl Pts',(-9.26208707226724,-35.4624124706879,
-2.27988097625192));
#50809=CARTESIAN_POINT('Ctrl Pts',(-9.2622953257845,-35.4624088164943,-2.27888779972648));
#50810=CARTESIAN_POINT('Ctrl Pts',(-9.26337757293257,-35.4623898264642,
-2.27372648251888));
#50811=CARTESIAN_POINT('Ctrl Pts',(-9.26452141238414,-35.4623710358368,
-2.26822537986269));
#50812=CARTESIAN_POINT('Ctrl Pts',(-9.26559401474242,-35.4623546396656,
-2.26302253304785));
#50813=CARTESIAN_POINT('Ctrl Pts',(-9.26611355650972,-35.4623466977701,
-2.26050240412191));
#50814=CARTESIAN_POINT('Ctrl Pts',(-9.26661651646356,-35.4623392968953,
-2.25805228847085));
#50815=CARTESIAN_POINT('Ctrl Pts',(-9.26708848510517,-35.4623325791954,
-2.25574488479086));
#50816=CARTESIAN_POINT('Ctrl Pts',(-9.26737027271032,-35.4623285684108,
-2.25436725564401));
#50817=CARTESIAN_POINT('Ctrl Pts',(-9.2676410212449,-35.4623247998691,-2.25304050065197));
#50818=CARTESIAN_POINT('Ctrl Pts',(-9.26789772426574,-35.4623212944959,
-2.25178010843329));
#50819=CARTESIAN_POINT('Ctrl Pts',(-9.26800536503634,-35.462319824622,-2.25125160047402));
#50820=CARTESIAN_POINT('Ctrl Pts',(-9.26811222752299,-35.4623183777677,
-2.25072646251089));
#50821=CARTESIAN_POINT('Ctrl Pts',(-9.26821936925621,-35.462316939489,-2.25019950193244));
#50822=CARTESIAN_POINT('Ctrl Pts',(-9.28299197902751,-35.4621186308583,
-2.17754263185134));
#50823=CARTESIAN_POINT('Ctrl Pts',(-9.2966570505828,-35.4621723300256,-2.10172353063556));
#50824=CARTESIAN_POINT('Ctrl Pts',(-9.30891553715524,-35.4624937676329,
-2.0227156018701));
#50825=CARTESIAN_POINT('Ctrl Pts',(-9.31872911874655,-35.4627510958248,
-1.95946548117058));
#50826=CARTESIAN_POINT('Ctrl Pts',(-9.32764138299525,-35.4631796938351,
-1.89417219253685));
#50827=CARTESIAN_POINT('Ctrl Pts',(-9.33551605715918,-35.4637801263595,
-1.82683775045262));
#50828=CARTESIAN_POINT('Ctrl Pts',(-9.3444045078848,-35.4644578578816,-1.75083474916722));
#50829=CARTESIAN_POINT('Ctrl Pts',(-9.35196984152661,-35.4653545131821,
-1.67223055084684));
#50830=CARTESIAN_POINT('Ctrl Pts',(-9.35804899336456,-35.4664615511483,
-1.59105350025987));
#50831=CARTESIAN_POINT('Ctrl Pts',(-9.36108856928353,-35.4670150701314,
-1.55046497496639));
#50832=CARTESIAN_POINT('Ctrl Pts',(-9.36375720753474,-35.4676162058835,
-1.50923361836706));
#50833=CARTESIAN_POINT('Ctrl Pts',(-9.36603846791738,-35.4682703204645,
-1.4673658482447));
#50834=CARTESIAN_POINT('Ctrl Pts',(-9.36717909810869,-35.468597377755,-1.44643196318352));
#50835=CARTESIAN_POINT('Ctrl Pts',(-9.36822292905917,-35.4689376875689,
-1.42533897812757));
#50836=CARTESIAN_POINT('Ctrl Pts',(-9.36916817438962,-35.4692912499044,
-1.40408790438279));
#50837=CARTESIAN_POINT('Ctrl Pts',(-9.36964079705484,-35.4694680310722,
-1.39346236751041));
#50838=CARTESIAN_POINT('Ctrl Pts',(-9.37008877629055,-35.4696481253704,
-1.38279730865109));
#50839=CARTESIAN_POINT('Ctrl Pts',(-9.37051190644291,-35.4698315327986,
-1.37209286098262));
#50840=CARTESIAN_POINT('Ctrl Pts',(-9.37072347151909,-35.4699232365127,
-1.36674063714838));
#50841=CARTESIAN_POINT('Ctrl Pts',(-9.370928824511,-35.4700157685094,-1.36137856611917));
#50842=CARTESIAN_POINT('Ctrl Pts',(-9.37112794080608,-35.4701091287885,
-1.35600666531908));
#50843=CARTESIAN_POINT('Ctrl Pts',(-9.37132705710116,-35.4702024890677,
-1.35063476451899));
#50844=CARTESIAN_POINT('Ctrl Pts',(-9.37159114630659,-35.4703329339099,
-1.34319574304992));
#50845=CARTESIAN_POINT('Ctrl Pts',(-9.37170655573111,-35.4703916944733,
-1.33986149128067));
#50846=CARTESIAN_POINT('Ctrl Pts',(-9.37411723708609,-35.471619089855,-1.27021537177055));
#50847=CARTESIAN_POINT('Ctrl Pts',(-9.37560542972272,-35.4730255082264,
-1.19532765056696));
#50848=CARTESIAN_POINT('Ctrl Pts',(-9.37579224143258,-35.4746404878121,
-1.11525292933757));
#50849=CARTESIAN_POINT('Ctrl Pts',(-9.3758128814272,-35.4748189197208,-1.10640582967405));
#50850=CARTESIAN_POINT('Ctrl Pts',(-9.37581767076311,-35.4749999006119,
-1.0974954518827));
#50851=CARTESIAN_POINT('Ctrl Pts',(-9.3758061275957,-35.4751834744026,-1.08852189959094));
#50852=CARTESIAN_POINT('Ctrl Pts',(-9.37571122871392,-35.4766926743333,
-1.01474838079893));
#50853=CARTESIAN_POINT('Ctrl Pts',(-9.37450956737563,-35.4783778620492,
-0.936702130807714));
#50854=CARTESIAN_POINT('Ctrl Pts',(-9.37195325945033,-35.4802306516693,
-0.854430817470772));
#50855=CARTESIAN_POINT('Ctrl Pts',(-9.36950548980399,-35.4820047736944,
-0.775652661851114));
#50856=CARTESIAN_POINT('Ctrl Pts',(-9.3658155900203,-35.4839320220494,-0.693000293466503));
#50857=CARTESIAN_POINT('Ctrl Pts',(-9.3606998335278,-35.486001697316,-0.606551309684227));
#50858=CARTESIAN_POINT('Ctrl Pts',(-9.35966829322684,-35.4864190262976,
-0.589119750758425));
#50859=CARTESIAN_POINT('Ctrl Pts',(-9.35857889303645,-35.4868421507618,
-0.571533953458252));
#50860=CARTESIAN_POINT('Ctrl Pts',(-9.35743029683677,-35.487270998256,-0.553794748002522));
#50861=CARTESIAN_POINT('Ctrl Pts',(-9.35152045370082,-35.4894775364817,
-0.462521660359738));
#50862=CARTESIAN_POINT('Ctrl Pts',(-9.34404045872566,-35.4918646701929,
-0.367181055595434));
#50863=CARTESIAN_POINT('Ctrl Pts',(-9.33483171081312,-35.4944086119262,
-0.267935924614849));
#50864=CARTESIAN_POINT('Ctrl Pts',(-9.32380215519322,-35.497455556756,-0.149067463608977));
#50865=CARTESIAN_POINT('Ctrl Pts',(-9.3102957030867,-35.5007250422298,-0.0246007203337422));
#50866=CARTESIAN_POINT('Ctrl Pts',(-9.2940739809111,-35.5042080159972,0.105138041622589));
#50867=CARTESIAN_POINT('Ctrl Pts',(-9.28332216793239,-35.506516542931,0.191129337093173));
#50868=CARTESIAN_POINT('Ctrl Pts',(-9.27137885445243,-35.5089196203523,
0.27943477778053));
#50869=CARTESIAN_POINT('Ctrl Pts',(-9.25816061636275,-35.5114289434686,
0.369973937452619));
#50870=CARTESIAN_POINT('Ctrl Pts',(-9.25143593074586,-35.512705543947,0.416035097849456));
#50871=CARTESIAN_POINT('Ctrl Pts',(-9.24438092873596,-35.5140098564956,
0.46267477320469));
#50872=CARTESIAN_POINT('Ctrl Pts',(-9.23698117833998,-35.5153448508951,
0.509886546917126));
#50873=CARTESIAN_POINT('Origin',(-1.81727342606,-36.1242356128,-7.9495168227));
#50874=CARTESIAN_POINT('',(-1.51727342288,-35.544540501139,-7.94951682269995));
#50875=CARTESIAN_POINT('',(-1.51727342606,-35.9593880834,-7.9495168227));
#50876=CARTESIAN_POINT('',(-1.51739959473689,-35.5460990323408,-7.95821664298045));
#50877=CARTESIAN_POINT('Origin',(-1.88128360390313,-40.0416488169456,-7.95002524253046));
#50878=CARTESIAN_POINT('',(-1.85568130399,-35.4970695389,-8.24704805785));
#50879=CARTESIAN_POINT('Ctrl Pts',(-1.51739959739202,-35.5460990330595,
-7.95821664354419));
#50880=CARTESIAN_POINT('Ctrl Pts',(-1.51784040157713,-35.551544433581,-7.9734107080064));
#50881=CARTESIAN_POINT('Ctrl Pts',(-1.51944015474546,-35.5564624662645,
-7.98865298821528));
#50882=CARTESIAN_POINT('Ctrl Pts',(-1.52221396870495,-35.5607753418337,
-8.00374326615405));
#50883=CARTESIAN_POINT('Ctrl Pts',(-1.52508034792987,-35.5652321428706,
-8.01933712349758));
#50884=CARTESIAN_POINT('Ctrl Pts',(-1.52920035542674,-35.5690427768125,
-8.03476806671595));
#50885=CARTESIAN_POINT('Ctrl Pts',(-1.53454083399218,-35.5721488750417,
-8.04981508926192));
#50886=CARTESIAN_POINT('Ctrl Pts',(-1.53985832132163,-35.5752416012412,
-8.06479733303534));
#50887=CARTESIAN_POINT('Ctrl Pts',(-1.54638538066407,-35.577636071276,-8.07939834280623));
#50888=CARTESIAN_POINT('Ctrl Pts',(-1.55404503872652,-35.579299076886,-8.09340906153831));
#50889=CARTESIAN_POINT('Ctrl Pts',(-1.56199623962116,-35.5810253800168,
-8.10795305794244));
#50890=CARTESIAN_POINT('Ctrl Pts',(-1.57116678649342,-35.581963465072,-8.12185869749068));
#50891=CARTESIAN_POINT('Ctrl Pts',(-1.58142798632441,-35.5821006264457,
-8.13491533384685));
#50892=CARTESIAN_POINT('Ctrl Pts',(-1.59149584448517,-35.5822352034228,
-8.14772595687882));
#50893=CARTESIAN_POINT('Ctrl Pts',(-1.602613595017,-35.5815989923742,-8.15971912255805));
#50894=CARTESIAN_POINT('Ctrl Pts',(-1.61462398371853,-35.5801988565566,
-8.17072375022459));
#50895=CARTESIAN_POINT('Ctrl Pts',(-1.62401123170297,-35.5791045187746,
-8.17932490139875));
#50896=CARTESIAN_POINT('Ctrl Pts',(-1.63394272185038,-35.5775439293429,
-8.18732229002714));
#50897=CARTESIAN_POINT('Ctrl Pts',(-1.64432960286547,-35.5755276116623,
-8.19465032514282));
#50898=CARTESIAN_POINT('Ctrl Pts',(-1.65751223624117,-35.5729685781358,
-8.20395078792408));
#50899=CARTESIAN_POINT('Ctrl Pts',(-1.67143040403805,-35.5696742607946,
-8.21217315079081));
#50900=CARTESIAN_POINT('Ctrl Pts',(-1.68587374540741,-35.565686430912,-8.2192114954254));
#50901=CARTESIAN_POINT('Ctrl Pts',(-1.70041483395494,-35.5616716128756,
-8.22629747296635));
#50902=CARTESIAN_POINT('Ctrl Pts',(-1.7154879825108,-35.5569536553932,-8.23218342574401));
#50903=CARTESIAN_POINT('Ctrl Pts',(-1.7308718665687,-35.5515942287824,-8.23681029394356));
#50904=CARTESIAN_POINT('Ctrl Pts',(-1.74453974665183,-35.5468326224185,
-8.24092105553498));
#50905=CARTESIAN_POINT('Ctrl Pts',(-1.75845269437942,-35.5415648512774,
-8.24403870478297));
#50906=CARTESIAN_POINT('Ctrl Pts',(-1.77245352352828,-35.5358486074623,
-8.24615310101329));
#50907=CARTESIAN_POINT('Ctrl Pts',(-1.78937968978829,-35.5289380100849,
-8.24870927977624));
#50908=CARTESIAN_POINT('Ctrl Pts',(-1.8064255637685,-35.521374841914,-8.24979779098238));
#50909=CARTESIAN_POINT('Ctrl Pts',(-1.82333732775558,-35.5132798883306,
-8.24945548954978));
#50910=CARTESIAN_POINT('Ctrl Pts',(-1.83055847689705,-35.5098234264757,
-8.24930933036154));
#50911=CARTESIAN_POINT('Ctrl Pts',(-1.83775521093275,-35.5062703565462,
-8.2489028379445));
#50912=CARTESIAN_POINT('Ctrl Pts',(-1.84490789334748,-35.5026317912376,
-8.24824123808703));
#50913=CARTESIAN_POINT('Ctrl Pts',(-1.84751151403415,-35.5013073309362,
-8.24800041164245));
#50914=CARTESIAN_POINT('Ctrl Pts',(-1.85010944922896,-35.499971478242,-8.24772578323896));
#50915=CARTESIAN_POINT('Ctrl Pts',(-1.85270080612586,-35.4986247745774,
-8.24741763123874));
#50916=CARTESIAN_POINT('Ctrl Pts',(-1.8536955086597,-35.4981078370806,-8.24729934588183));
#50917=CARTESIAN_POINT('Ctrl Pts',(-1.85468986954109,-35.4975889712202,
-8.24717603800027));
#50918=CARTESIAN_POINT('Ctrl Pts',(-1.85568130399,-35.4970695389,-8.24704805785));
#50919=CARTESIAN_POINT('Origin',(-1.86844266437558,-35.7037699017498,-8.22958286354931));
#50920=CARTESIAN_POINT('Origin',(-1.51727342606,-32.4742356128,-5.11808633804));
#50921=CARTESIAN_POINT('',(-1.51727342606,-35.544540554,-5.3083202352798));
#50922=CARTESIAN_POINT('Origin',(-1.09995011675E-15,-34.4242356128,2.38806125834E-16));
#50923=CARTESIAN_POINT('',(9.33061792149,-32.5742356128,12.8743764588));
#50924=CARTESIAN_POINT('',(-8.90572184957,-32.5742356128,13.1718684452));
#50925=CARTESIAN_POINT('Origin',(-4.19954447987E-15,-32.5742356128,1.22464679915E-17));
#50926=CARTESIAN_POINT('',(-8.90572184957,-36.2742356128,13.1718684452));
#50927=CARTESIAN_POINT('',(-8.90572184957,-34.4242356128,13.1718684452));
#50928=CARTESIAN_POINT('',(9.33061792149,-36.2742356128,12.8743764588));
#50929=CARTESIAN_POINT('Origin',(-1.55306943244E-15,-36.2742356128,4.65365783676E-16));
#50930=CARTESIAN_POINT('',(9.33061792149,-34.4242356128,12.8743764588));
#50931=CARTESIAN_POINT('Origin',(-5.10578311124E-15,-36.2742356128,-1.31099105572E-15));
#50932=CARTESIAN_POINT('Origin',(9.27193478991,-36.2742356128,12.7934055377));
#50933=CARTESIAN_POINT('Origin',(-8.84971102033,-36.2742356128,13.0890265053));
#50934=CARTESIAN_POINT('Origin',(9.15456852675,-36.2742356128,12.6314636954));
#50935=CARTESIAN_POINT('',(9.36397871523,-36.2742356128,12.4166442993));
#50936=CARTESIAN_POINT('Origin',(9.29417531907,-36.2742356128,12.4882507647));
#50937=CARTESIAN_POINT('Origin',(9.15456852675,-36.2742356128,12.6314636954));
#50938=CARTESIAN_POINT('Origin',(9.15456852675,-34.4242356128,12.6314636954));
#50939=CARTESIAN_POINT('',(9.36397871523,-32.5742356128,12.4166442993));
#50940=CARTESIAN_POINT('',(9.36397871523,-34.4242356128,12.4166442993));
#50941=CARTESIAN_POINT('Origin',(9.15456852675,-32.5742356128,12.6314636954));
#50942=CARTESIAN_POINT('Origin',(-0.316839226711,-36.2742356128,3.11924403781));
#50943=CARTESIAN_POINT('',(8.19033423541,-36.2742356128,11.2725524894));
#50944=CARTESIAN_POINT('Origin',(8.12053083925,-36.2742356128,11.3441589548));
#50945=CARTESIAN_POINT('',(8.77715647532,-36.2742356128,11.8445983944));
#50946=CARTESIAN_POINT('Origin',(7.97551483927,-32.4742356128,11.0631423009));
#50947=CARTESIAN_POINT('',(8.19033423541,-32.5742356128,11.2725524894));
#50948=CARTESIAN_POINT('',(8.19033423541,-34.4242356128,11.2725524894));
#50949=CARTESIAN_POINT('',(-0.24703583055,-32.5742356128,3.04763757243));
#50950=CARTESIAN_POINT('Origin',(8.39974442389,-36.2742356128,11.0577330933));
#50951=CARTESIAN_POINT('',(8.18492502775,-36.2742356128,10.8483229048));
#50952=CARTESIAN_POINT('Origin',(8.11331856237,-36.2742356128,10.7785195086));
#50953=CARTESIAN_POINT('Origin',(8.39974442389,-36.2742356128,11.0577330933));
#50954=CARTESIAN_POINT('Origin',(8.39974442389,-34.4242356128,11.0577330933));
#50955=CARTESIAN_POINT('',(8.18492502775,-32.5742356128,10.8483229048));
#50956=CARTESIAN_POINT('',(8.18492502775,-34.4242356128,10.8483229048));
#50957=CARTESIAN_POINT('Origin',(8.39974442389,-32.5742356128,11.0577330933));
#50958=CARTESIAN_POINT('Origin',(8.43647932171,-36.2742356128,10.447011287));
#50959=CARTESIAN_POINT('',(11.1928713102,-36.2742356128,7.76267932308));
#50960=CARTESIAN_POINT('Origin',(11.1212648448,-36.2742356128,7.69287592692));
#50961=CARTESIAN_POINT('',(9.68889816899,-36.2742356128,9.30550111394));
#50962=CARTESIAN_POINT('Origin',(11.4022814987,-32.4742356128,7.54785992694));
#50963=CARTESIAN_POINT('',(11.1928713102,-32.5742356128,7.76267932308));
#50964=CARTESIAN_POINT('',(11.1928713102,-34.4242356128,7.76267932308));
#50965=CARTESIAN_POINT('',(8.50808578709,-32.5742356128,10.5168146831));
#50966=CARTESIAN_POINT('Origin',(11.4076907064,-36.2742356128,7.97208951156));
#50967=CARTESIAN_POINT('',(11.6171008949,-36.2742356128,7.75727011542));
#50968=CARTESIAN_POINT('Origin',(11.686904291,-36.2742356128,7.68566365004));
#50969=CARTESIAN_POINT('Origin',(11.4076907064,-36.2742356128,7.97208951156));
#50970=CARTESIAN_POINT('Origin',(11.4076907064,-34.4242356128,7.97208951156));
#50971=CARTESIAN_POINT('',(11.6171008949,-32.5742356128,7.75727011542));
#50972=CARTESIAN_POINT('',(11.6171008949,-34.4242356128,7.75727011542));
#50973=CARTESIAN_POINT('Origin',(11.4076907064,-32.5742356128,7.97208951156));
#50974=CARTESIAN_POINT('Origin',(0.45986885604,-36.2742356128,-3.25867214427));
#50975=CARTESIAN_POINT('',(12.7650943916,-36.2742356128,8.87635684058));
#50976=CARTESIAN_POINT('Origin',(12.8348977878,-36.2742356128,8.80475037519));
#50977=CARTESIAN_POINT('',(12.1910976432,-36.2742356128,8.316813478));
#50978=CARTESIAN_POINT('Origin',(11.4022814987,-32.4742356128,7.54785992694));
#50979=CARTESIAN_POINT('',(12.7650943916,-32.5742356128,8.87635684058));
#50980=CARTESIAN_POINT('',(12.7650943916,-34.4242356128,8.87635684058));
#50981=CARTESIAN_POINT('',(0.390065459879,-32.5742356128,-3.18706567889));
#50982=CARTESIAN_POINT('Origin',(12.9745045801,-36.2742356128,8.66153744443));
#50983=CARTESIAN_POINT('',(13.2240142836,-36.2742356128,8.82810547221));
#50984=CARTESIAN_POINT('Origin',(13.1408443824,-36.2742356128,8.77258279628));
#50985=CARTESIAN_POINT('Origin',(12.9745045801,-36.2742356128,8.66153744443));
#50986=CARTESIAN_POINT('Origin',(12.9745045801,-34.4242356128,8.66153744443));
#50987=CARTESIAN_POINT('',(13.2240142836,-32.5742356128,8.82810547221));
#50988=CARTESIAN_POINT('',(13.2240142836,-34.4242356128,8.82810547221));
#50989=CARTESIAN_POINT('Origin',(12.9745045801,-32.5742356128,8.66153744443));
#50990=CARTESIAN_POINT('Origin',(5.04708629797E-13,-36.2742356128,3.05110563741E-13));
#50991=CARTESIAN_POINT('',(14.1979138053,-36.2742356128,7.15746069337));
#50992=CARTESIAN_POINT('Origin',(14.1086187499,-36.2742356128,7.11244521731));
#50993=CARTESIAN_POINT('Origin',(-1.55306943244E-15,-36.2742356128,4.65365783676E-16));
#50994=CARTESIAN_POINT('Origin',(-1.09995011675E-15,-34.4242356128,2.38806125834E-16));
#50995=CARTESIAN_POINT('',(14.1979138053,-32.5742356128,7.15746069337));
#50996=CARTESIAN_POINT('',(14.1979138053,-34.4242356128,7.15746069337));
#50997=CARTESIAN_POINT('Origin',(6.68547290961E-14,-32.5742356128,3.37630264166E-14));
#50998=CARTESIAN_POINT('Origin',(13.7514385284,-36.2742356128,6.93238331308));
#50999=CARTESIAN_POINT('',(14.2514385284,-36.2742356128,6.93238331308));
#51000=CARTESIAN_POINT('Origin',(14.1514385284,-36.2742356128,6.93238331308));
#51001=CARTESIAN_POINT('Origin',(13.7514385284,-36.2742356128,6.93238331308));
#51002=CARTESIAN_POINT('Origin',(13.7514385284,-34.4242356128,6.93238331308));
#51003=CARTESIAN_POINT('',(14.2514385284,-32.5742356128,6.93238331308));
#51004=CARTESIAN_POINT('',(14.2514385284,-34.4242356128,6.93238331308));
#51005=CARTESIAN_POINT('Origin',(13.7514385284,-32.5742356128,6.93238331308));
#51006=CARTESIAN_POINT('Origin',(14.1514385284,-36.2742356128,5.66451995282E-15));
#51007=CARTESIAN_POINT('',(14.2514385284,-36.2742356128,-6.93238331308));
#51008=CARTESIAN_POINT('Origin',(14.1514385284,-36.2742356128,-6.93238331308));
#51009=CARTESIAN_POINT('',(14.2514385284,-36.2742356128,7.1054273576E-15));
#51010=CARTESIAN_POINT('Origin',(14.2514385284,-32.4742356128,7.05028367309));
#51011=CARTESIAN_POINT('',(14.2514385284,-32.5742356128,-6.93238331308));
#51012=CARTESIAN_POINT('',(14.2514385284,-34.4242356128,-6.93238331308));
#51013=CARTESIAN_POINT('',(14.2514385284,-32.5742356128,3.5527136788E-15));
#51014=CARTESIAN_POINT('Origin',(13.7514385284,-36.2742356128,-6.93238331308));
#51015=CARTESIAN_POINT('',(14.1979138053,-36.2742356128,-7.15746069337));
#51016=CARTESIAN_POINT('Origin',(14.1086187499,-36.2742356128,-7.11244521731));
#51017=CARTESIAN_POINT('Origin',(13.7514385284,-36.2742356128,-6.93238331308));
#51018=CARTESIAN_POINT('Origin',(13.7514385284,-34.4242356128,-6.93238331308));
#51019=CARTESIAN_POINT('',(14.1979138053,-32.5742356128,-7.15746069337));
#51020=CARTESIAN_POINT('',(14.1979138053,-34.4242356128,-7.15746069337));
#51021=CARTESIAN_POINT('Origin',(13.7514385284,-32.5742356128,-6.93238331308));
#51022=CARTESIAN_POINT('Origin',(2.23287406962E-16,-36.2742356128,4.65365783676E-16));
#51023=CARTESIAN_POINT('',(13.2240142836,-36.2742356128,-8.82810547221));
#51024=CARTESIAN_POINT('Origin',(13.1408443824,-36.2742356128,-8.77258279628));
#51025=CARTESIAN_POINT('Origin',(-1.55306943244E-15,-36.2742356128,4.65365783676E-16));
#51026=CARTESIAN_POINT('Origin',(-1.09995011675E-15,-34.4242356128,2.38806125834E-16));
#51027=CARTESIAN_POINT('',(13.2240142836,-32.5742356128,-8.82810547221));
#51028=CARTESIAN_POINT('',(13.2240142836,-34.4242356128,-8.82810547221));
#51029=CARTESIAN_POINT('Origin',(1.12952603833E-15,-32.5742356128,1.22464679915E-17));
#51030=CARTESIAN_POINT('Origin',(12.9745045801,-36.2742356128,-8.66153744443));
#51031=CARTESIAN_POINT('',(12.7650943916,-36.2742356128,-8.87635684058));
#51032=CARTESIAN_POINT('Origin',(12.8348977878,-36.2742356128,-8.80475037519));
#51033=CARTESIAN_POINT('Origin',(12.9745045801,-36.2742356128,-8.66153744443));
#51034=CARTESIAN_POINT('Origin',(12.9745045801,-34.4242356128,-8.66153744443));
#51035=CARTESIAN_POINT('',(12.7650943916,-32.5742356128,-8.87635684058));
#51036=CARTESIAN_POINT('',(12.7650943916,-34.4242356128,-8.87635684058));
#51037=CARTESIAN_POINT('Origin',(12.9745045801,-32.5742356128,-8.66153744443));
#51038=CARTESIAN_POINT('Origin',(0.45986885604,-36.2742356128,3.25867214427));
#51039=CARTESIAN_POINT('',(11.6171008949,-36.2742356128,-7.75727011542));
#51040=CARTESIAN_POINT('Origin',(11.686904291,-36.2742356128,-7.68566365004));
#51041=CARTESIAN_POINT('',(12.1910976432,-36.2742356128,-8.316813478));
#51042=CARTESIAN_POINT('Origin',(11.4022814987,-32.4742356128,-7.54785992694));
#51043=CARTESIAN_POINT('',(11.6171008949,-32.5742356128,-7.75727011542));
#51044=CARTESIAN_POINT('',(11.6171008949,-34.4242356128,-7.75727011542));
#51045=CARTESIAN_POINT('',(0.390065459879,-32.5742356128,3.18706567889));
#51046=CARTESIAN_POINT('Origin',(11.4076907064,-36.2742356128,-7.97208951156));
#51047=CARTESIAN_POINT('',(11.1928713102,-36.2742356128,-7.76267932308));
#51048=CARTESIAN_POINT('Origin',(11.1212648448,-36.2742356128,-7.69287592692));
#51049=CARTESIAN_POINT('Origin',(11.4076907064,-36.2742356128,-7.97208951156));
#51050=CARTESIAN_POINT('Origin',(11.4076907064,-34.4242356128,-7.97208951156));
#51051=CARTESIAN_POINT('',(11.1928713102,-32.5742356128,-7.76267932308));
#51052=CARTESIAN_POINT('',(11.1928713102,-34.4242356128,-7.76267932308));
#51053=CARTESIAN_POINT('Origin',(11.4076907064,-32.5742356128,-7.97208951156));
#51054=CARTESIAN_POINT('Origin',(8.43647932171,-36.2742356128,-10.447011287));
#51055=CARTESIAN_POINT('',(8.18492502775,-36.2742356128,-10.8483229048));
#51056=CARTESIAN_POINT('Origin',(8.11331856237,-36.2742356128,-10.7785195086));
#51057=CARTESIAN_POINT('',(9.68889816899,-36.2742356128,-9.30550111394));
#51058=CARTESIAN_POINT('Origin',(11.4022814987,-32.4742356128,-7.54785992694));
#51059=CARTESIAN_POINT('',(8.18492502775,-32.5742356128,-10.8483229048));
#51060=CARTESIAN_POINT('',(8.18492502775,-34.4242356128,-10.8483229048));
#51061=CARTESIAN_POINT('',(8.50808578709,-32.5742356128,-10.5168146831));
#51062=CARTESIAN_POINT('Origin',(8.39974442389,-36.2742356128,-11.0577330933));
#51063=CARTESIAN_POINT('',(8.19033423541,-36.2742356128,-11.2725524894));
#51064=CARTESIAN_POINT('Origin',(8.12053083925,-36.2742356128,-11.3441589548));
#51065=CARTESIAN_POINT('Origin',(8.39974442389,-36.2742356128,-11.0577330933));
#51066=CARTESIAN_POINT('Origin',(8.39974442389,-34.4242356128,-11.0577330933));
#51067=CARTESIAN_POINT('',(8.19033423541,-32.5742356128,-11.2725524894));
#51068=CARTESIAN_POINT('',(8.19033423541,-34.4242356128,-11.2725524894));
#51069=CARTESIAN_POINT('Origin',(8.39974442389,-32.5742356128,-11.0577330933));
#51070=CARTESIAN_POINT('Origin',(-0.316839226711,-36.2742356128,-3.11924403781));
#51071=CARTESIAN_POINT('',(9.36397871523,-36.2742356128,-12.4166442993));
#51072=CARTESIAN_POINT('Origin',(9.29417531907,-36.2742356128,-12.4882507647));
#51073=CARTESIAN_POINT('',(8.77715647532,-36.2742356128,-11.8445983944));
#51074=CARTESIAN_POINT('Origin',(7.97551483927,-32.4742356128,-11.0631423009));
#51075=CARTESIAN_POINT('',(9.36397871523,-32.5742356128,-12.4166442993));
#51076=CARTESIAN_POINT('',(9.36397871523,-34.4242356128,-12.4166442993));
#51077=CARTESIAN_POINT('',(-0.24703583055,-32.5742356128,-3.04763757243));
#51078=CARTESIAN_POINT('Origin',(9.15456852675,-36.2742356128,-12.6314636954));
#51079=CARTESIAN_POINT('',(9.33061792149,-36.2742356128,-12.8743764588));
#51080=CARTESIAN_POINT('Origin',(9.27193478991,-36.2742356128,-12.7934055377));
#51081=CARTESIAN_POINT('Origin',(9.15456852675,-36.2742356128,-12.6314636954));
#51082=CARTESIAN_POINT('Origin',(9.15456852675,-34.4242356128,-12.6314636954));
#51083=CARTESIAN_POINT('',(9.33061792149,-32.5742356128,-12.8743764588));
#51084=CARTESIAN_POINT('',(9.33061792149,-34.4242356128,-12.8743764588));
#51085=CARTESIAN_POINT('Origin',(9.15456852675,-32.5742356128,-12.6314636954));
#51086=CARTESIAN_POINT('Origin',(-1.09995011675E-15,-34.4242356128,2.38806125834E-16));
#51087=CARTESIAN_POINT('',(-9.33061792149,-32.5742356128,-12.8743764588));
#51088=CARTESIAN_POINT('Origin',(1.12952603833E-15,-32.5742356128,-1.76411037141E-15));
#51089=CARTESIAN_POINT('',(-9.33061792149,-36.2742356128,-12.8743764588));
#51090=CARTESIAN_POINT('Origin',(-1.55306943244E-15,-36.2742356128,4.65365783676E-16));
#51091=CARTESIAN_POINT('',(-9.33061792149,-34.4242356128,-12.8743764588));
#51092=CARTESIAN_POINT('Origin',(1.99964424636E-15,-36.2742356128,2.24172262308E-15));
#51093=CARTESIAN_POINT('Origin',(-9.27193478991,-36.2742356128,-12.7934055377));
#51094=CARTESIAN_POINT('Origin',(-9.15456852675,-36.2742356128,-12.6314636954));
#51095=CARTESIAN_POINT('',(-9.36397871523,-36.2742356128,-12.4166442993));
#51096=CARTESIAN_POINT('Origin',(-9.29417531907,-36.2742356128,-12.4882507647));
#51097=CARTESIAN_POINT('Origin',(-9.15456852675,-36.2742356128,-12.6314636954));
#51098=CARTESIAN_POINT('Origin',(-9.15456852675,-34.4242356128,-12.6314636954));
#51099=CARTESIAN_POINT('',(-9.36397871523,-32.5742356128,-12.4166442993));
#51100=CARTESIAN_POINT('',(-9.36397871523,-34.4242356128,-12.4166442993));
#51101=CARTESIAN_POINT('Origin',(-9.15456852675,-32.5742356128,-12.6314636954));
#51102=CARTESIAN_POINT('Origin',(0.316839226711,-36.2742356128,-3.11924403781));
#51103=CARTESIAN_POINT('',(-8.19033423541,-36.2742356128,-11.2725524894));
#51104=CARTESIAN_POINT('Origin',(-8.12053083925,-36.2742356128,-11.3441589548));
#51105=CARTESIAN_POINT('',(-8.77715647532,-36.2742356128,-11.8445983944));
#51106=CARTESIAN_POINT('Origin',(-7.97551483927,-32.4742356128,-11.0631423009));
#51107=CARTESIAN_POINT('',(-8.19033423541,-32.5742356128,-11.2725524894));
#51108=CARTESIAN_POINT('',(-8.19033423541,-34.4242356128,-11.2725524894));
#51109=CARTESIAN_POINT('',(0.24703583055,-32.5742356128,-3.04763757243));
#51110=CARTESIAN_POINT('Origin',(-8.39974442389,-36.2742356128,-11.0577330933));
#51111=CARTESIAN_POINT('',(-8.18492502775,-36.2742356128,-10.8483229048));
#51112=CARTESIAN_POINT('Origin',(-8.11331856237,-36.2742356128,-10.7785195086));
#51113=CARTESIAN_POINT('Origin',(-8.39974442389,-36.2742356128,-11.0577330933));
#51114=CARTESIAN_POINT('Origin',(-8.39974442389,-34.4242356128,-11.0577330933));
#51115=CARTESIAN_POINT('',(-8.18492502775,-32.5742356128,-10.8483229048));
#51116=CARTESIAN_POINT('',(-8.18492502775,-34.4242356128,-10.8483229048));
#51117=CARTESIAN_POINT('Origin',(-8.39974442389,-32.5742356128,-11.0577330933));
#51118=CARTESIAN_POINT('Origin',(-8.43647932171,-36.2742356128,-10.447011287));
#51119=CARTESIAN_POINT('',(-11.1928713102,-36.2742356128,-7.76267932308));
#51120=CARTESIAN_POINT('Origin',(-11.1212648448,-36.2742356128,-7.69287592692));
#51121=CARTESIAN_POINT('',(-9.68889816899,-36.2742356128,-9.30550111394));
#51122=CARTESIAN_POINT('Origin',(-11.4022814987,-32.4742356128,-7.54785992694));
#51123=CARTESIAN_POINT('',(-11.1928713102,-32.5742356128,-7.76267932308));
#51124=CARTESIAN_POINT('',(-11.1928713102,-34.4242356128,-7.76267932308));
#51125=CARTESIAN_POINT('',(-8.50808578709,-32.5742356128,-10.5168146831));
#51126=CARTESIAN_POINT('Origin',(-11.4076907064,-36.2742356128,-7.97208951156));
#51127=CARTESIAN_POINT('',(-11.6171008949,-36.2742356128,-7.75727011542));
#51128=CARTESIAN_POINT('Origin',(-11.686904291,-36.2742356128,-7.68566365004));
#51129=CARTESIAN_POINT('Origin',(-11.4076907064,-36.2742356128,-7.97208951156));
#51130=CARTESIAN_POINT('Origin',(-11.4076907064,-34.4242356128,-7.97208951156));
#51131=CARTESIAN_POINT('',(-11.6171008949,-32.5742356128,-7.75727011542));
#51132=CARTESIAN_POINT('',(-11.6171008949,-34.4242356128,-7.75727011542));
#51133=CARTESIAN_POINT('Origin',(-11.4076907064,-32.5742356128,-7.97208951156));
#51134=CARTESIAN_POINT('Origin',(-0.45986885604,-36.2742356128,3.25867214427));
#51135=CARTESIAN_POINT('',(-12.7650943916,-36.2742356128,-8.87635684058));
#51136=CARTESIAN_POINT('Origin',(-12.8348977878,-36.2742356128,-8.80475037519));
#51137=CARTESIAN_POINT('',(-12.1910976432,-36.2742356128,-8.316813478));
#51138=CARTESIAN_POINT('Origin',(-11.4022814987,-32.4742356128,-7.54785992694));
#51139=CARTESIAN_POINT('',(-12.7650943916,-32.5742356128,-8.87635684058));
#51140=CARTESIAN_POINT('',(-12.7650943916,-34.4242356128,-8.87635684058));
#51141=CARTESIAN_POINT('',(-0.390065459879,-32.5742356128,3.18706567889));
#51142=CARTESIAN_POINT('Origin',(-12.9745045801,-36.2742356128,-8.66153744443));
#51143=CARTESIAN_POINT('',(-13.2240142836,-36.2742356128,-8.82810547221));
#51144=CARTESIAN_POINT('Origin',(-13.1408443824,-36.2742356128,-8.77258279628));
#51145=CARTESIAN_POINT('Origin',(-12.9745045801,-36.2742356128,-8.66153744443));
#51146=CARTESIAN_POINT('Origin',(-12.9745045801,-34.4242356128,-8.66153744443));
#51147=CARTESIAN_POINT('',(-13.2240142836,-32.5742356128,-8.82810547221));
#51148=CARTESIAN_POINT('',(-13.2240142836,-34.4242356128,-8.82810547221));
#51149=CARTESIAN_POINT('Origin',(-12.9745045801,-32.5742356128,-8.66153744443));
#51150=CARTESIAN_POINT('Origin',(5.55235792516E-15,-36.2742356128,2.24172262308E-15));
#51151=CARTESIAN_POINT('',(-14.1979138053,-36.2742356128,-7.15746069337));
#51152=CARTESIAN_POINT('Origin',(-14.1086187499,-36.2742356128,-7.11244521731));
#51153=CARTESIAN_POINT('Origin',(-1.55306943244E-15,-36.2742356128,4.65365783676E-16));
#51154=CARTESIAN_POINT('Origin',(-1.09995011675E-15,-34.4242356128,2.38806125834E-16));
#51155=CARTESIAN_POINT('',(-14.1979138053,-32.5742356128,-7.15746069337));
#51156=CARTESIAN_POINT('',(-14.1979138053,-34.4242356128,-7.15746069337));
#51157=CARTESIAN_POINT('Origin',(1.12952603833E-15,-32.5742356128,1.22464679915E-17));
#51158=CARTESIAN_POINT('Origin',(-13.7514385284,-36.2742356128,-6.93238331308));
#51159=CARTESIAN_POINT('',(-14.2514385284,-36.2742356128,-6.93238331308));
#51160=CARTESIAN_POINT('Origin',(-14.1514385284,-36.2742356128,-6.93238331308));
#51161=CARTESIAN_POINT('Origin',(-13.7514385284,-36.2742356128,-6.93238331308));
#51162=CARTESIAN_POINT('Origin',(-13.7514385284,-34.4242356128,-6.93238331308));
#51163=CARTESIAN_POINT('',(-14.2514385284,-32.5742356128,-6.93238331308));
#51164=CARTESIAN_POINT('',(-14.2514385284,-34.4242356128,-6.93238331308));
#51165=CARTESIAN_POINT('Origin',(-13.7514385284,-32.5742356128,-6.93238331308));
#51166=CARTESIAN_POINT('Origin',(-14.1514385284,-36.2742356128,-4.73378838547E-15));
#51167=CARTESIAN_POINT('',(-14.2514385284,-36.2742356128,6.93238331308));
#51168=CARTESIAN_POINT('Origin',(-14.1514385284,-36.2742356128,6.93238331308));
#51169=CARTESIAN_POINT('',(-14.2514385284,-36.2742356128,-1.7763568394E-15));
#51170=CARTESIAN_POINT('Origin',(-14.2514385284,-32.4742356128,7.05028367309));
#51171=CARTESIAN_POINT('',(-14.2514385284,-32.5742356128,6.93238331308));
#51172=CARTESIAN_POINT('',(-14.2514385284,-34.4242356128,6.93238331308));
#51173=CARTESIAN_POINT('',(-14.2514385284,-32.5742356128,-3.5527136788E-15));
#51174=CARTESIAN_POINT('Origin',(-13.7514385284,-36.2742356128,6.93238331308));
#51175=CARTESIAN_POINT('',(-14.1979138053,-36.2742356128,7.15746069337));
#51176=CARTESIAN_POINT('Origin',(-14.1086187499,-36.2742356128,7.11244521731));
#51177=CARTESIAN_POINT('Origin',(-13.7514385284,-36.2742356128,6.93238331308));
#51178=CARTESIAN_POINT('Origin',(-13.7514385284,-34.4242356128,6.93238331308));
#51179=CARTESIAN_POINT('',(-14.1979138053,-32.5742356128,7.15746069337));
#51180=CARTESIAN_POINT('',(-14.1979138053,-34.4242356128,7.15746069337));
#51181=CARTESIAN_POINT('Origin',(-13.7514385284,-32.5742356128,6.93238331308));
#51182=CARTESIAN_POINT('Origin',(5.79114658385E-12,-36.2742356128,-3.26980757555E-12));
#51183=CARTESIAN_POINT('',(-13.5056315679,-36.2742356128,8.39094249493));
#51184=CARTESIAN_POINT('Origin',(-13.4206904888,-36.2742356128,8.33816927169));
#51185=CARTESIAN_POINT('Origin',(-1.55306943244E-15,-36.2742356128,4.65365783676E-16));
#51186=CARTESIAN_POINT('Origin',(-1.09995011675E-15,-34.4242356128,2.38806125834E-16));
#51187=CARTESIAN_POINT('',(-13.5056315679,-32.5742356128,8.39094249493));
#51188=CARTESIAN_POINT('',(-13.5056315679,-34.4242356128,8.39094249493));
#51189=CARTESIAN_POINT('Origin',(6.95023748177E-12,-32.5742356128,-3.88843287498E-12));
#51190=CARTESIAN_POINT('Origin',(-13.2508083307,-36.2742356128,8.23262282521));
#51191=CARTESIAN_POINT('',(-13.0413981423,-36.2742356128,8.44744222135));
#51192=CARTESIAN_POINT('Origin',(-13.1112015384,-36.2742356128,8.37583575597));
#51193=CARTESIAN_POINT('Origin',(-13.2508083307,-36.2742356128,8.23262282521));
#51194=CARTESIAN_POINT('Origin',(-13.2508083307,-34.4242356128,8.23262282521));
#51195=CARTESIAN_POINT('',(-13.0413981423,-32.5742356128,8.44744222135));
#51196=CARTESIAN_POINT('',(-13.0413981423,-34.4242356128,8.44744222135));
#51197=CARTESIAN_POINT('Origin',(-13.2508083307,-32.5742356128,8.23262282521));
#51198=CARTESIAN_POINT('Origin',(-0.818017619209,-36.2742356128,-3.60780262944));
#51199=CARTESIAN_POINT('',(-11.9661178757,-36.2742356128,7.39923778851));
#51200=CARTESIAN_POINT('Origin',(-12.0359212718,-36.2742356128,7.32763132313));
#51201=CARTESIAN_POINT('',(-12.5283819332,-36.2742356128,7.94734389244));
#51202=CARTESIAN_POINT('Origin',(-11.7512984795,-32.4742356128,7.18982760003));
#51203=CARTESIAN_POINT('',(-11.9661178757,-32.5742356128,7.39923778851));
#51204=CARTESIAN_POINT('',(-11.9661178757,-34.4242356128,7.39923778851));
#51205=CARTESIAN_POINT('',(-0.748214223049,-32.5742356128,-3.53619616406));
#51206=CARTESIAN_POINT('Origin',(-11.7567076872,-36.2742356128,7.61405718465));
#51207=CARTESIAN_POINT('',(-11.541888291,-36.2742356128,7.40464699617));
#51208=CARTESIAN_POINT('Origin',(-11.4702818256,-36.2742356128,7.33484360001));
#51209=CARTESIAN_POINT('Origin',(-11.7567076872,-36.2742356128,7.61405718465));
#51210=CARTESIAN_POINT('Origin',(-11.7567076872,-34.4242356128,7.61405718465));
#51211=CARTESIAN_POINT('',(-11.541888291,-32.5742356128,7.40464699617));
#51212=CARTESIAN_POINT('',(-11.541888291,-34.4242356128,7.40464699617));
#51213=CARTESIAN_POINT('Origin',(-11.7567076872,-32.5742356128,7.61405718465));
#51214=CARTESIAN_POINT('Origin',(-8.43647932171,-36.2742356128,10.447011287));
#51215=CARTESIAN_POINT('',(-7.83590804694,-36.2742356128,11.2063552317));
#51216=CARTESIAN_POINT('Origin',(-7.76430158156,-36.2742356128,11.1365518355));
#51217=CARTESIAN_POINT('',(-9.68889816899,-36.2742356128,9.30550111394));
#51218=CARTESIAN_POINT('Origin',(-11.4022814987,-32.4742356128,7.54785992694));
#51219=CARTESIAN_POINT('',(-7.83590804694,-32.5742356128,11.2063552317));
#51220=CARTESIAN_POINT('',(-7.83590804694,-34.4242356128,11.2063552317));
#51221=CARTESIAN_POINT('',(-8.50808578709,-32.5742356128,10.5168146831));
#51222=CARTESIAN_POINT('Origin',(-8.73768936184,-36.2742356128,12.9233426255));
#51223=CARTESIAN_POINT('',(-8.94709955032,-36.2742356128,12.7085232294));
#51224=CARTESIAN_POINT('Origin',(-8.73768936184,-36.2742356128,12.9233426255));
#51225=CARTESIAN_POINT('Origin',(-8.87729615416,-36.2742356128,12.7801296947));
#51226=CARTESIAN_POINT('Origin',(-8.73768936184,-34.4242356128,12.9233426255));
#51227=CARTESIAN_POINT('',(-8.94709955032,-32.5742356128,12.7085232294));
#51228=CARTESIAN_POINT('Origin',(-8.73768936184,-32.5742356128,12.9233426255));
#51229=CARTESIAN_POINT('',(-8.94709955032,-34.4242356128,12.7085232294));
#51230=CARTESIAN_POINT('Origin',(-8.05072744309,-36.2742356128,11.4157654202));
#51231=CARTESIAN_POINT('',(-7.84131725461,-36.2742356128,11.6305848163));
#51232=CARTESIAN_POINT('Origin',(-7.77151385845,-36.2742356128,11.7021912817));
#51233=CARTESIAN_POINT('Origin',(-8.05072744309,-36.2742356128,11.4157654202));
#51234=CARTESIAN_POINT('Origin',(-8.05072744309,-34.4242356128,11.4157654202));
#51235=CARTESIAN_POINT('',(-7.84131725461,-32.5742356128,11.6305848163));
#51236=CARTESIAN_POINT('',(-7.84131725461,-34.4242356128,11.6305848163));
#51237=CARTESIAN_POINT('Origin',(-8.05072744309,-32.5742356128,11.4157654202));
#51238=CARTESIAN_POINT('Origin',(0.67498798988,-36.2742356128,3.46837452298));
#51239=CARTESIAN_POINT('',(-8.41710184852,-36.2742356128,12.191871006));
#51240=CARTESIAN_POINT('Origin',(-7.62649785846,-32.4742356128,11.4211746278));
#51241=CARTESIAN_POINT('',(0.60518459372,-32.5742356128,3.3967680576));
#51242=CARTESIAN_POINT('Origin',(-12.7514385284,-32.4742356128,7.05028367309));
#51243=CARTESIAN_POINT('',(-12.7514385284,-32.4742356128,6.07000095416));
#51244=CARTESIAN_POINT('',(-12.7514385284,-32.8742356128,6.07000095416));
#51245=CARTESIAN_POINT('',(-12.7514385284,-32.6742356128,6.07000095416));
#51246=CARTESIAN_POINT('',(-12.7514385284,-32.8742356128,-6.7682619245));
#51247=CARTESIAN_POINT('',(-12.7514385284,-32.8742356128,-5.3290705182E-15));
#51248=CARTESIAN_POINT('',(-12.7514385284,-32.4742356128,-6.7682619245));
#51249=CARTESIAN_POINT('',(-12.7514385284,-33.6742356128,-6.7682619245));
#51250=CARTESIAN_POINT('',(-12.7514385284,-32.4742356128,-0.349130485171));
#51251=CARTESIAN_POINT('Ctrl Pts',(-1.87043161103,-35.3742356128,-8.24476960824));
#51252=CARTESIAN_POINT('Ctrl Pts',(-0.881024471639,-32.4742356128,-9.12211895883));
#51253=CARTESIAN_POINT('Ctrl Pts',(-1.76698369017,-35.3742356128,-8.26339468616));
#51254=CARTESIAN_POINT('Ctrl Pts',(-0.751586859387,-32.4742356128,-9.0904082994));
#51255=CARTESIAN_POINT('Ctrl Pts',(-1.65525765665,-35.3742356128,-8.23673498884));
#51256=CARTESIAN_POINT('Ctrl Pts',(-0.632864708596,-32.4742356128,-9.01561057704));
#51257=CARTESIAN_POINT('Ctrl Pts',(-1.56310817921,-35.3742356128,-8.15928174403));
#51258=CARTESIAN_POINT('Ctrl Pts',(-0.544519454171,-32.4742356128,-8.90337130527));
#51259=CARTESIAN_POINT('Ctrl Pts',(-1.51727343488,-35.3742356128,-8.05439924541));
#51260=CARTESIAN_POINT('Ctrl Pts',(-0.500000005883,-32.4742356128,-8.76992589769));
#51261=CARTESIAN_POINT('Ctrl Pts',(-1.51727342606,-35.3742356128,-7.9495168227));
#51262=CARTESIAN_POINT('Ctrl Pts',(-0.5,-32.4742356128,-8.63648038577));
#51263=CARTESIAN_POINT('',(-1.46144760572984,-35.2150897285804,-7.9872159489329));
#51264=CARTESIAN_POINT('',(-0.5,-32.4742356128,-8.63648038577));
#51265=CARTESIAN_POINT('',(-1.461447583,-35.2150896638,-7.98721594967));
#51266=CARTESIAN_POINT('',(-0.881024471639,-32.4742356128,-9.12211895883));
#51267=CARTESIAN_POINT('Ctrl Pts',(-0.881024471639,-32.4742356128,-9.12211895883));
#51268=CARTESIAN_POINT('Ctrl Pts',(-0.827016089126107,-32.4742356128,-9.10888755418313));
#51269=CARTESIAN_POINT('Ctrl Pts',(-0.775540637915395,-32.4742356128,-9.08673032516009));
#51270=CARTESIAN_POINT('Ctrl Pts',(-0.682134270020785,-32.4742356128,-9.02649837726588));
#51271=CARTESIAN_POINT('Ctrl Pts',(-0.640813901103346,-32.4742356141908,
-8.98885840070038));
#51272=CARTESIAN_POINT('Ctrl Pts',(-0.57228055336198,-32.4742356141908,
-8.901510263898));
#51273=CARTESIAN_POINT('Ctrl Pts',(-0.545563385694432,-32.4742356128,-8.85244719394298));
#51274=CARTESIAN_POINT('Ctrl Pts',(-0.509276617611063,-32.4742356128,-8.74739553291418));
#51275=CARTESIAN_POINT('Ctrl Pts',(-0.500000002452142,-32.4742356128,-8.69210290609089));
#51276=CARTESIAN_POINT('Ctrl Pts',(-0.5,-32.4742356128,-8.63648038577));
#51277=CARTESIAN_POINT('',(-1.83110023521525,-35.2589537682581,-8.27964633186293));
#51278=CARTESIAN_POINT('',(-1.83110005118,-35.2589529157,-8.27964657357));
#51279=CARTESIAN_POINT('Ctrl Pts',(-1.46144762641058,-35.2150897875193,
-7.98721596760513));
#51280=CARTESIAN_POINT('Ctrl Pts',(-1.45999274413531,-35.2109422616504,
-8.00191902509857));
#51281=CARTESIAN_POINT('Ctrl Pts',(-1.45957341091662,-35.2071571950236,
-8.01670884221526));
#51282=CARTESIAN_POINT('Ctrl Pts',(-1.46026191644033,-35.203764095227,-8.03143220521763));
#51283=CARTESIAN_POINT('Ctrl Pts',(-1.46096768768079,-35.2002859063528,
-8.04652478735688));
#51284=CARTESIAN_POINT('Ctrl Pts',(-1.46283764504754,-35.1972195789501,
-8.06154670605974));
#51285=CARTESIAN_POINT('Ctrl Pts',(-1.46590012256396,-35.1945898968725,
-8.07630792772827));
#51286=CARTESIAN_POINT('Ctrl Pts',(-1.46903420709223,-35.1918987274289,
-8.0914142970654));
#51287=CARTESIAN_POINT('Ctrl Pts',(-1.47341730681797,-35.1896648446532,
-8.10624662772912));
#51288=CARTESIAN_POINT('Ctrl Pts',(-1.47902730659165,-35.1879077839919,
-8.1205895819562));
#51289=CARTESIAN_POINT('Ctrl Pts',(-1.48166047777195,-35.1870830706796,
-8.1273217486647));
#51290=CARTESIAN_POINT('Ctrl Pts',(-1.48456319805496,-35.1863633079977,
-8.13394603229644));
#51291=CARTESIAN_POINT('Ctrl Pts',(-1.48772926757142,-35.1857500185123,
-8.14044030456528));
#51292=CARTESIAN_POINT('Ctrl Pts',(-1.49433115834809,-35.1844711867696,
-8.15398216647638));
#51293=CARTESIAN_POINT('Ctrl Pts',(-1.5020813773099,-35.1836556215759,-8.16695799089605));
#51294=CARTESIAN_POINT('Ctrl Pts',(-1.51088863668741,-35.1833130708024,
-8.17917555169671));
#51295=CARTESIAN_POINT('Ctrl Pts',(-1.51677966584951,-35.1830839442933,
-8.18734767470132));
#51296=CARTESIAN_POINT('Ctrl Pts',(-1.52314264543556,-35.1830663220979,
-8.19518080428534));
#51297=CARTESIAN_POINT('Ctrl Pts',(-1.52993884840686,-35.18326173225,-8.20262371909327));
#51298=CARTESIAN_POINT('Ctrl Pts',(-1.5396630145576,-35.1835413296656,-8.21327321566418));
#51299=CARTESIAN_POINT('Ctrl Pts',(-1.55027411075703,-35.1842571031188,
-8.22312066676176));
#51300=CARTESIAN_POINT('Ctrl Pts',(-1.56163020662216,-35.1854101081919,
-8.23204589669893));
#51301=CARTESIAN_POINT('Ctrl Pts',(-1.56997721952966,-35.1862575955979,
-8.23860616268935));
#51302=CARTESIAN_POINT('Ctrl Pts',(-1.57872600240808,-35.1873412311022,
-8.24466874427926));
#51303=CARTESIAN_POINT('Ctrl Pts',(-1.58780845871722,-35.1886604340494,
-8.25019966634848));
#51304=CARTESIAN_POINT('Ctrl Pts',(-1.6005630488647,-35.1905130048013,-8.25796679912947));
#51305=CARTESIAN_POINT('Ctrl Pts',(-1.6139737807599,-35.1928321347006,-8.26468081127607));
#51306=CARTESIAN_POINT('Ctrl Pts',(-1.6278554617678,-35.1955968415854,-8.27028675557324));
#51307=CARTESIAN_POINT('Ctrl Pts',(-1.64227743897151,-35.1984691550787,
-8.27611089177209));
#51308=CARTESIAN_POINT('Ctrl Pts',(-1.65720660407866,-35.2018228868763,
-8.28073943848053));
#51309=CARTESIAN_POINT('Ctrl Pts',(-1.67243049904531,-35.2056328375554,
-8.28416822709316));
#51310=CARTESIAN_POINT('Ctrl Pts',(-1.68794439477149,-35.2095153641812,
-8.28766233087671));
#51311=CARTESIAN_POINT('Ctrl Pts',(-1.70376300691381,-35.2138722198964,
-8.28991123800377));
#51312=CARTESIAN_POINT('Ctrl Pts',(-1.71967583215399,-35.2186669738979,
-8.29096015927791));
#51313=CARTESIAN_POINT('Ctrl Pts',(-1.72516869832638,-35.2203220503323,
-8.29132223100918));
#51314=CARTESIAN_POINT('Ctrl Pts',(-1.73067300845718,-35.2220291797313,
-8.29154169905675));
#51315=CARTESIAN_POINT('Ctrl Pts',(-1.73618094824065,-35.2237864091028,
-8.29162151774592));
#51316=CARTESIAN_POINT('Ctrl Pts',(-1.75076469988551,-35.2284391463775,
-8.2918328591885));
#51317=CARTESIAN_POINT('Ctrl Pts',(-1.76537892989469,-35.2334500139743,
-8.29106239128857));
#51318=CARTESIAN_POINT('Ctrl Pts',(-1.77988835203768,-35.2387691032084,
-8.28937964173054));
#51319=CARTESIAN_POINT('Ctrl Pts',(-1.79299811300231,-35.2435750829173,
-8.28785921974187));
#51320=CARTESIAN_POINT('Ctrl Pts',(-1.8060221558571,-35.2486326175861,-8.28559474347183));
#51321=CARTESIAN_POINT('Ctrl Pts',(-1.81889037024243,-35.2538888283575,
-8.28265208359663));
#51322=CARTESIAN_POINT('Ctrl Pts',(-1.82241578493209,-35.2553288356585,
-8.28184590365277));
#51323=CARTESIAN_POINT('Ctrl Pts',(-1.82592932282104,-35.2567834218319,
-8.28098898477275));
#51324=CARTESIAN_POINT('Ctrl Pts',(-1.82942950902499,-35.2582510471779,
-8.28008297427468));
#51325=CARTESIAN_POINT('Ctrl Pts',(-1.82998637759462,-35.258484541735,-8.27993883086609));
#51326=CARTESIAN_POINT('Ctrl Pts',(-1.83054294259533,-35.2587183799279,
-8.27979343760619));
#51327=CARTESIAN_POINT('Ctrl Pts',(-1.83110005096932,-35.2589529154682,
-8.27964657215517));
#51328=CARTESIAN_POINT('Origin',(-1.51727342606,-35.3742356128,-6.62635333853281));
#51329=CARTESIAN_POINT('',(-1.46090316329,-35.2135376551,-5.30645216923));
#51330=CARTESIAN_POINT('',(-0.5,-32.4742356128,-5.26505293156));
#51331=CARTESIAN_POINT('',(-1.46090316329,-35.2135376551,-5.30645216923));
#51332=CARTESIAN_POINT('',(-0.5,-32.4742356128,-5.26505293156));
#51333=CARTESIAN_POINT('',(-1.46090089616294,-35.2135311920909,-7.94951678979554));
#51334=CARTESIAN_POINT('Origin',(-2.99786357884902,-39.5950398533888,-7.94865516340226));
#51335=CARTESIAN_POINT('',(-1.46090316329,-35.2135376551,-5.30645216923));
#51336=CARTESIAN_POINT('Ctrl Pts',(-2.06618662358,-35.3742356128,-8.20763292551));
#51337=CARTESIAN_POINT('Ctrl Pts',(-1.13092983125,-32.4742356128,-9.11903336658));
#51338=CARTESIAN_POINT('Ctrl Pts',(-2.02728693019,-35.3742356128,-8.21539237438));
#51339=CARTESIAN_POINT('Ctrl Pts',(-1.08254865919,-32.4742356128,-9.13216050293));
#51340=CARTESIAN_POINT('Ctrl Pts',(-1.98835267261,-35.3742356128,-8.22296816028));
#51341=CARTESIAN_POINT('Ctrl Pts',(-1.03251986746,-32.4742356128,-9.13922496193));
#51342=CARTESIAN_POINT('Ctrl Pts',(-1.94830447917,-35.3742356128,-8.23056358523));
#51343=CARTESIAN_POINT('Ctrl Pts',(-0.980045978296,-32.4742356128,-9.13989363405));
#51344=CARTESIAN_POINT('Ctrl Pts',(-1.90939289225,-35.3742356128,-8.23775490438));
#51345=CARTESIAN_POINT('Ctrl Pts',(-0.929775106566,-32.4742356128,-9.13406227499));
#51346=CARTESIAN_POINT('Ctrl Pts',(-1.87043161103,-35.3742356128,-8.24476960824));
#51347=CARTESIAN_POINT('Ctrl Pts',(-0.881024471639,-32.4742356128,-9.12211895883));
#51348=CARTESIAN_POINT('',(-1.13092983125,-32.4742356128,-9.11903336658));
#51349=CARTESIAN_POINT('Ctrl Pts',(-0.881024471639,-32.4742356128,-9.12211895883));
#51350=CARTESIAN_POINT('Ctrl Pts',(-0.92220301191105,-32.4742356128,-9.13220720334646));
#51351=CARTESIAN_POINT('Ctrl Pts',(-0.964264740457436,-32.474235612914,
-9.13687601377793));
#51352=CARTESIAN_POINT('Ctrl Pts',(-1.04807641455819,-32.474235612914,-9.13584112130989));
#51353=CARTESIAN_POINT('Ctrl Pts',(-1.09001172345298,-32.4742356128,-9.13013556930401));
#51354=CARTESIAN_POINT('Ctrl Pts',(-1.13092983125,-32.4742356128,-9.11903336658));
#51355=CARTESIAN_POINT('',(-2.02882224805641,-35.258377357075,-8.24404435912867));
#51356=CARTESIAN_POINT('',(-2.02882173043,-35.2583763205,-8.24404472212));
#51357=CARTESIAN_POINT('',(-1.88461534275654,-35.2526204926692,-8.27242221793694));
#51358=CARTESIAN_POINT('Ctrl Pts',(-1.88461534316216,-35.2526204924197,
-8.27242222025263));
#51359=CARTESIAN_POINT('Ctrl Pts',(-1.91265386025649,-35.2529892698862,
-8.26755066673147));
#51360=CARTESIAN_POINT('Ctrl Pts',(-1.94082131994964,-35.2537157453151,
-8.26234408725425));
#51361=CARTESIAN_POINT('Ctrl Pts',(-1.96909946479954,-35.2548039079099,
-8.25679923395567));
#51362=CARTESIAN_POINT('Ctrl Pts',(-1.99780133897712,-35.2563733143722,
-8.2508227750941));
#51363=CARTESIAN_POINT('Ctrl Pts',(-2.02658489036,-35.258233098,-8.24453400819));
#51364=CARTESIAN_POINT('Ctrl Pts',(-2.02732982489,-35.2582811474,-8.24437112291));
#51365=CARTESIAN_POINT('Ctrl Pts',(-2.02807537275,-35.2583289394,-8.24420802987));
#51366=CARTESIAN_POINT('Ctrl Pts',(-2.02882173043,-35.2583763205,-8.24404472212));
#51367=CARTESIAN_POINT('Origin',(-1.87243909403022,-35.4444729230294,-8.21860710030529));
#51368=CARTESIAN_POINT('Ctrl Pts',(-8.90408048591,-35.3742356128,-3.33175685019));
#51369=CARTESIAN_POINT('Ctrl Pts',(-9.78972512979,-32.4742356128,-2.88747118331));
#51370=CARTESIAN_POINT('Ctrl Pts',(-8.6873937464,-35.3742356128,-3.78156218415));
#51371=CARTESIAN_POINT('Ctrl Pts',(-9.44154892618,-32.4742356128,-3.40960230403));
#51372=CARTESIAN_POINT('Ctrl Pts',(-8.41228804471,-35.3742356128,-4.20311089247));
#51373=CARTESIAN_POINT('Ctrl Pts',(-9.06633060557,-32.4742356128,-3.9138589137));
#51374=CARTESIAN_POINT('Ctrl Pts',(-8.09063109224,-35.3742356128,-4.59678365893));
#51375=CARTESIAN_POINT('Ctrl Pts',(-8.6592141531,-32.4742356128,-4.40538764451));
#51376=CARTESIAN_POINT('Ctrl Pts',(-7.360622472,-35.3742356128,-5.38465519647));
#51377=CARTESIAN_POINT('Ctrl Pts',(-7.74414150515,-32.4742356128,-5.40001779324));
#51378=CARTESIAN_POINT('Ctrl Pts',(-6.54392160985,-35.3742356128,-6.08248533528));
#51379=CARTESIAN_POINT('Ctrl Pts',(-6.72376489891,-32.4742356128,-6.28784412471));
#51380=CARTESIAN_POINT('Ctrl Pts',(-6.08996440487,-35.3742356128,-6.43395446983));
#51381=CARTESIAN_POINT('Ctrl Pts',(-6.15045388192,-32.4742356128,-6.72961730824));
#51382=CARTESIAN_POINT('Ctrl Pts',(-5.07098217764,-35.3742356128,-7.12903795521));
#51383=CARTESIAN_POINT('Ctrl Pts',(-4.8659622122,-32.4742356128,-7.60280558321));
#51384=CARTESIAN_POINT('Ctrl Pts',(-3.96068628695,-35.3742356128,-7.66774624913));
#51385=CARTESIAN_POINT('Ctrl Pts',(-3.47975995949,-32.4742356128,-8.30623076748));
#51386=CARTESIAN_POINT('Ctrl Pts',(-3.34362139801,-35.3742356128,-7.90067576649));
#51387=CARTESIAN_POINT('Ctrl Pts',(-2.71614717835,-32.4742356128,-8.63027694049));
#51388=CARTESIAN_POINT('Ctrl Pts',(-2.70966555084,-35.3742356128,-8.07927608136));
#51389=CARTESIAN_POINT('Ctrl Pts',(-1.93124535238,-32.4742356128,-8.90188586102));
#51390=CARTESIAN_POINT('Ctrl Pts',(-2.06618662358,-35.3742356128,-8.20763292551));
#51391=CARTESIAN_POINT('Ctrl Pts',(-1.13092983125,-32.4742356128,-9.11903336658));
#51392=CARTESIAN_POINT('',(-9.78972512979,-32.4742356128,-2.88747118331));
#51393=CARTESIAN_POINT('Ctrl Pts',(-1.13092983125,-32.4742356128,-9.11903336658));
#51394=CARTESIAN_POINT('Ctrl Pts',(-1.35748096440087,-32.4742356128002,
-9.05756384343984));
#51395=CARTESIAN_POINT('Ctrl Pts',(-1.58257164660585,-32.4742356128003,
-8.99085150410091));
#51396=CARTESIAN_POINT('Ctrl Pts',(-1.80593829563056,-32.4742356128004,
-8.91898444731663));
#51397=CARTESIAN_POINT('Ctrl Pts',(-2.06358605409587,-32.4742356128005,
-8.83608762199012));
#51398=CARTESIAN_POINT('Ctrl Pts',(-2.31894092044636,-32.4742356128005,
-8.74633156326516));
#51399=CARTESIAN_POINT('Ctrl Pts',(-2.57167018297851,-32.4742356128005,
-8.6498360378973));
#51400=CARTESIAN_POINT('Ctrl Pts',(-2.87961762633398,-32.4742356128005,
-8.53225744792893));
#51401=CARTESIAN_POINT('Ctrl Pts',(-3.18367140744747,-32.4742356128005,
-8.40466930268279));
#51402=CARTESIAN_POINT('Ctrl Pts',(-3.48328763307677,-32.4742356128004,
-8.26730091093105));
#51403=CARTESIAN_POINT('Ctrl Pts',(-3.71568832582298,-32.4742356128003,
-8.16074957400834));
#51404=CARTESIAN_POINT('Ctrl Pts',(-3.94542176433015,-32.4742356128003,
-8.0483135945673));
#51405=CARTESIAN_POINT('Ctrl Pts',(-4.17221459820387,-32.4742356128002,
-7.93012756314153));
#51406=CARTESIAN_POINT('Ctrl Pts',(-4.3691051862723,-32.4742356128002,-7.82752415706631));
#51407=CARTESIAN_POINT('Ctrl Pts',(-4.56378009094538,-32.4742356128001,
-7.72058696590365));
#51408=CARTESIAN_POINT('Ctrl Pts',(-4.75602733655703,-32.4742356128001,
-7.60942955096299));
#51409=CARTESIAN_POINT('Ctrl Pts',(-4.81482808842437,-32.4742356128001,
-7.57543093863777));
#51410=CARTESIAN_POINT('Ctrl Pts',(-4.87340144129883,-32.4742356128001,
-7.54103772494405));
#51411=CARTESIAN_POINT('Ctrl Pts',(-4.93174048144869,-32.4742356128001,
-7.50625373162201));
#51412=CARTESIAN_POINT('Ctrl Pts',(-5.17371609272893,-32.4742356128,-7.36197850828535));
#51413=CARTESIAN_POINT('Ctrl Pts',(-5.41165903155182,-32.4742356128,-7.21097959772054));
#51414=CARTESIAN_POINT('Ctrl Pts',(-5.64521361977431,-32.4742356128,-7.0534854983882));
#51415=CARTESIAN_POINT('Ctrl Pts',(-5.92854786582719,-32.4742356128,-6.86242321940786));
#51416=CARTESIAN_POINT('Ctrl Pts',(-6.20541886627958,-32.4742356128,-6.66180293529635));
#51417=CARTESIAN_POINT('Ctrl Pts',(-6.47520523011177,-32.4742356128,-6.45207607376425));
#51418=CARTESIAN_POINT('Ctrl Pts',(-6.7042174903774,-32.4742356128001,-6.27404623594872));
#51419=CARTESIAN_POINT('Ctrl Pts',(-6.92812568553406,-32.4742356128001,
-6.08945471655604));
#51420=CARTESIAN_POINT('Ctrl Pts',(-7.14656401932481,-32.4742356128001,
-5.89860434351618));
#51421=CARTESIAN_POINT('Ctrl Pts',(-7.30145174556248,-32.4742356128002,
-5.76327836927544));
#51422=CARTESIAN_POINT('Ctrl Pts',(-7.4535896236381,-32.4742356128002,-5.62480608682023));
#51423=CARTESIAN_POINT('Ctrl Pts',(-7.60284952378423,-32.4742356128003,
-5.48330473081067));
#51424=CARTESIAN_POINT('Ctrl Pts',(-7.66409102798865,-32.4742356128003,
-5.42524656595522));
#51425=CARTESIAN_POINT('Ctrl Pts',(-7.72484844931582,-32.4742356128003,
-5.36667817449847));
#51426=CARTESIAN_POINT('Ctrl Pts',(-7.78511221664714,-32.4742356128003,
-5.30760881482714));
#51427=CARTESIAN_POINT('Ctrl Pts',(-7.86083082414573,-32.4742356128003,
-5.23339092473813));
#51428=CARTESIAN_POINT('Ctrl Pts',(-7.9357705171939,-32.4742356128004,-5.1583808441567));
#51429=CARTESIAN_POINT('Ctrl Pts',(-8.00994285087825,-32.4742356128004,
-5.08255688170474));
#51430=CARTESIAN_POINT('Ctrl Pts',(-8.09229096248547,-32.4742356128004,
-4.99837508759984));
#51431=CARTESIAN_POINT('Ctrl Pts',(-8.17369314495629,-32.4742356128004,
-4.91319009037416));
#51432=CARTESIAN_POINT('Ctrl Pts',(-8.25412492760548,-32.4742356128004,
-4.82702704996663));
#51433=CARTESIAN_POINT('Ctrl Pts',(-8.31333790947206,-32.4742356128004,
-4.76359478002089));
#51434=CARTESIAN_POINT('Ctrl Pts',(-8.37202401218054,-32.4742356128004,
-4.69963371548019));
#51435=CARTESIAN_POINT('Ctrl Pts',(-8.43016285000587,-32.4742356128004,
-4.63516899165583));
#51436=CARTESIAN_POINT('Ctrl Pts',(-8.45791646133128,-32.4742356128004,
-4.60439560580666));
#51437=CARTESIAN_POINT('Ctrl Pts',(-8.48554521988306,-32.4742356128004,
-4.57350770746612));
#51438=CARTESIAN_POINT('Ctrl Pts',(-8.51305689825755,-32.4742356128004,
-4.54249677272974));
#51439=CARTESIAN_POINT('Ctrl Pts',(-8.62342507636421,-32.4742356128004,
-4.41809068155457));
#51440=CARTESIAN_POINT('Ctrl Pts',(-8.7318733436495,-32.4742356128004,-4.29174315144362));
#51441=CARTESIAN_POINT('Ctrl Pts',(-8.8382486463566,-32.4742356128004,-4.16363335145393));
#51442=CARTESIAN_POINT('Ctrl Pts',(-8.93277342320662,-32.4742356128004,
-4.04979536511541));
#51443=CARTESIAN_POINT('Ctrl Pts',(-9.02565819435723,-32.4742356128005,
-3.93456977982075));
#51444=CARTESIAN_POINT('Ctrl Pts',(-9.11679326953606,-32.4742356128005,
-3.81808802140576));
#51445=CARTESIAN_POINT('Ctrl Pts',(-9.19450142462868,-32.4742356128005,
-3.7187675069868));
#51446=CARTESIAN_POINT('Ctrl Pts',(-9.2709365589139,-32.4742356128005,-3.61853483930442));
#51447=CARTESIAN_POINT('Ctrl Pts',(-9.34605185297795,-32.4742356128005,
-3.51744756155323));
#51448=CARTESIAN_POINT('Ctrl Pts',(-9.41503263776077,-32.4742356128005,
-3.42461587078078));
#51449=CARTESIAN_POINT('Ctrl Pts',(-9.48289988060696,-32.4742356128004,
-3.33106404763001));
#51450=CARTESIAN_POINT('Ctrl Pts',(-9.54964545463381,-32.4742356128004,
-3.23680385237855));
#51451=CARTESIAN_POINT('Ctrl Pts',(-9.6112390224299,-32.4742356128003,-3.14981948208372));
#51452=CARTESIAN_POINT('Ctrl Pts',(-9.67187720579196,-32.4742356128002,
-3.0622321188807));
#51453=CARTESIAN_POINT('Ctrl Pts',(-9.73158294374893,-32.4742356128001,
-2.97401646795334));
#51454=CARTESIAN_POINT('Ctrl Pts',(-9.75106213192314,-32.4742356128001,
-2.94523582938955));
#51455=CARTESIAN_POINT('Ctrl Pts',(-9.77044232827666,-32.4742356128,-2.91638800950429));
#51456=CARTESIAN_POINT('Ctrl Pts',(-9.78972512979,-32.4742356128,-2.88747118331));
#51457=CARTESIAN_POINT('',(-8.93444612284907,-35.274804900368,-3.31652382194753));
#51458=CARTESIAN_POINT('',(-8.93444623808,-35.2748044449,-3.31652380097));
#51459=CARTESIAN_POINT('Ctrl Pts',(-2.02882232648753,-35.2583763371521,
-8.24404459697176));
#51460=CARTESIAN_POINT('Ctrl Pts',(-2.76037088316413,-35.278813606438,-8.09044863214831));
#51461=CARTESIAN_POINT('Ctrl Pts',(-3.46770779566994,-35.2977417662847,
-7.87807502189995));
#51462=CARTESIAN_POINT('Ctrl Pts',(-4.14485661336304,-35.3130519325903,
-7.60417976937799));
#51463=CARTESIAN_POINT('Ctrl Pts',(-5.21843933075938,-35.3262967397835,
-7.04499008624918));
#51464=CARTESIAN_POINT('Ctrl Pts',(-6.21090480851,-35.3291957718,-6.34191684905));
#51465=CARTESIAN_POINT('Ctrl Pts',(-6.59524089295,-35.3292320711,-6.04038307893));
#51466=CARTESIAN_POINT('Ctrl Pts',(-7.36674621113887,-35.3292429117998,
-5.37908304420829));
#51467=CARTESIAN_POINT('Ctrl Pts',(-8.06644389763777,-35.3242511580814,
-4.63577834525724));
#51468=CARTESIAN_POINT('Ctrl Pts',(-8.40676936045737,-35.3182542216342,
-4.22563367825667));
#51469=CARTESIAN_POINT('Ctrl Pts',(-8.69862023264536,-35.3007569336673,
-3.78649459696414));
#51470=CARTESIAN_POINT('Ctrl Pts',(-8.93444619651196,-35.2748044494745,
-3.31652388380974));
#51471=CARTESIAN_POINT('Ctrl Pts',(-8.98669828191,-35.3742356128,-3.15062625521));
#51472=CARTESIAN_POINT('Ctrl Pts',(-9.87176476169,-32.4742356128,-2.65438916225));
#51473=CARTESIAN_POINT('Ctrl Pts',(-8.97105229548,-35.3742356128,-3.18695239061));
#51474=CARTESIAN_POINT('Ctrl Pts',(-9.86736571705,-32.4742356128,-2.70382530588));
#51475=CARTESIAN_POINT('Ctrl Pts',(-8.95501903475,-35.3742356128,-3.22311199053));
#51476=CARTESIAN_POINT('Ctrl Pts',(-9.85683264819,-32.4742356128,-2.75271530399));
#51477=CARTESIAN_POINT('Ctrl Pts',(-8.93801024352,-35.3742356128,-3.26038797601));
#51478=CARTESIAN_POINT('Ctrl Pts',(-9.83970156009,-32.4742356128,-2.80141079064));
#51479=CARTESIAN_POINT('Ctrl Pts',(-8.92122822926,-35.3742356128,-3.29616101079));
#51480=CARTESIAN_POINT('Ctrl Pts',(-9.81727888481,-32.4742356128,-2.84615108413));
#51481=CARTESIAN_POINT('Ctrl Pts',(-8.90408048591,-35.3742356128,-3.33175685019));
#51482=CARTESIAN_POINT('Ctrl Pts',(-9.78972512979,-32.4742356128,-2.88747118331));
#51483=CARTESIAN_POINT('Ctrl Pts',(-9.78972512979,-32.4742356128,-2.88747118331));
#51484=CARTESIAN_POINT('Ctrl Pts',(-9.81295258958151,-32.4742356128,-2.85263887310081));
#51485=CARTESIAN_POINT('Ctrl Pts',(-9.83153874678994,-32.4742356128027,
-2.81516874991383));
#51486=CARTESIAN_POINT('Ctrl Pts',(-9.85907250391396,-32.4742356128027,
-2.7369427829564));
#51487=CARTESIAN_POINT('Ctrl Pts',(-9.86805391767536,-32.4742356128,-2.69609135731934));
#51488=CARTESIAN_POINT('Ctrl Pts',(-9.87176476169,-32.4742356128,-2.65438916225));
#51489=CARTESIAN_POINT('Ctrl Pts',(-8.93444605304206,-35.2748053537063,
-3.31652375104877));
#51490=CARTESIAN_POINT('Ctrl Pts',(-8.93943078683952,-35.2740356286657,
-3.30669402651363));
#51491=CARTESIAN_POINT('Ctrl Pts',(-8.94434451549187,-35.2733172975681,
-3.29686734543151));
#51492=CARTESIAN_POINT('Ctrl Pts',(-8.94920331673012,-35.272662843585,-3.28699914163946));
#51493=CARTESIAN_POINT('Ctrl Pts',(-8.95476993132043,-35.2719130510102,
-3.27569337206476));
#51494=CARTESIAN_POINT('Ctrl Pts',(-8.96026410692822,-35.2712477134621,
-3.26433342692446));
#51495=CARTESIAN_POINT('Ctrl Pts',(-8.96568233550565,-35.2706790956147,
-3.25291618430066));
#51496=CARTESIAN_POINT('Ctrl Pts',(-8.97215912488461,-35.2699993867427,
-3.23926835185764));
#51497=CARTESIAN_POINT('Ctrl Pts',(-8.97852587883437,-35.2694597776266,
-3.22554062845691));
#51498=CARTESIAN_POINT('Ctrl Pts',(-8.98475365565657,-35.2690516336245,
-3.21179689045617));
#51499=CARTESIAN_POINT('Ctrl Pts',(-8.98837874704945,-35.2688140593904,
-3.203796875723));
#51500=CARTESIAN_POINT('Ctrl Pts',(-8.99195645868942,-35.2686203376525,
-3.19579252489701));
#51501=CARTESIAN_POINT('Ctrl Pts',(-8.99548252093106,-35.2684610193862,
-3.18779854474187));
#51502=CARTESIAN_POINT('Ctrl Pts',(-8.99854073311971,-35.2683228400148,
-3.18086523333927));
#51503=CARTESIAN_POINT('Ctrl Pts',(-9.00156177291394,-35.2682167859986,
-3.17393229744647));
#51504=CARTESIAN_POINT('Ctrl Pts',(-9.00454520265064,-35.2681414577284,
-3.1670013767672));
#51505=CARTESIAN_POINT('Ctrl Pts',(-9.00705208603224,-35.2680781617218,
-3.16117753930374));
#51506=CARTESIAN_POINT('Ctrl Pts',(-9.00953172445309,-35.2680334238437,
-3.15535857579231));
#51507=CARTESIAN_POINT('Ctrl Pts',(-9.01198468982812,-35.2680064936339,
-3.14954401027304));
#51508=CARTESIAN_POINT('Ctrl Pts',(-9.01387857125029,-35.2679857014023,
-3.14505471020912));
#51509=CARTESIAN_POINT('Ctrl Pts',(-9.01575650600665,-35.2679752542737,
-3.14056830801862));
#51510=CARTESIAN_POINT('Ctrl Pts',(-9.01762235287468,-35.2679892318977,
-3.1360680066287));
#51511=CARTESIAN_POINT('Ctrl Pts',(-9.01812186455268,-35.267992973891,-3.13486321692313));
#51512=CARTESIAN_POINT('Ctrl Pts',(-9.01862041750448,-35.2679978846909,
-3.13365798589397));
#51513=CARTESIAN_POINT('Ctrl Pts',(-9.01911868766448,-35.2680072166355,
-3.13244884927113));
#51514=CARTESIAN_POINT('Ctrl Pts',(-3.51985615629,-35.3742356128,-3.20601908088));
#51515=CARTESIAN_POINT('Ctrl Pts',(-3.1350457731,-32.4742356128,-2.57376246377));
#51516=CARTESIAN_POINT('Ctrl Pts',(-3.5389561844,-35.3742356128,-3.1668368061));
#51517=CARTESIAN_POINT('Ctrl Pts',(-3.17276903042,-32.4742356128,-2.53334077836));
#51518=CARTESIAN_POINT('Ctrl Pts',(-3.56517269185,-35.3742356128,-3.13112318899));
#51519=CARTESIAN_POINT('Ctrl Pts',(-3.21038331308,-32.4742356128,-2.49281798697));
#51520=CARTESIAN_POINT('Ctrl Pts',(-3.59940527056,-35.3742356128,-3.09917422736));
#51521=CARTESIAN_POINT('Ctrl Pts',(-3.24932685202,-32.4742356128,-2.45063230102));
#51522=CARTESIAN_POINT('Ctrl Pts',(-3.63699355357,-35.3742356128,-3.07546800882));
#51523=CARTESIAN_POINT('Ctrl Pts',(-3.28665002885,-32.4742356128,-2.40998048911));
#51524=CARTESIAN_POINT('Ctrl Pts',(-3.67755401867,-35.3742356128,-3.05915055738));
#51525=CARTESIAN_POINT('Ctrl Pts',(-3.32386409198,-32.4742356128,-2.36922853848));
#51526=CARTESIAN_POINT('',(-3.66207294828794,-35.2473021021,-3.02895254909137));
#51527=CARTESIAN_POINT('',(-3.32386409198,-32.4742356128,-2.36922853848));
#51528=CARTESIAN_POINT('',(-3.66207294829203,-35.247302102094,-3.02895254911367));
#51529=CARTESIAN_POINT('',(-3.1350457731,-32.4742356128,-2.57376246377));
#51530=CARTESIAN_POINT('Origin',(15.769898679409,-32.4742355606854,15.0680202722476));
#51531=CARTESIAN_POINT('',(-3.50597898793362,-35.2696545343368,-3.18321829788018));
#51532=CARTESIAN_POINT('',(-3.50597895501,-35.2696545374,-3.18321836469));
#51533=CARTESIAN_POINT('Ctrl Pts',(-3.66207294827955,-35.2473021021057,
-3.02895254907185));
#51534=CARTESIAN_POINT('Ctrl Pts',(-3.66091495179321,-35.2473795704993,
-3.02947323796857));
#51535=CARTESIAN_POINT('Ctrl Pts',(-3.65976226369913,-35.2474575947881,
-3.0300000109274));
#51536=CARTESIAN_POINT('Ctrl Pts',(-3.65861281967912,-35.2475362729335,
-3.03053380228582));
#51537=CARTESIAN_POINT('Ctrl Pts',(-3.65240605310862,-35.2479611190979,
-3.03341616828313));
#51538=CARTESIAN_POINT('Ctrl Pts',(-3.6463111786709,-35.2484032769964,-3.03649530323666));
#51539=CARTESIAN_POINT('Ctrl Pts',(-3.64031422873348,-35.248862763431,-3.03977928431773));
#51540=CARTESIAN_POINT('Ctrl Pts',(-3.6322888734286,-35.2494776663289,-3.04417403752813));
#51541=CARTESIAN_POINT('Ctrl Pts',(-3.62443677559274,-35.2501213489573,
-3.04893623763928));
#51542=CARTESIAN_POINT('Ctrl Pts',(-3.61676784831451,-35.2508052779905,
-3.05406683233371));
#51543=CARTESIAN_POINT('Ctrl Pts',(-3.60730204981363,-35.2516494553026,
-3.06039955317002));
#51544=CARTESIAN_POINT('Ctrl Pts',(-3.59811807272275,-35.2525562450447,
-3.06729452529451));
#51545=CARTESIAN_POINT('Ctrl Pts',(-3.58929693635001,-35.2535534756824,
-3.0747059316244));
#51546=CARTESIAN_POINT('Ctrl Pts',(-3.58809950408998,-35.2536888455583,
-3.0757119989446));
#51547=CARTESIAN_POINT('Ctrl Pts',(-3.58690878465367,-35.2538258680597,
-3.07672751152805));
#51548=CARTESIAN_POINT('Ctrl Pts',(-3.58572498566927,-35.253964593268,-3.07775228998077));
#51549=CARTESIAN_POINT('Ctrl Pts',(-3.57769765100733,-35.2549052881722,
-3.08470130725703));
#51550=CARTESIAN_POINT('Ctrl Pts',(-3.56999072711075,-35.2559268700649,
-3.09207839837468));
#51551=CARTESIAN_POINT('Ctrl Pts',(-3.56268644817232,-35.2570395958347,
-3.09981180666564));
#51552=CARTESIAN_POINT('Ctrl Pts',(-3.55508194090727,-35.2581980580555,
-3.10786308181927));
#51553=CARTESIAN_POINT('Ctrl Pts',(-3.54791482463172,-35.2594544673558,
-3.11629765460186));
#51554=CARTESIAN_POINT('Ctrl Pts',(-3.54124405919227,-35.2607842073526,
-3.12502681208725));
#51555=CARTESIAN_POINT('Ctrl Pts',(-3.54078309233966,-35.2608760957674,
-3.12563001906379));
#51556=CARTESIAN_POINT('Ctrl Pts',(-3.54032447922608,-35.2609683237252,
-3.1262346405582));
#51557=CARTESIAN_POINT('Ctrl Pts',(-3.53986823173921,-35.2610608787453,
-3.12684065180599));
#51558=CARTESIAN_POINT('Ctrl Pts',(-3.53401616594948,-35.262248037212,-3.13461366490414));
#51559=CARTESIAN_POINT('Ctrl Pts',(-3.5285556873506,-35.263490013451,-3.1426127338717));
#51560=CARTESIAN_POINT('Ctrl Pts',(-3.52349535751664,-35.2647552260756,
-3.15080332732354));
#51561=CARTESIAN_POINT('Ctrl Pts',(-3.51892135499415,-35.2658988443625,
-3.15820675681106));
#51562=CARTESIAN_POINT('Ctrl Pts',(-3.51467414707485,-35.2670609744409,
-3.16576608898576));
#51563=CARTESIAN_POINT('Ctrl Pts',(-3.51073522720237,-35.2682166399343,
-3.1734916718749));
#51564=CARTESIAN_POINT('Ctrl Pts',(-3.50940929552838,-35.2686056637103,
-3.1760922820382));
#51565=CARTESIAN_POINT('Ctrl Pts',(-3.50811808179657,-35.2689939686856,
-3.17871208941865));
#51566=CARTESIAN_POINT('Ctrl Pts',(-3.50686019645209,-35.2693806830338,
-3.18135268706089));
#51567=CARTESIAN_POINT('Ctrl Pts',(-3.50656455234841,-35.269471573525,-3.18197331367565));
#51568=CARTESIAN_POINT('Ctrl Pts',(-3.50627078919946,-35.2695623867448,
-3.1825950147686));
#51569=CARTESIAN_POINT('Ctrl Pts',(-3.50597901251073,-35.2696545195266,
-3.18321824197148));
#51570=CARTESIAN_POINT('Ctrl Pts',(-7.21384189758,-35.3742356128,2.18958432614));
#51571=CARTESIAN_POINT('Ctrl Pts',(-7.92659403983,-32.4742356128,4.74000601033));
#51572=CARTESIAN_POINT('Ctrl Pts',(-7.26623945249,-35.3742356128,2.28696407666));
#51573=CARTESIAN_POINT('Ctrl Pts',(-7.98210778857,-32.4742356128,4.86805404157));
#51574=CARTESIAN_POINT('Ctrl Pts',(-7.33077888815,-35.3742356128,2.37781046265));
#51575=CARTESIAN_POINT('Ctrl Pts',(-8.06503365985,-32.4742356128,4.98421786182));
#51576=CARTESIAN_POINT('Ctrl Pts',(-7.40436869293,-35.3742356128,2.46126398331));
#51577=CARTESIAN_POINT('Ctrl Pts',(-8.17216612273,-32.4742356128,5.0807589417));
#51578=CARTESIAN_POINT('Ctrl Pts',(-7.56704033307,-35.3742356128,2.61160417272));
#51579=CARTESIAN_POINT('Ctrl Pts',(-8.41851793763,-32.4742356128,5.22052728604));
#51580=CARTESIAN_POINT('Ctrl Pts',(-7.76385631892,-35.3742356128,2.71310420624));
#51581=CARTESIAN_POINT('Ctrl Pts',(-8.70021558456,-32.4742356128,5.24806936162));
#51582=CARTESIAN_POINT('Ctrl Pts',(-7.87246551919,-35.3742356128,2.74929666995));
#51583=CARTESIAN_POINT('Ctrl Pts',(-8.84211900681,-32.4742356128,5.23137961658));
#51584=CARTESIAN_POINT('Ctrl Pts',(-8.09632446877,-35.3742356128,2.75144961057));
#51585=CARTESIAN_POINT('Ctrl Pts',(-9.10596900702,-32.4742356128,5.14052628192));
#51586=CARTESIAN_POINT('Ctrl Pts',(-8.29201770973,-35.3742356128,2.64306639111));
#51587=CARTESIAN_POINT('Ctrl Pts',(-9.31107389815,-32.4742356128,4.95155477014));
#51588=CARTESIAN_POINT('Ctrl Pts',(-8.37411601908,-35.3742356128,2.57138954697));
#51589=CARTESIAN_POINT('Ctrl Pts',(-9.39185739171,-32.4742356128,4.83723274541));
#51590=CARTESIAN_POINT('Ctrl Pts',(-8.4486251678,-35.3742356128,2.49348119172));
#51591=CARTESIAN_POINT('Ctrl Pts',(-9.44632201614,-32.4742356128,4.7098382487));
#51592=CARTESIAN_POINT('Ctrl Pts',(-8.51721509197,-35.3742356128,2.41066261776));
#51593=CARTESIAN_POINT('Ctrl Pts',(-9.47312185748,-32.4742356128,4.57687569684));
#51594=CARTESIAN_POINT('',(-8.6009108248196,-35.120322107747,2.60032839187079));
#51595=CARTESIAN_POINT('',(-9.47312185748,-32.4742356128,4.57687569684));
#51596=CARTESIAN_POINT('',(-8.60091083126,-35.1203221009,2.60032840073));
#51597=CARTESIAN_POINT('',(-7.92659403983,-32.4742356128,4.74000601033));
#51598=CARTESIAN_POINT('Ctrl Pts',(-9.47312185748,-32.4742356128,4.57687569684));
#51599=CARTESIAN_POINT('Ctrl Pts',(-9.46576357172862,-32.4742356128,4.61338249695149));
#51600=CARTESIAN_POINT('Ctrl Pts',(-9.45589852782759,-32.4742356128,4.64938312384879));
#51601=CARTESIAN_POINT('Ctrl Pts',(-9.4436151767327,-32.4742356128001,4.68454468695718));
#51602=CARTESIAN_POINT('Ctrl Pts',(-9.43116790267184,-32.4742356128001,
4.72017548583586));
#51603=CARTESIAN_POINT('Ctrl Pts',(-9.41623764589746,-32.4742356128001,
4.75494407050594));
#51604=CARTESIAN_POINT('Ctrl Pts',(-9.39896958249035,-32.4742356128001,
4.78851518953424));
#51605=CARTESIAN_POINT('Ctrl Pts',(-9.38152489595556,-32.4742356128002,
4.82242968441788));
#51606=CARTESIAN_POINT('Ctrl Pts',(-9.36169469208315,-32.4742356128002,
4.85512144315062));
#51607=CARTESIAN_POINT('Ctrl Pts',(-9.33967747672362,-32.4742356128002,
4.88626565542905));
#51608=CARTESIAN_POINT('Ctrl Pts',(-9.32473727646168,-32.4742356128002,
4.90739915305088));
#51609=CARTESIAN_POINT('Ctrl Pts',(-9.30879106644691,-32.4742356128002,
4.92782051201125));
#51610=CARTESIAN_POINT('Ctrl Pts',(-9.29191215925214,-32.4742356128002,
4.94743594307661));
#51611=CARTESIAN_POINT('Ctrl Pts',(-9.26807208685844,-32.4742356128001,
4.97514113105093));
#51612=CARTESIAN_POINT('Ctrl Pts',(-9.2423551960503,-32.4742356128002,5.00125358349318));
#51613=CARTESIAN_POINT('Ctrl Pts',(-9.21499925935546,-32.4742356128004,
5.02552229400269));
#51614=CARTESIAN_POINT('Ctrl Pts',(-9.18812489694226,-32.4742356128005,
5.04936377780233));
#51615=CARTESIAN_POINT('Ctrl Pts',(-9.15966921110771,-32.4742356128007,
5.07142540239296));
#51616=CARTESIAN_POINT('Ctrl Pts',(-9.12988757458161,-32.4742356128009,
5.09150932334396));
#51617=CARTESIAN_POINT('Ctrl Pts',(-9.1177306388397,-32.474235612801,5.09970762823674));
#51618=CARTESIAN_POINT('Ctrl Pts',(-9.10535306806464,-32.474235612801,5.1075768984626));
#51619=CARTESIAN_POINT('Ctrl Pts',(-9.09277339742187,-32.4742356128011,
5.11510591129192));
#51620=CARTESIAN_POINT('Ctrl Pts',(-9.06401134948185,-32.4742356128012,
5.13232017978011));
#51621=CARTESIAN_POINT('Ctrl Pts',(-9.03418916029184,-32.4742356128013,
5.1477537113724));
#51622=CARTESIAN_POINT('Ctrl Pts',(-9.00352034950314,-32.4742356128012,
5.1612883287322));
#51623=CARTESIAN_POINT('Ctrl Pts',(-8.98613398992056,-32.4742356128012,
5.16896119631913));
#51624=CARTESIAN_POINT('Ctrl Pts',(-8.9684764199063,-32.4742356128011,5.17602435236192));
#51625=CARTESIAN_POINT('Ctrl Pts',(-8.95059220546224,-32.474235612801,5.1824608849134));
#51626=CARTESIAN_POINT('Ctrl Pts',(-8.91460611802292,-32.4742356128007,
5.19541228537485));
#51627=CARTESIAN_POINT('Ctrl Pts',(-8.8776867278997,-32.4742356128005,5.20582893332123));
#51628=CARTESIAN_POINT('Ctrl Pts',(-8.84020622755982,-32.4742356128004,
5.21361149973278));
#51629=CARTESIAN_POINT('Ctrl Pts',(-8.80212100914067,-32.4742356128002,
5.22151963166691));
#51630=CARTESIAN_POINT('Ctrl Pts',(-8.76345811848754,-32.4742356128002,
5.22670768415973));
#51631=CARTESIAN_POINT('Ctrl Pts',(-8.72463030839696,-32.4742356128002,
5.22912100680538));
#51632=CARTESIAN_POINT('Ctrl Pts',(-8.68739236868495,-32.4742356128002,
5.23143551187209));
#51633=CARTESIAN_POINT('Ctrl Pts',(-8.65000425691521,-32.4742356128002,
5.23119800092422));
#51634=CARTESIAN_POINT('Ctrl Pts',(-8.6128267026259,-32.4742356128003,5.22840604118267));
#51635=CARTESIAN_POINT('Ctrl Pts',(-8.58737790569537,-32.4742356128003,
5.22649488758855));
#51636=CARTESIAN_POINT('Ctrl Pts',(-8.56202769486349,-32.4742356128004,
5.22338772754605));
#51637=CARTESIAN_POINT('Ctrl Pts',(-8.53688547477249,-32.4742356128005,
5.21909660544825));
#51638=CARTESIAN_POINT('Ctrl Pts',(-8.50390469579943,-32.4742356128006,
5.21346764551782));
#51639=CARTESIAN_POINT('Ctrl Pts',(-8.47128746528097,-32.4742356128007,
5.20580045842078));
#51640=CARTESIAN_POINT('Ctrl Pts',(-8.4392653732531,-32.4742356128007,5.19615646079357));
#51641=CARTESIAN_POINT('Ctrl Pts',(-8.43597511948344,-32.4742356128007,
5.19516554491213));
#51642=CARTESIAN_POINT('Ctrl Pts',(-8.43269111740371,-32.4742356128007,
5.19415379222059));
#51643=CARTESIAN_POINT('Ctrl Pts',(-8.42941359545578,-32.4742356128007,
5.19312129233961));
#51644=CARTESIAN_POINT('Ctrl Pts',(-8.3944144019285,-32.4742356128007,5.18209568710319));
#51645=CARTESIAN_POINT('Ctrl Pts',(-8.36015521648491,-32.4742356128006,
5.16869999519598));
#51646=CARTESIAN_POINT('Ctrl Pts',(-8.32695087107122,-32.4742356128006,
5.15305321371686));
#51647=CARTESIAN_POINT('Ctrl Pts',(-8.29319095413242,-32.4742356128005,
5.13714463197815));
#51648=CARTESIAN_POINT('Ctrl Pts',(-8.26052202447813,-32.4742356128004,
5.11890928463567));
#51649=CARTESIAN_POINT('Ctrl Pts',(-8.22925624736326,-32.4742356128004,
5.09852305936231));
#51650=CARTESIAN_POINT('Ctrl Pts',(-8.20513847568554,-32.4742356128003,
5.08279754821614));
#51651=CARTESIAN_POINT('Ctrl Pts',(-8.18185530346072,-32.4742356128002,
5.06579330067018));
#51652=CARTESIAN_POINT('Ctrl Pts',(-8.15953944897647,-32.4742356128002,
5.04760937719499));
#51653=CARTESIAN_POINT('Ctrl Pts',(-8.13000306159537,-32.4742356128001,
5.02354185120129));
#51654=CARTESIAN_POINT('Ctrl Pts',(-8.1021534308539,-32.4742356128001,4.99739923287759));
#51655=CARTESIAN_POINT('Ctrl Pts',(-8.07626720330521,-32.4742356128001,
4.96943994770265));
#51656=CARTESIAN_POINT('Ctrl Pts',(-8.0505351356036,-32.4742356128,4.94164716802253));
#51657=CARTESIAN_POINT('Ctrl Pts',(-8.0267436078806,-32.4742356128,4.91205976688404));
#51658=CARTESIAN_POINT('Ctrl Pts',(-8.00512575620472,-32.4742356128,4.88096523499291));
#51659=CARTESIAN_POINT('Ctrl Pts',(-7.98386071885989,-32.4742356128,4.85037818167243));
#51660=CARTESIAN_POINT('Ctrl Pts',(-7.96469932551459,-32.4742356128,4.81833327235114));
#51661=CARTESIAN_POINT('Ctrl Pts',(-7.94782028391973,-32.4742356128,4.78512968374919));
#51662=CARTESIAN_POINT('Ctrl Pts',(-7.94028653932774,-32.4742356128,4.77030968614097));
#51663=CARTESIAN_POINT('Ctrl Pts',(-7.93320686704621,-32.4742356128,4.75525915977829));
#51664=CARTESIAN_POINT('Ctrl Pts',(-7.92659403983,-32.4742356128,4.74000601033));
#51665=CARTESIAN_POINT('',(-7.23545016824,-35.2863172732,2.26690461571));
#51666=CARTESIAN_POINT('',(-7.23545016824,-35.2863172732,2.26690461571));
#51667=CARTESIAN_POINT('Ctrl Pts',(-8.60091083126,-35.1203221009,2.60032840073));
#51668=CARTESIAN_POINT('Ctrl Pts',(-8.56160117875,-35.1140346808,2.66060541831));
#51669=CARTESIAN_POINT('Ctrl Pts',(-8.51829161967,-35.1086508497,2.71924356476));
#51670=CARTESIAN_POINT('Ctrl Pts',(-8.47165311425,-35.1035435988,2.77475885702));
#51671=CARTESIAN_POINT('Ctrl Pts',(-8.35159188251,-35.0922845623,2.89275323394));
#51672=CARTESIAN_POINT('Ctrl Pts',(-8.20219946581,-35.0869079403,2.96964215712));
#51673=CARTESIAN_POINT('Ctrl Pts',(-8.10597427981,-35.0887550559,2.98941073315));
#51674=CARTESIAN_POINT('Ctrl Pts',(-7.82075728158,-35.1140008873,2.95981413055));
#51675=CARTESIAN_POINT('Ctrl Pts',(-7.56538653659,-35.1573736159,2.76989788484));
#51676=CARTESIAN_POINT('Ctrl Pts',(-7.43180190579,-35.1865123729,2.62065670169));
#51677=CARTESIAN_POINT('Ctrl Pts',(-7.32065041948,-35.231204862,2.4495725015));
#51678=CARTESIAN_POINT('Ctrl Pts',(-7.23545016824,-35.2863172732,2.26690461571));
#51679=CARTESIAN_POINT('Ctrl Pts',(-8.51721509197,-35.3742356128,2.41066261776));
#51680=CARTESIAN_POINT('Ctrl Pts',(-9.47312185748,-32.4742356128,4.57687569684));
#51681=CARTESIAN_POINT('Ctrl Pts',(-8.57124548357,-35.3742356128,2.34542388422));
#51682=CARTESIAN_POINT('Ctrl Pts',(-9.49423281845,-32.4742356128,4.47213748961));
#51683=CARTESIAN_POINT('Ctrl Pts',(-8.62160287869,-35.3742356128,2.27713826199));
#51684=CARTESIAN_POINT('Ctrl Pts',(-9.51478914505,-32.4742356128,4.367292468));
#51685=CARTESIAN_POINT('Ctrl Pts',(-8.66952448488,-35.3742356128,2.20708948255));
#51686=CARTESIAN_POINT('Ctrl Pts',(-9.53482564259,-32.4742356128,4.26215510362));
#51687=CARTESIAN_POINT('Ctrl Pts',(-8.71540499967,-35.3742356128,2.13579061508));
#51688=CARTESIAN_POINT('Ctrl Pts',(-9.55426490812,-32.4742356128,4.15713558997));
#51689=CARTESIAN_POINT('Ctrl Pts',(-8.75956299023,-35.3742356128,2.0634404101));
#51690=CARTESIAN_POINT('Ctrl Pts',(-9.5731487029,-32.4742356128,4.05201631342));
#51691=CARTESIAN_POINT('',(-8.82321718811955,-35.1473420531381,2.21902512680689));
#51692=CARTESIAN_POINT('',(-9.5731487029,-32.4742356128,4.05201631342));
#51693=CARTESIAN_POINT('',(-8.82321723512,-35.1473421125,2.21902487472));
#51694=CARTESIAN_POINT('Origin',(15.3007564523972,-32.4742356010378,-0.416450801703818));
#51695=CARTESIAN_POINT('Ctrl Pts',(-8.8232168869647,-35.1473420700646,2.219025543263));
#51696=CARTESIAN_POINT('Ctrl Pts',(-8.80526362682125,-35.145153271855,2.25350258409433));
#51697=CARTESIAN_POINT('Ctrl Pts',(-8.78684682703311,-35.1429249882693,
2.28803306323546));
#51698=CARTESIAN_POINT('Ctrl Pts',(-8.76791345287321,-35.1406440769323,
2.32254344633434));
#51699=CARTESIAN_POINT('Ctrl Pts',(-8.75132900856273,-35.138646142136,2.35277237023366));
#51700=CARTESIAN_POINT('Ctrl Pts',(-8.73434636716193,-35.1366097977285,
2.38298586372834));
#51701=CARTESIAN_POINT('Ctrl Pts',(-8.71692245297776,-35.1345191813108,
2.41310198813675));
#51702=CARTESIAN_POINT('Ctrl Pts',(-8.70215559144233,-35.1327473725865,
2.43862556650279));
#51703=CARTESIAN_POINT('Ctrl Pts',(-8.68707123431251,-35.1309370177603,
2.46407888932811));
#51704=CARTESIAN_POINT('Ctrl Pts',(-8.67165070386463,-35.1290601449782,
2.489389823811));
#51705=CARTESIAN_POINT('Ctrl Pts',(-8.66337872647115,-35.1280533411412,
2.50296727359835));
#51706=CARTESIAN_POINT('Ctrl Pts',(-8.65500395568259,-35.1270312044469,
2.51650713409901));
#51707=CARTESIAN_POINT('Ctrl Pts',(-8.64651908034742,-35.1259916049772,
2.52999652004439));
#51708=CARTESIAN_POINT('Ctrl Pts',(-8.63865177225743,-35.125027672215,2.54250408803862));
#51709=CARTESIAN_POINT('Ctrl Pts',(-8.63069362675025,-35.1240461475895,
2.55496615938241));
#51710=CARTESIAN_POINT('Ctrl Pts',(-8.62264312140985,-35.123042269789,2.56736795085125));
#51711=CARTESIAN_POINT('Ctrl Pts',(-8.61689703694199,-35.1223257474848,
2.57621978540321));
#51712=CARTESIAN_POINT('Ctrl Pts',(-8.61110407596,-35.1215977157902,2.58504077148982));
#51713=CARTESIAN_POINT('Ctrl Pts',(-8.60525029211926,-35.1208654219131,
2.59383214904833));
#51714=CARTESIAN_POINT('Ctrl Pts',(-8.60380709913618,-35.1206848820411,
2.59599957694612));
#51715=CARTESIAN_POINT('Ctrl Pts',(-8.60236297383733,-35.1205021342156,
2.59816380216256));
#51716=CARTESIAN_POINT('Ctrl Pts',(-8.60091081515229,-35.1203221010069,
2.60032838482467));
#51717=CARTESIAN_POINT('Ctrl Pts',(-8.75956299023,-35.3742356128,2.0634404101));
#51718=CARTESIAN_POINT('Ctrl Pts',(-9.5731487029,-32.4742356128,4.05201631342));
#51719=CARTESIAN_POINT('Ctrl Pts',(-8.92885481093,-35.3742356128,1.78606749512));
#51720=CARTESIAN_POINT('Ctrl Pts',(-9.64554465255,-32.4742356128,3.6490141658));
#51721=CARTESIAN_POINT('Ctrl Pts',(-9.07282740405,-35.3742356128,1.49324081294));
#51722=CARTESIAN_POINT('Ctrl Pts',(-9.70977650917,-32.4742356128,3.24454541193));
#51723=CARTESIAN_POINT('Ctrl Pts',(-9.12664920772,-35.3742356128,1.15116500779));
#51724=CARTESIAN_POINT('Ctrl Pts',(-9.76784884218,-32.4742356128,2.82302310552));
#51725=CARTESIAN_POINT('Ctrl Pts',(-9.18659879637,-35.3742356128,0.831334347991));
#51726=CARTESIAN_POINT('Ctrl Pts',(-9.8153632788,-32.4742356128,2.41643837733));
#51727=CARTESIAN_POINT('Ctrl Pts',(-9.23698117862,-35.3742356128,0.509886547138));
#51728=CARTESIAN_POINT('Ctrl Pts',(-9.85462053301,-32.4742356128,2.00920484002));
#51729=CARTESIAN_POINT('Ctrl Pts',(-9.5731487029,-32.4742356128,4.05201631342));
#51730=CARTESIAN_POINT('Ctrl Pts',(-9.58385803994689,-32.4742356128002,
3.99240129558575));
#51731=CARTESIAN_POINT('Ctrl Pts',(-9.5943536855861,-32.4742356128003,3.93274277792962));
#51732=CARTESIAN_POINT('Ctrl Pts',(-9.60464591256779,-32.4742356128005,
3.87295958919005));
#51733=CARTESIAN_POINT('Ctrl Pts',(-9.61549552175361,-32.4742356128006,
3.80993880322598));
#51734=CARTESIAN_POINT('Ctrl Pts',(-9.62611903415597,-32.4742356128007,
3.74677981964133));
#51735=CARTESIAN_POINT('Ctrl Pts',(-9.63652068269621,-32.4742356128008,
3.6834457777419));
#51736=CARTESIAN_POINT('Ctrl Pts',(-9.64770872862421,-32.4742356128009,
3.61532348281569));
#51737=CARTESIAN_POINT('Ctrl Pts',(-9.65864002597334,-32.4742356128009,
3.54699913843106));
#51738=CARTESIAN_POINT('Ctrl Pts',(-9.66931194496843,-32.4742356128009,
3.47848631183152));
#51739=CARTESIAN_POINT('Ctrl Pts',(-9.68148004640578,-32.474235612801,3.40036811919844));
#51740=CARTESIAN_POINT('Ctrl Pts',(-9.69331083177811,-32.474235612801,3.32200562453741));
#51741=CARTESIAN_POINT('Ctrl Pts',(-9.70479179824442,-32.4742356128009,
3.24348485468347));
#51742=CARTESIAN_POINT('Ctrl Pts',(-9.7201856722383,-32.4742356128009,3.13820287859019));
#51743=CARTESIAN_POINT('Ctrl Pts',(-9.73495007583227,-32.4742356128008,
3.03264005645671));
#51744=CARTESIAN_POINT('Ctrl Pts',(-9.74904466851698,-32.4742356128007,
2.92708814611483));
#51745=CARTESIAN_POINT('Ctrl Pts',(-9.75943548222614,-32.4742356128006,
2.84927318107526));
#51746=CARTESIAN_POINT('Ctrl Pts',(-9.7694618745955,-32.4742356128006,2.77146717702854));
#51747=CARTESIAN_POINT('Ctrl Pts',(-9.77911025980369,-32.4742356128005,
2.6937724200985));
#51748=CARTESIAN_POINT('Ctrl Pts',(-9.78779970867891,-32.4742356128004,
2.62379961079945));
#51749=CARTESIAN_POINT('Ctrl Pts',(-9.79618242234148,-32.4742356128003,
2.55391804485843));
#51750=CARTESIAN_POINT('Ctrl Pts',(-9.80425367824051,-32.4742356128003,
2.48416708378499));
#51751=CARTESIAN_POINT('Ctrl Pts',(-9.81180034779321,-32.4742356128002,
2.41894954381487));
#51752=CARTESIAN_POINT('Ctrl Pts',(-9.81907464790267,-32.4742356128002,
2.3538467998227));
#51753=CARTESIAN_POINT('Ctrl Pts',(-9.8260789591149,-32.4742356128001,2.28884751742815));
#51754=CARTESIAN_POINT('Ctrl Pts',(-9.83260578437975,-32.4742356128001,
2.22827925515725));
#51755=CARTESIAN_POINT('Ctrl Pts',(-9.83889814477805,-32.4742356128,2.16780107633691));
#51756=CARTESIAN_POINT('Ctrl Pts',(-9.84496431448896,-32.4742356128,2.10735907911607));
#51757=CARTESIAN_POINT('Ctrl Pts',(-9.84824849657925,-32.4742356128,2.07463620220455));
#51758=CARTESIAN_POINT('Ctrl Pts',(-9.85146649575577,-32.4742356128,2.041923117793));
#51759=CARTESIAN_POINT('Ctrl Pts',(-9.85462053301,-32.4742356128,2.00920484002));
#51760=CARTESIAN_POINT('',(-8.84972910932056,-35.1509197094744,2.16703888406964));
#51761=CARTESIAN_POINT('Ctrl Pts',(-8.84972757036633,-35.1509188455761,
2.16704273318452));
#51762=CARTESIAN_POINT('Ctrl Pts',(-8.84263701355718,-35.1498854734004,
2.18123269435607));
#51763=CARTESIAN_POINT('Ctrl Pts',(-8.83539046048538,-35.1488785397256,
2.19550438840577));
#51764=CARTESIAN_POINT('Ctrl Pts',(-8.82797601093741,-35.1479357210167,
2.20985097691311));
#51765=CARTESIAN_POINT('Ctrl Pts',(-8.82639727975385,-35.1477349701333,
2.2129057426793));
#51766=CARTESIAN_POINT('Ctrl Pts',(-8.82481106154748,-35.1475370463719,
2.21596377869292));
#51767=CARTESIAN_POINT('Ctrl Pts',(-8.82321740410989,-35.1473422016281,
2.21902486252055));
#51768=CARTESIAN_POINT('Ctrl Pts',(-9.26569102913818,-35.2394341100243,
0.579580104582361));
#51769=CARTESIAN_POINT('Ctrl Pts',(-9.26432897936841,-35.2391993937044,
0.588916840903954));
#51770=CARTESIAN_POINT('Ctrl Pts',(-9.26295526781442,-35.2389720582188,
0.598255150960743));
#51771=CARTESIAN_POINT('Ctrl Pts',(-9.26157088200535,-35.2387502154634,
0.607597401941648));
#51772=CARTESIAN_POINT('Ctrl Pts',(-9.25606802654771,-35.2378684030313,
0.644732322322909));
#51773=CARTESIAN_POINT('Ctrl Pts',(-9.25039903101778,-35.2370737660972,
0.681935582958867));
#51774=CARTESIAN_POINT('Ctrl Pts',(-9.24459515278581,-35.2362958421616,
0.719269900919489));
#51775=CARTESIAN_POINT('Ctrl Pts',(-9.23860144043817,-35.2354924737738,
0.757825355325635));
#51776=CARTESIAN_POINT('Ctrl Pts',(-9.23246358621943,-35.2347066278465,
0.796520371533143));
#51777=CARTESIAN_POINT('Ctrl Pts',(-9.22617547021298,-35.2338649909902,
0.835383081090787));
#51778=CARTESIAN_POINT('Ctrl Pts',(-9.21950775230034,-35.2329725460771,
0.876591860379445));
#51779=CARTESIAN_POINT('Ctrl Pts',(-9.21267081123946,-35.2320169111237,
0.917989042641703));
#51780=CARTESIAN_POINT('Ctrl Pts',(-9.20561664949873,-35.2309214566663,
0.959565403305954));
#51781=CARTESIAN_POINT('Ctrl Pts',(-9.20129161992591,-35.2302498144361,
0.985056595032471));
#51782=CARTESIAN_POINT('Ctrl Pts',(-9.19688415582833,-35.2295258515741,
1.0106143158295));
#51783=CARTESIAN_POINT('Ctrl Pts',(-9.19237714642468,-35.2287349082349,
1.0362297220611));
#51784=CARTESIAN_POINT('Ctrl Pts',(-9.18433806879567,-35.2273241157706,
1.08191949564519));
#51785=CARTESIAN_POINT('Ctrl Pts',(-9.17598329873894,-35.2256969838539,
1.12779875063943));
#51786=CARTESIAN_POINT('Ctrl Pts',(-9.16718884329799,-35.2237950554676,
1.17378828861314));
#51787=CARTESIAN_POINT('Ctrl Pts',(-9.15824445275229,-35.2218607014429,
1.22056189403028));
#51788=CARTESIAN_POINT('Ctrl Pts',(-9.14884412978376,-35.2196413404115,
1.26744866220585));
#51789=CARTESIAN_POINT('Ctrl Pts',(-9.13883756774077,-35.2171160563015,
1.31433550967857));
#51790=CARTESIAN_POINT('Ctrl Pts',(-9.12913301134297,-35.2146669871847,
1.35980727647108));
#51791=CARTESIAN_POINT('Ctrl Pts',(-9.11885715887533,-35.2119298210439,
1.40527813132619));
#51792=CARTESIAN_POINT('Ctrl Pts',(-9.10787101160138,-35.2089310791387,
1.4506315207492));
#51793=CARTESIAN_POINT('Ctrl Pts',(-9.10306272832524,-35.2076186262657,
1.47048124044086));
#51794=CARTESIAN_POINT('Ctrl Pts',(-9.09811845693115,-35.2062566994767,
1.49030836911984));
#51795=CARTESIAN_POINT('Ctrl Pts',(-9.09302722159328,-35.2048506613808,
1.51010300502406));
#51796=CARTESIAN_POINT('Ctrl Pts',(-9.08137976609742,-35.201634002739,1.55538811275342));
#51797=CARTESIAN_POINT('Ctrl Pts',(-9.0689621044373,-35.1981822931679,1.60050286270257));
#51798=CARTESIAN_POINT('Ctrl Pts',(-9.05566818026723,-35.1945757132466,
1.64531873653687));
#51799=CARTESIAN_POINT('Ctrl Pts',(-9.04311114502703,-35.1911690478716,
1.68765044385356));
#51800=CARTESIAN_POINT('Ctrl Pts',(-9.02977099290996,-35.1876254879663,
1.72971514826849));
#51801=CARTESIAN_POINT('Ctrl Pts',(-9.01559361637142,-35.1840385572175,
1.77140429309896));
#51802=CARTESIAN_POINT('Ctrl Pts',(-9.00271099223959,-35.1807792038035,
1.80928616650255));
#51803=CARTESIAN_POINT('Ctrl Pts',(-8.98913667424359,-35.1774848505479,
1.84685777318515));
#51804=CARTESIAN_POINT('Ctrl Pts',(-8.97487070089677,-35.1742336894979,
1.88404080636593));
#51805=CARTESIAN_POINT('Ctrl Pts',(-8.96340477304722,-35.1716206481638,
1.91392576165875));
#51806=CARTESIAN_POINT('Ctrl Pts',(-8.95149260611499,-35.1690357681137,
1.94355972733414));
#51807=CARTESIAN_POINT('Ctrl Pts',(-8.93915874000816,-35.1665192378142,
1.97290476540593));
#51808=CARTESIAN_POINT('Ctrl Pts',(-8.92511135651658,-35.1636530913943,
2.00632664625004));
#51809=CARTESIAN_POINT('Ctrl Pts',(-8.9105144674308,-35.1608758193711,2.03937607228335));
#51810=CARTESIAN_POINT('Ctrl Pts',(-8.89544878975767,-35.1582413753976,
2.07199872308543));
#51811=CARTESIAN_POINT('Ctrl Pts',(-8.8938366780672,-35.1579594751725,2.07548952900025));
#51812=CARTESIAN_POINT('Ctrl Pts',(-8.8922192469323,-35.15767920151,2.07897545514641));
#51813=CARTESIAN_POINT('Ctrl Pts',(-8.89059663078593,-35.1574006136199,
2.08245644010738));
#51814=CARTESIAN_POINT('Ctrl Pts',(-8.87729309257504,-35.155116521569,2.11099641029262));
#51815=CARTESIAN_POINT('Ctrl Pts',(-8.8636443139379,-35.1529474030868,2.13919120126784));
#51816=CARTESIAN_POINT('Ctrl Pts',(-8.84973117353,-35.1509193731,2.1670354781));
#51817=CARTESIAN_POINT('Origin',(12.4493324411,-32.4742356128,-6.47376294621));
#51818=CARTESIAN_POINT('',(12.4493324411,-32.4742356128,-6.47376294621));
#51819=CARTESIAN_POINT('',(12.4493324411,-32.8742356128,-6.47376294621));
#51820=CARTESIAN_POINT('',(12.4493324411,-32.6742356128,-6.47376294621));
#51821=CARTESIAN_POINT('',(12.4493324411,-32.8742356128,-6.47376294621));
#51822=CARTESIAN_POINT('',(12.6003854848,-32.4742356128,-6.62101243536));
#51823=CARTESIAN_POINT('Origin',(-12.4493324411,-32.4742356128,-6.47376294621));
#51824=CARTESIAN_POINT('',(-12.4493324411,-32.4742356128,-6.47376294621));
#51825=CARTESIAN_POINT('',(-12.6003854848,-32.4742356128,-6.62101243536));
#51826=CARTESIAN_POINT('',(-12.4493324411,-32.8742356128,-6.47376294621));
#51827=CARTESIAN_POINT('',(-12.7514385284,-32.8742356128,-6.7682619245));
#51828=CARTESIAN_POINT('',(-12.4493324411,-32.6742356128,-6.47376294621));
#51829=CARTESIAN_POINT('Ctrl Pts',(3.48890306473,-35.2652540838,-3.21461371005));
#51830=CARTESIAN_POINT('Ctrl Pts',(3.49935367494,-35.3079501575,-3.21504790568));
#51831=CARTESIAN_POINT('Ctrl Pts',(3.50770783242,-35.351170349,-3.21440294636));
#51832=CARTESIAN_POINT('Ctrl Pts',(3.51392345177,-35.3947427768,-3.21267707712));
#51833=CARTESIAN_POINT('Ctrl Pts',(3.51797541026,-35.4384913267,-3.20987727374));
#51834=CARTESIAN_POINT('Ctrl Pts',(3.51985615043,-35.4822398766,-3.20601907528));
#51835=CARTESIAN_POINT('Ctrl Pts',(3.24150677815,-35.2297273503,-3.67797056337));
#51836=CARTESIAN_POINT('Ctrl Pts',(3.25788366108,-35.2867834422,-3.68259788135));
#51837=CARTESIAN_POINT('Ctrl Pts',(3.2708619246,-35.3449131549,-3.6851550674));
#51838=CARTESIAN_POINT('Ctrl Pts',(3.28034612237,-35.4037663878,-3.68562224436));
#51839=CARTESIAN_POINT('Ctrl Pts',(3.28628025023,-35.4629813934,-3.68400243047));
#51840=CARTESIAN_POINT('Ctrl Pts',(3.28864951001,-35.5221963991,-3.68032135));
#51841=CARTESIAN_POINT('Ctrl Pts',(2.93020007641,-35.2159821642,-4.09471223066));
#51842=CARTESIAN_POINT('Ctrl Pts',(2.94976329618,-35.2791022779,-4.10741039029));
#51843=CARTESIAN_POINT('Ctrl Pts',(2.96507838407,-35.3440365738,-4.11671739461));
#51844=CARTESIAN_POINT('Ctrl Pts',(2.97596822887,-35.4101991223,-4.12255014873));
#51845=CARTESIAN_POINT('Ctrl Pts',(2.98233164479,-35.4769758456,-4.12487890497));
#51846=CARTESIAN_POINT('Ctrl Pts',(2.984147828,-35.543752569,-4.12372796686));
#51847=CARTESIAN_POINT('Ctrl Pts',(2.57349039398,-35.21650702,-4.45141980073));
#51848=CARTESIAN_POINT('Ctrl Pts',(2.58535390407,-35.2792535748,-4.47101557567));
#51849=CARTESIAN_POINT('Ctrl Pts',(2.59391358392,-35.3437511414,-4.48640413798));
#51850=CARTESIAN_POINT('Ctrl Pts',(2.59909669845,-35.4094332325,-4.49741590343));
#51851=CARTESIAN_POINT('Ctrl Pts',(2.60088024578,-35.4757076219,-4.50395318786));
#51852=CARTESIAN_POINT('Ctrl Pts',(2.59929137485,-35.5419820113,-4.50599426346));
#51853=CARTESIAN_POINT('Ctrl Pts',(2.15330460094,-35.2313461468,-4.76288665231));
#51854=CARTESIAN_POINT('Ctrl Pts',(2.15740174514,-35.2874140925,-4.77869293776));
#51855=CARTESIAN_POINT('Ctrl Pts',(2.15952364918,-35.3444755753,-4.7912469843));
#51856=CARTESIAN_POINT('Ctrl Pts',(2.15965446887,-35.4022061334,-4.8004623347));
#51857=CARTESIAN_POINT('Ctrl Pts',(2.15779886139,-35.4602712393,-4.80628788231));
#51858=CARTESIAN_POINT('Ctrl Pts',(2.15398176798,-35.5183363452,-4.80870937341));
#51859=CARTESIAN_POINT('Ctrl Pts',(1.69382497102,-35.2682575054,-5.0104353994));
#51860=CARTESIAN_POINT('Ctrl Pts',(1.69402180198,-35.3094041642,-5.02023545326));
#51861=CARTESIAN_POINT('Ctrl Pts',(1.69321049227,-35.3510179116,-5.02809462923));
#51862=CARTESIAN_POINT('Ctrl Pts',(1.69139030263,-35.3929453813,-5.0339763881));
#51863=CARTESIAN_POINT('Ctrl Pts',(1.68856804274,-35.4350297152,-5.03785872515));
#51864=CARTESIAN_POINT('Ctrl Pts',(1.68475791979,-35.477114049,-5.03973465917));
#51865=CARTESIAN_POINT('',(1.69382496789361,-35.2682576613344,-5.0104354398608));
#51866=CARTESIAN_POINT('Origin',(1.24303943910855,-35.4771140870975,-4.14258062935315));
#51867=CARTESIAN_POINT('',(3.48890306745266,-35.2652540841568,-3.21461371228527));
#51868=CARTESIAN_POINT('Ctrl Pts',(3.48890306460208,-35.2652540848695,-3.21461371081793));
#51869=CARTESIAN_POINT('Ctrl Pts',(3.44775130357986,-35.2593445965621,-3.29168823695534));
#51870=CARTESIAN_POINT('Ctrl Pts',(3.40380709382689,-35.2540719037323,-3.36847562230748));
#51871=CARTESIAN_POINT('Ctrl Pts',(3.35708951743242,-35.2494371435468,-3.44461007506016));
#51872=CARTESIAN_POINT('Ctrl Pts',(3.30985454838516,-35.2447510538393,-3.52158770953414));
#51873=CARTESIAN_POINT('Ctrl Pts',(3.2597844948942,-35.2407166455098,-3.59789767427568));
#51874=CARTESIAN_POINT('Ctrl Pts',(3.20687172401791,-35.2373316218687,-3.67320954173569));
#51875=CARTESIAN_POINT('Ctrl Pts',(3.15192353050766,-35.233816384791,-3.75141846934008));
#51876=CARTESIAN_POINT('Ctrl Pts',(3.09390910438811,-35.2310008789339,-3.82855109054718));
#51877=CARTESIAN_POINT('Ctrl Pts',(3.03279428228795,-35.2288868032877,-3.90429009496304));
#51878=CARTESIAN_POINT('Ctrl Pts',(2.96685035092806,-35.2266056797482,-3.98601376749996));
#51879=CARTESIAN_POINT('Ctrl Pts',(2.89729472225231,-35.2251402672288,-4.06611544111579));
#51880=CARTESIAN_POINT('Ctrl Pts',(2.82407449292744,-35.224509773473,-4.14425308595335));
#51881=CARTESIAN_POINT('Ctrl Pts',(2.79172464830231,-35.2242312114523,-4.17877552180443));
#51882=CARTESIAN_POINT('Ctrl Pts',(2.75865953861759,-35.224115929813,-4.21291522461585));
#51883=CARTESIAN_POINT('Ctrl Pts',(2.72487604324634,-35.2241673001316,-4.24664506250073));
#51884=CARTESIAN_POINT('Ctrl Pts',(2.65472562468747,-35.2242739690629,-4.31668406289263));
#51885=CARTESIAN_POINT('Ctrl Pts',(2.58276783092832,-35.2250970726848,-4.38366465920977));
#51886=CARTESIAN_POINT('Ctrl Pts',(2.50928836705134,-35.2266146759269,-4.44761232797486));
#51887=CARTESIAN_POINT('Ctrl Pts',(2.44121046007607,-35.2280207184712,-4.50685913267071));
#51888=CARTESIAN_POINT('Ctrl Pts',(2.37182601344067,-35.2300234573763,-4.56350349989407));
#51889=CARTESIAN_POINT('Ctrl Pts',(2.3014054178217,-35.2326174005493,-4.61756403780509));
#51890=CARTESIAN_POINT('Ctrl Pts',(2.23212377102363,-35.2351693905339,-4.67075022659467));
#51891=CARTESIAN_POINT('Ctrl Pts',(2.16183899809641,-35.2382939828071,-4.7214359382488));
#51892=CARTESIAN_POINT('Ctrl Pts',(2.09085658743666,-35.2419915887232,-4.76962725403854));
#51893=CARTESIAN_POINT('Ctrl Pts',(2.01848437800597,-35.2457615918445,-4.81876213078701));
#51894=CARTESIAN_POINT('Ctrl Pts',(1.94538686340585,-35.25012764269,-4.86530413139964));
#51895=CARTESIAN_POINT('Ctrl Pts',(1.87194092409075,-35.2550905119588,-4.90924276159168));
#51896=CARTESIAN_POINT('Ctrl Pts',(1.81272063931411,-35.2590921291231,-4.94467097201329));
#51897=CARTESIAN_POINT('Ctrl Pts',(1.75327501706489,-35.2634818477057,-4.97840619304004));
#51898=CARTESIAN_POINT('Ctrl Pts',(1.69382497176268,-35.2682576606557,-5.01043543637783));
#51899=CARTESIAN_POINT('Origin',(2.62096730277507,-35.4822399141373,-2.76784133732473));
#51900=CARTESIAN_POINT('Ctrl Pts',(1.65073607085,-35.2758272825,-5.03428274092));
#51901=CARTESIAN_POINT('Ctrl Pts',(1.65784980534,-35.3154856499,-5.03981034314));
#51902=CARTESIAN_POINT('Ctrl Pts',(1.66405083454,-35.3555597177,-5.04353006314));
#51903=CARTESIAN_POINT('Ctrl Pts',(1.66931464207,-35.3959128353,-5.04542284568));
#51904=CARTESIAN_POINT('Ctrl Pts',(1.67362302807,-35.4364054801,-5.0454821464));
#51905=CARTESIAN_POINT('Ctrl Pts',(1.67696448333,-35.4768981249,-5.04371406628));
#51906=CARTESIAN_POINT('Ctrl Pts',(1.61326364266,-35.2619218696,-5.05000316771));
#51907=CARTESIAN_POINT('Ctrl Pts',(1.62236549352,-35.3070877788,-5.05662956819));
#51908=CARTESIAN_POINT('Ctrl Pts',(1.63007921825,-35.3528484277,-5.0610482607));
#51909=CARTESIAN_POINT('Ctrl Pts',(1.63636464034,-35.3990097556,-5.06322951683));
#51910=CARTESIAN_POINT('Ctrl Pts',(1.64119504878,-35.4453707616,-5.06316361876));
#51911=CARTESIAN_POINT('Ctrl Pts',(1.64455688984,-35.4917317677,-5.06086202998));
#51912=CARTESIAN_POINT('Ctrl Pts',(1.57763814761,-35.2502524393,-5.07162003768));
#51913=CARTESIAN_POINT('Ctrl Pts',(1.58925529962,-35.3001212511,-5.07894359568));
#51914=CARTESIAN_POINT('Ctrl Pts',(1.59886212553,-35.350806501,-5.08374537669));
#51915=CARTESIAN_POINT('Ctrl Pts',(1.60640164997,-35.4020401921,-5.08598819927));
#51916=CARTESIAN_POINT('Ctrl Pts',(1.6118338475,-35.4535491166,-5.08566006898));
#51917=CARTESIAN_POINT('Ctrl Pts',(1.61513825447,-35.505058041,-5.08277314744));
#51918=CARTESIAN_POINT('Ctrl Pts',(1.5467652741,-35.2408307961,-5.09796224817));
#51919=CARTESIAN_POINT('Ctrl Pts',(1.56082810828,-35.2948250485,-5.10559533807));
#51920=CARTESIAN_POINT('Ctrl Pts',(1.5721279205,-35.3498911181,-5.11056679276));
#51921=CARTESIAN_POINT('Ctrl Pts',(1.58057518036,-35.4056813318,-5.11281573481));
#51922=CARTESIAN_POINT('Ctrl Pts',(1.58611547612,-35.4618331019,-5.11233170678));
#51923=CARTESIAN_POINT('Ctrl Pts',(1.58873141496,-35.5179848719,-5.10914094848));
#51924=CARTESIAN_POINT('Ctrl Pts',(1.50094788409,-35.2255784603,-5.15114151002));
#51925=CARTESIAN_POINT('Ctrl Pts',(1.51919307915,-35.2853745424,-5.15844241592));
#51926=CARTESIAN_POINT('Ctrl Pts',(1.53333303669,-35.34668297,-5.16330955045));
#51927=CARTESIAN_POINT('Ctrl Pts',(1.54322139667,-35.4090153954,-5.16568966994));
#51928=CARTESIAN_POINT('Ctrl Pts',(1.54877729981,-35.471860276,-5.16555970229));
#51929=CARTESIAN_POINT('Ctrl Pts',(1.54998925981,-35.5347051565,-5.16293840519));
#51930=CARTESIAN_POINT('Ctrl Pts',(1.47301395752,-35.2164048258,-5.21579034781));
#51931=CARTESIAN_POINT('Ctrl Pts',(1.49420720065,-35.2792319381,-5.22072059065));
#51932=CARTESIAN_POINT('Ctrl Pts',(1.51037196702,-35.3438574448,-5.22412710654));
#51933=CARTESIAN_POINT('Ctrl Pts',(1.52131309724,-35.4097044807,-5.22595779822));
#51934=CARTESIAN_POINT('Ctrl Pts',(1.52692924844,-35.4761620333,-5.22619785569));
#51935=CARTESIAN_POINT('Ctrl Pts',(1.52721834654,-35.5426195859,-5.22486268019));
#51936=CARTESIAN_POINT('Ctrl Pts',(1.46470315626,-35.213766631,-5.24531814123));
#51937=CARTESIAN_POINT('Ctrl Pts',(1.48680690707,-35.277355512,-5.24884399471));
#51938=CARTESIAN_POINT('Ctrl Pts',(1.50361778858,-35.3428209065,-5.25131648121));
#51939=CARTESIAN_POINT('Ctrl Pts',(1.51492750077,-35.4095603027,-5.25272449316));
#51940=CARTESIAN_POINT('Ctrl Pts',(1.52062825527,-35.4769374515,-5.25304460068));
#51941=CARTESIAN_POINT('Ctrl Pts',(1.52071813077,-35.5443146003,-5.25227472437));
#51942=CARTESIAN_POINT('Ctrl Pts',(1.46069629729,-35.2129478838,-5.27610920663));
#51943=CARTESIAN_POINT('Ctrl Pts',(1.48316494179,-35.2768382352,-5.27796326442));
#51944=CARTESIAN_POINT('Ctrl Pts',(1.50022470946,-35.3426337834,-5.2792979259));
#51945=CARTESIAN_POINT('Ctrl Pts',(1.51165995618,-35.4097245745,-5.28008044471));
#51946=CARTESIAN_POINT('Ctrl Pts',(1.51736021529,-35.4774626159,-5.28030986048));
#51947=CARTESIAN_POINT('Ctrl Pts',(1.51732687674,-35.5452006575,-5.27999548691));
#51948=CARTESIAN_POINT('Ctrl Pts',(1.46090316329,-35.2135376551,-5.30645216923));
#51949=CARTESIAN_POINT('Ctrl Pts',(1.48323786433,-35.277208474,-5.30683297122));
#51950=CARTESIAN_POINT('Ctrl Pts',(1.50020219619,-35.3427631323,-5.30721377032));
#51951=CARTESIAN_POINT('Ctrl Pts',(1.51158410625,-35.4095977304,-5.30759095434));
#51952=CARTESIAN_POINT('Ctrl Pts',(1.51727462121,-35.4770723771,-5.30796091202));
#51953=CARTESIAN_POINT('Ctrl Pts',(1.51727394979,-35.5445470238,-5.30832023528));
#51954=CARTESIAN_POINT('',(1.46090316329,-35.2135376551,-5.30645216923));
#51955=CARTESIAN_POINT('Origin',(0.517242653608352,-35.5445510518349,-5.30645466752134));
#51956=CARTESIAN_POINT('',(1.65073615060969,-35.2758275456144,-5.03428276116372));
#51957=CARTESIAN_POINT('Ctrl Pts',(1.65073607085,-35.2758272825,-5.03428274092));
#51958=CARTESIAN_POINT('Ctrl Pts',(1.63917641294469,-35.2715376801465,-5.03913224666584));
#51959=CARTESIAN_POINT('Ctrl Pts',(1.62778335848467,-35.2674875132726,-5.04467326186675));
#51960=CARTESIAN_POINT('Ctrl Pts',(1.61668444443609,-35.2636573158247,-5.05087657242354));
#51961=CARTESIAN_POINT('Ctrl Pts',(1.60383194679254,-35.2592219626488,-5.05805998099526));
#51962=CARTESIAN_POINT('Ctrl Pts',(1.59137279284757,-35.2550802614962,-5.06613093554639));
#51963=CARTESIAN_POINT('Ctrl Pts',(1.57945190627886,-35.2511801020351,-5.07508134045879));
#51964=CARTESIAN_POINT('Ctrl Pts',(1.57822278811962,-35.2507779711374,-5.07600418333185));
#51965=CARTESIAN_POINT('Ctrl Pts',(1.57699936255477,-35.2503784044852,-5.0769364083727));
#51966=CARTESIAN_POINT('Ctrl Pts',(1.5757817713614,-35.249981345754,-5.0778780290884));
#51967=CARTESIAN_POINT('Ctrl Pts',(1.56892018406347,-35.2477437694955,-5.08318441827502));
#51968=CARTESIAN_POINT('Ctrl Pts',(1.56238122240745,-35.2456299610748,-5.08867791263399));
#51969=CARTESIAN_POINT('Ctrl Pts',(1.55606420538616,-35.2435937838966,-5.09443615432473));
#51970=CARTESIAN_POINT('Ctrl Pts',(1.54987411671174,-35.2415985197954,-5.10007869518765));
#51971=CARTESIAN_POINT('Ctrl Pts',(1.54389660825347,-35.2396777876347,-5.10597582340282));
#51972=CARTESIAN_POINT('Ctrl Pts',(1.53806898844261,-35.2378043314629,-5.1122340347836));
#51973=CARTESIAN_POINT('Ctrl Pts',(1.53262204854038,-35.236053255808,-5.1180834385527));
#51974=CARTESIAN_POINT('Ctrl Pts',(1.52730576708068,-35.2343432891189,-5.12424859598885));
#51975=CARTESIAN_POINT('Ctrl Pts',(1.52210243099411,-35.2326677069358,-5.13084104408167));
#51976=CARTESIAN_POINT('Ctrl Pts',(1.51932482645314,-35.2317732606415,-5.13436017362742));
#51977=CARTESIAN_POINT('Ctrl Pts',(1.51658000405007,-35.2308888851264,-5.13800146111875));
#51978=CARTESIAN_POINT('Ctrl Pts',(1.51387019301489,-35.2300161278903,-5.14178470318121));
#51979=CARTESIAN_POINT('Ctrl Pts',(1.50899186094646,-35.2284449483662,-5.14859547737775));
#51980=CARTESIAN_POINT('Ctrl Pts',(1.50447971014778,-35.226974435639,-5.15550406977863));
#51981=CARTESIAN_POINT('Ctrl Pts',(1.50032158273591,-35.2256142603436,-5.16249261721141));
#51982=CARTESIAN_POINT('Ctrl Pts',(1.49062427650963,-35.2224421506284,-5.17879083942049));
#51983=CARTESIAN_POINT('Ctrl Pts',(1.48284972550606,-35.2198703197455,-5.19552723132818));
#51984=CARTESIAN_POINT('Ctrl Pts',(1.47685246235576,-35.2179251530912,-5.21241218505702));
#51985=CARTESIAN_POINT('Ctrl Pts',(1.47188719805485,-35.2163147074086,-5.22639160464748));
#51986=CARTESIAN_POINT('Ctrl Pts',(1.46814309341427,-35.2151376620024,-5.24047372826221));
#51987=CARTESIAN_POINT('Ctrl Pts',(1.46553748721243,-35.214392780468,-5.25447234610973));
#51988=CARTESIAN_POINT('Ctrl Pts',(1.46316296846251,-35.2137139614014,-5.26722944675239));
#51989=CARTESIAN_POINT('Ctrl Pts',(1.46173426076785,-35.2133943776133,-5.27991727358435));
#51990=CARTESIAN_POINT('Ctrl Pts',(1.461172945671,-35.2133981106173,-5.29237060577687));
#51991=CARTESIAN_POINT('Ctrl Pts',(1.46095968732751,-35.2133995288835,-5.29710195365816));
#51992=CARTESIAN_POINT('Ctrl Pts',(1.46087144111853,-35.2134472157513,-5.3017991828776));
#51993=CARTESIAN_POINT('Ctrl Pts',(1.46090316329,-35.2135376551,-5.30645216923));
#51994=CARTESIAN_POINT('Origin',(1.209267879813,-35.4768981557443,-4.15982468249633));
#51995=CARTESIAN_POINT('Ctrl Pts',(1.69382496103,-35.2682576589,-5.01043544546));
#51996=CARTESIAN_POINT('Ctrl Pts',(1.69402179658,-35.3094043143,-5.02023549828));
#51997=CARTESIAN_POINT('Ctrl Pts',(1.69321049045,-35.351018059,-5.02809467113));
#51998=CARTESIAN_POINT('Ctrl Pts',(1.69139030338,-35.3929455262,-5.03397642476));
#51999=CARTESIAN_POINT('Ctrl Pts',(1.68856804502,-35.4350298576,-5.03785875444));
#52000=CARTESIAN_POINT('Ctrl Pts',(1.6847579226,-35.4771141891,-5.03973467901));
#52001=CARTESIAN_POINT('Ctrl Pts',(1.68490151218,-35.268974041,-5.01524294734));
#52002=CARTESIAN_POINT('Ctrl Pts',(1.68651188124,-35.3098358784,-5.02415397172));
#52003=CARTESIAN_POINT('Ctrl Pts',(1.68714086448,-35.3511508863,-5.03116493545));
#52004=CARTESIAN_POINT('Ctrl Pts',(1.68678246934,-35.3927702163,-5.03624343644));
#52005=CARTESIAN_POINT('Ctrl Pts',(1.68543788474,-35.4345417096,-5.03937097175));
#52006=CARTESIAN_POINT('Ctrl Pts',(1.68311545107,-35.4763132029,-5.04054334111));
#52007=CARTESIAN_POINT('Ctrl Pts',(1.67612908012,-35.2701100859,-5.02003914153));
#52008=CARTESIAN_POINT('Ctrl Pts',(1.67913856906,-35.3106802184,-5.02807779826));
#52009=CARTESIAN_POINT('Ctrl Pts',(1.68118935788,-35.3516915586,-5.03424982493));
#52010=CARTESIAN_POINT('Ctrl Pts',(1.6822703811,-35.3929991785,-5.03852665843));
#52011=CARTESIAN_POINT('Ctrl Pts',(1.68237796302,-35.4344548915,-5.04089285688));
#52012=CARTESIAN_POINT('Ctrl Pts',(1.68151488066,-35.4759106045,-5.04134696784));
#52013=CARTESIAN_POINT('Ctrl Pts',(1.66745641736,-35.2716459733,-5.02484351574));
#52014=CARTESIAN_POINT('Ctrl Pts',(1.67185679176,-35.3119189644,-5.03202383893));
#52015=CARTESIAN_POINT('Ctrl Pts',(1.67531720482,-35.3526230495,-5.03736380107));
#52016=CARTESIAN_POINT('Ctrl Pts',(1.67782194293,-35.3936164734,-5.04083824001));
#52017=CARTESIAN_POINT('Ctrl Pts',(1.67936231019,-35.4347546994,-5.04243484007));
#52018=CARTESIAN_POINT('Ctrl Pts',(1.67993607839,-35.4758929253,-5.04215470289));
#52019=CARTESIAN_POINT('Ctrl Pts',(1.65900707813,-35.2735686701,-5.02958783575));
#52020=CARTESIAN_POINT('Ctrl Pts',(1.66477502429,-35.3135351172,-5.03593051298));
#52021=CARTESIAN_POINT('Ctrl Pts',(1.6696184323,-35.3539241381,-5.04045242297));
#52022=CARTESIAN_POINT('Ctrl Pts',(1.67351721006,-35.3945968399,-5.04313153636));
#52023=CARTESIAN_POINT('Ctrl Pts',(1.67645771737,-35.4354113842,-5.0439585342));
#52024=CARTESIAN_POINT('Ctrl Pts',(1.67843305643,-35.4762259285,-5.04293699751));
#52025=CARTESIAN_POINT('Ctrl Pts',(1.65073625045,-35.2758278019,-5.0342827697));
#52026=CARTESIAN_POINT('Ctrl Pts',(1.65785005217,-35.3154860139,-5.03981027692));
#52027=CARTESIAN_POINT('Ctrl Pts',(1.66405116082,-35.3555599215,-5.04352991245));
#52028=CARTESIAN_POINT('Ctrl Pts',(1.66931505993,-35.3959128757,-5.04542262153));
#52029=CARTESIAN_POINT('Ctrl Pts',(1.67362354949,-35.4364053554,-5.04548186008));
#52030=CARTESIAN_POINT('Ctrl Pts',(1.67696511998,-35.4768978351,-5.04371372921));
#52031=CARTESIAN_POINT('Ctrl Pts',(1.69382496014738,-35.268257661,-5.01043544642385));
#52032=CARTESIAN_POINT('Ctrl Pts',(1.68803312612198,-35.2687226336122,-5.01355579279809));
#52033=CARTESIAN_POINT('Ctrl Pts',(1.68231297816127,-35.2693997637279,-5.01667279399805));
#52034=CARTESIAN_POINT('Ctrl Pts',(1.67666523914987,-35.2702777195431,-5.0197822570377));
#52035=CARTESIAN_POINT('Ctrl Pts',(1.67037182346692,-35.2712560474872,-5.02324720883873));
#52036=CARTESIAN_POINT('Ctrl Pts',(1.66417391129964,-35.2724846442873,-5.02670011798684));
#52037=CARTESIAN_POINT('Ctrl Pts',(1.65809711371162,-35.2739404345783,-5.03012131671218));
#52038=CARTESIAN_POINT('Ctrl Pts',(1.65562402628534,-35.2745329006942,-5.03151364933934));
#52039=CARTESIAN_POINT('Ctrl Pts',(1.65317074085282,-35.2751628346991,-5.03290083178419));
#52040=CARTESIAN_POINT('Ctrl Pts',(1.65073625045,-35.2758278019,-5.0342827697));
#52041=CARTESIAN_POINT('Origin',(0.517276095271889,-35.5445396177181,-6.5565839998119));
#52042=CARTESIAN_POINT('',(1.46090089616294,-35.2135311920909,-7.94951678979554));
#52043=CARTESIAN_POINT('Origin',(0.51727190487542,-35.5445407938518,-7.94950134108497));
#52044=CARTESIAN_POINT('',(1.46090316329,-35.2135376551,-5.30645216923));
#52045=CARTESIAN_POINT('Ctrl Pts',(1.8311006173,-35.2589545751,-8.27964607156));
#52046=CARTESIAN_POINT('Ctrl Pts',(1.83516599722,-35.30564267,-8.26740892391));
#52047=CARTESIAN_POINT('Ctrl Pts',(1.83967892993,-35.3530290502,-8.25798461135));
#52048=CARTESIAN_POINT('Ctrl Pts',(1.84461954945,-35.4008855262,-8.25143297176));
#52049=CARTESIAN_POINT('Ctrl Pts',(1.84996359063,-35.4489770577,-8.24778618257));
#52050=CARTESIAN_POINT('Ctrl Pts',(1.85568309486,-35.4970685893,-8.24704782502));
#52051=CARTESIAN_POINT('Ctrl Pts',(1.8411549102,-35.2563947443,-8.27868180069));
#52052=CARTESIAN_POINT('Ctrl Pts',(1.84372513023,-35.3033039498,-8.26655797443));
#52053=CARTESIAN_POINT('Ctrl Pts',(1.84674896075,-35.3509164835,-8.25725221826));
#52054=CARTESIAN_POINT('Ctrl Pts',(1.85021379554,-35.3990025183,-8.25082395949));
#52055=CARTESIAN_POINT('Ctrl Pts',(1.85410255764,-35.447325312,-8.24730484866));
#52056=CARTESIAN_POINT('Ctrl Pts',(1.85839419939,-35.4956481058,-8.24669783586));
#52057=CARTESIAN_POINT('Ctrl Pts',(1.8515433823,-35.25441601,-8.27750101411));
#52058=CARTESIAN_POINT('Ctrl Pts',(1.85257607592,-35.3015060532,-8.26552228872));
#52059=CARTESIAN_POINT('Ctrl Pts',(1.85406935318,-35.3493041477,-8.25636790881));
#52060=CARTESIAN_POINT('Ctrl Pts',(1.85601808078,-35.3975789365,-8.25009675826));
#52061=CARTESIAN_POINT('Ctrl Pts',(1.8584126658,-35.4460920799,-8.24673979731));
#52062=CARTESIAN_POINT('Ctrl Pts',(1.86123915467,-35.4946052233,-8.24629917315));
#52063=CARTESIAN_POINT('Ctrl Pts',(1.86227923956,-35.2530824801,-8.2760758565));
#52064=CARTESIAN_POINT('Ctrl Pts',(1.86172760863,-35.3003142451,-8.26427721621));
#52065=CARTESIAN_POINT('Ctrl Pts',(1.86164442165,-35.3482586468,-8.25531090742));
#52066=CARTESIAN_POINT('Ctrl Pts',(1.86203232275,-35.3966828431,-8.24923515298));
#52067=CARTESIAN_POINT('Ctrl Pts',(1.86288941138,-35.4453469517,-8.24608002563));
#52068=CARTESIAN_POINT('Ctrl Pts',(1.86420909862,-35.4940110603,-8.24584666363));
#52069=CARTESIAN_POINT('Ctrl Pts',(1.8733302454,-35.2524719557,-8.27438297071));
#52070=CARTESIAN_POINT('Ctrl Pts',(1.87114978057,-35.2998071163,-8.26280107324));
#52071=CARTESIAN_POINT('Ctrl Pts',(1.86944655662,-35.34785966,-8.25406232754));
#52072=CARTESIAN_POINT('Ctrl Pts',(1.8682313281,-35.3963952193,-8.24822411924));
#52073=CARTESIAN_POINT('Ctrl Pts',(1.8675100956,-35.4451722935,-8.24531550566));
#52074=CARTESIAN_POINT('Ctrl Pts',(1.86728392959,-35.4939493677,-8.24533636007));
#52075=CARTESIAN_POINT('Ctrl Pts',(1.88461561635,-35.2526204897,-8.27242216736));
#52076=CARTESIAN_POINT('Ctrl Pts',(1.88077145213,-35.3000228694,-8.26109202298));
#52077=CARTESIAN_POINT('Ctrl Pts',(1.87741430691,-35.3481478104,-8.25261964893));
#52078=CARTESIAN_POINT('Ctrl Pts',(1.87456332753,-35.3967592797,-8.24706149184));
#52079=CARTESIAN_POINT('Ctrl Pts',(1.87223278053,-35.4456140212,-8.24444536521));
#52080=CARTESIAN_POINT('Ctrl Pts',(1.87043162953,-35.4944687629,-8.2447696254));
#52081=CARTESIAN_POINT('',(1.8846153427573,-35.2526204926719,-8.27242221793613));
#52082=CARTESIAN_POINT('Origin',(2.04762529146993,-35.4944692033061,-9.22894623475615));
#52083=CARTESIAN_POINT('',(1.83110037507866,-35.258953748698,-8.2796463148645));
#52084=CARTESIAN_POINT('Origin',(1.87243576229956,-35.4444265283287,-8.21862309905423));
#52085=CARTESIAN_POINT('Origin',(1.98368693863888,-35.4970721031414,-9.2388220939813));
#52086=CARTESIAN_POINT('Ctrl Pts',(1.46144763142,-35.2150898018,-7.98721591698));
#52087=CARTESIAN_POINT('Ctrl Pts',(1.48377600029,-35.278742568,-7.9813037531));
#52088=CARTESIAN_POINT('Ctrl Pts',(1.50069598676,-35.344292508,-7.97539158967));
#52089=CARTESIAN_POINT('Ctrl Pts',(1.51199409489,-35.4111316208,-7.96953590506));
#52090=CARTESIAN_POINT('Ctrl Pts',(1.51756138096,-35.4786154003,-7.96379316359));
#52091=CARTESIAN_POINT('Ctrl Pts',(1.51739959704,-35.5460991799,-7.95821663141));
#52092=CARTESIAN_POINT('Ctrl Pts',(1.45535023282,-35.1977075828,-8.04883580535));
#52093=CARTESIAN_POINT('Ctrl Pts',(1.48166949688,-35.2678829449,-8.03945279279));
#52094=CARTESIAN_POINT('Ctrl Pts',(1.50141667723,-35.3406016986,-8.03107453153));
#52095=CARTESIAN_POINT('Ctrl Pts',(1.51429114701,-35.4150544061,-8.02380364128));
#52096=CARTESIAN_POINT('Ctrl Pts',(1.52014358616,-35.4903742161,-8.01772327965));
#52097=CARTESIAN_POINT('Ctrl Pts',(1.51898580713,-35.5656940262,-8.01289172937));
#52098=CARTESIAN_POINT('Ctrl Pts',(1.46435245205,-35.1856198088,-8.11169781125));
#52099=CARTESIAN_POINT('Ctrl Pts',(1.49329848629,-35.2601192136,-8.09750578865));
#52100=CARTESIAN_POINT('Ctrl Pts',(1.51493019199,-35.3378102208,-8.08590190484));
#52101=CARTESIAN_POINT('Ctrl Pts',(1.52885470957,-35.4176855473,-8.07706315905));
#52102=CARTESIAN_POINT('Ctrl Pts',(1.53488112404,-35.4986532993,-8.07110658123));
#52103=CARTESIAN_POINT('Ctrl Pts',(1.53303520019,-35.5796210507,-8.06808053282));
#52104=CARTESIAN_POINT('Ctrl Pts',(1.49172176542,-35.1799552596,-8.17111299923));
#52105=CARTESIAN_POINT('Ctrl Pts',(1.51992397896,-35.2563325377,-8.15127801209));
#52106=CARTESIAN_POINT('Ctrl Pts',(1.54120100093,-35.3362785459,-8.13597848758));
#52107=CARTESIAN_POINT('Ctrl Pts',(1.5551380035,-35.4186751656,-8.12550808337));
#52108=CARTESIAN_POINT('Ctrl Pts',(1.56152781403,-35.5022972201,-8.12002297191));
#52109=CARTESIAN_POINT('Ctrl Pts',(1.5603885908,-35.5859192753,-8.11952822853));
#52110=CARTESIAN_POINT('Ctrl Pts',(1.57027832078,-35.1818573291,-8.25620202557));
#52111=CARTESIAN_POINT('Ctrl Pts',(1.59174100272,-35.2575761439,-8.2305972979));
#52112=CARTESIAN_POINT('Ctrl Pts',(1.60864769834,-35.3366611931,-8.21163579835));
#52113=CARTESIAN_POINT('Ctrl Pts',(1.62070812016,-35.4180526309,-8.19967893383));
#52114=CARTESIAN_POINT('Ctrl Pts',(1.62775389781,-35.5005977196,-8.19489712008));
#52115=CARTESIAN_POINT('Ctrl Pts',(1.62975211946,-35.5831428078,-8.19725603749));
#52116=CARTESIAN_POINT('Ctrl Pts',(1.67937525828,-35.2054111593,-8.29244102122));
#52117=CARTESIAN_POINT('Ctrl Pts',(1.69139601914,-35.2726177891,-8.26960761361));
#52118=CARTESIAN_POINT('Ctrl Pts',(1.70188615133,-35.3420423454,-8.25274940255));
#52119=CARTESIAN_POINT('Ctrl Pts',(1.7107273602,-35.4129758871,-8.24210785095));
#52120=CARTESIAN_POINT('Ctrl Pts',(1.71782785643,-35.4846639068,-8.23779633493));
#52121=CARTESIAN_POINT('Ctrl Pts',(1.72312748813,-35.5563519268,-8.23979333534));
#52122=CARTESIAN_POINT('Ctrl Pts',(1.73126212215,-35.2199435259,-8.29740056817));
#52123=CARTESIAN_POINT('Ctrl Pts',(1.73944999004,-35.2817848557,-8.27769690404));
#52124=CARTESIAN_POINT('Ctrl Pts',(1.74724337723,-35.3452273068,-8.26303381776));
#52125=CARTESIAN_POINT('Ctrl Pts',(1.75458028421,-35.4097526752,-8.25356881995));
#52126=CARTESIAN_POINT('Ctrl Pts',(1.76140026731,-35.4748200605,-8.24938018459));
#52127=CARTESIAN_POINT('Ctrl Pts',(1.7676477796,-35.5398874456,-8.25046377193));
#52128=CARTESIAN_POINT('Ctrl Pts',(1.78213085799,-35.2383375006,-8.29255588031));
#52129=CARTESIAN_POINT('Ctrl Pts',(1.7878752107,-35.2931533399,-8.27665796781));
#52130=CARTESIAN_POINT('Ctrl Pts',(1.79382722081,-35.3490506456,-8.26463904937));
#52131=CARTESIAN_POINT('Ctrl Pts',(1.79995135062,-35.4056781551,-8.25659979182));
#52132=CARTESIAN_POINT('Ctrl Pts',(1.80620870196,-35.4626704426,-8.2525916122));
#52133=CARTESIAN_POINT('Ctrl Pts',(1.81255794182,-35.5196627301,-8.25261467335));
#52134=CARTESIAN_POINT('Ctrl Pts',(1.83110005152,-35.2589529157,-8.27964657201));
#52135=CARTESIAN_POINT('Ctrl Pts',(1.83516520879,-35.3056415029,-8.26740924886));
#52136=CARTESIAN_POINT('Ctrl Pts',(1.83967790698,-35.3530283973,-8.25798482029));
#52137=CARTESIAN_POINT('Ctrl Pts',(1.84461828078,-35.4008854025,-8.25143312625));
#52138=CARTESIAN_POINT('Ctrl Pts',(1.84996206575,-35.4489774707,-8.24778634512));
#52139=CARTESIAN_POINT('Ctrl Pts',(1.85568130399,-35.4970695389,-8.24704805785));
#52140=CARTESIAN_POINT('',(1.46144760573678,-35.2150897285778,-7.98721594892785));
#52141=CARTESIAN_POINT('Ctrl Pts',(1.461447626411,-35.2150897875206,-7.98721596760062));
#52142=CARTESIAN_POINT('Ctrl Pts',(1.45975611672774,-35.2102676927798,-8.00431028529611));
#52143=CARTESIAN_POINT('Ctrl Pts',(1.45949088883459,-35.2060112736049,-8.0212499105763));
#52144=CARTESIAN_POINT('Ctrl Pts',(1.46063290708311,-35.2023078195083,-8.03785564020924));
#52145=CARTESIAN_POINT('Ctrl Pts',(1.4619849592698,-35.1979232457801,-8.0575154075472));
#52146=CARTESIAN_POINT('Ctrl Pts',(1.46530862871115,-35.1943131533458,-8.07670545288678));
#52147=CARTESIAN_POINT('Ctrl Pts',(1.47049421230562,-35.1914533514575,-8.09512876016919));
#52148=CARTESIAN_POINT('Ctrl Pts',(1.47590344828213,-35.1884702073275,-8.1143466581633));
#52149=CARTESIAN_POINT('Ctrl Pts',(1.48333705879276,-35.1863028020104,-8.13272925288172));
#52150=CARTESIAN_POINT('Ctrl Pts',(1.49261651363463,-35.1849311628113,-8.14996266488784));
#52151=CARTESIAN_POINT('Ctrl Pts',(1.50139934296483,-35.1836329321292,-8.16627376494771));
#52152=CARTESIAN_POINT('Ctrl Pts',(1.51183526909898,-35.1830473682593,-8.18155534070476));
#52153=CARTESIAN_POINT('Ctrl Pts',(1.52374090219576,-35.1831700187017,-8.19556753354493));
#52154=CARTESIAN_POINT('Ctrl Pts',(1.53476411711598,-35.183283578575,-8.20854117483937));
#52155=CARTESIAN_POINT('Ctrl Pts',(1.54704765661419,-35.1840042929883,-8.22042644252083));
#52156=CARTESIAN_POINT('Ctrl Pts',(1.56041708072795,-35.1853404899314,-8.23105732045887));
#52157=CARTESIAN_POINT('Ctrl Pts',(1.56910154768583,-35.1862084523884,-8.23796289151418));
#52158=CARTESIAN_POINT('Ctrl Pts',(1.57825731769038,-35.1873345507109,-8.24435196287183));
#52159=CARTESIAN_POINT('Ctrl Pts',(1.58782634821685,-35.1887261822664,-8.25017848425026));
#52160=CARTESIAN_POINT('Ctrl Pts',(1.60172467941707,-35.1907474273878,-8.25864108907095));
#52161=CARTESIAN_POINT('Ctrl Pts',(1.6164949308172,-35.1933280702808,-8.26591472259457));
#52162=CARTESIAN_POINT('Ctrl Pts',(1.63196242905032,-35.1964777725275,-8.27188457667519));
#52163=CARTESIAN_POINT('Ctrl Pts',(1.64849069024609,-35.1998434817482,-8.27826384409504));
#52164=CARTESIAN_POINT('Ctrl Pts',(1.66581448192413,-35.2038599872894,-8.28315426383548));
#52165=CARTESIAN_POINT('Ctrl Pts',(1.68369377872932,-35.208545021433,-8.28646866080559));
#52166=CARTESIAN_POINT('Ctrl Pts',(1.70103107100662,-35.2130880304318,-8.28968258300957));
#52167=CARTESIAN_POINT('Ctrl Pts',(1.71888903761226,-35.2182610669448,-8.29141505338385));
#52168=CARTESIAN_POINT('Ctrl Pts',(1.73704188098263,-35.2240674952026,-8.29163087046771));
#52169=CARTESIAN_POINT('Ctrl Pts',(1.75245675447925,-35.2289981474005,-8.2918141361401));
#52170=CARTESIAN_POINT('Ctrl Pts',(1.76808309114067,-35.2343860832447,-8.29090457051527));
#52171=CARTESIAN_POINT('Ctrl Pts',(1.78379592237618,-35.2402121797429,-8.28890352851202));
#52172=CARTESIAN_POINT('Ctrl Pts',(1.79823012727575,-35.2455641796059,-8.28706532062609));
#52173=CARTESIAN_POINT('Ctrl Pts',(1.81273625305411,-35.2512865057029,-8.28430641503284));
#52174=CARTESIAN_POINT('Ctrl Pts',(1.82724442381139,-35.2573372993209,-8.28064174154456));
#52175=CARTESIAN_POINT('Ctrl Pts',(1.82852960227087,-35.2578732972596,-8.28031711347759));
#52176=CARTESIAN_POINT('Ctrl Pts',(1.82981482215612,-35.2584118502895,-8.27998538547209));
#52177=CARTESIAN_POINT('Ctrl Pts',(1.83110005096932,-35.2589529154682,-8.27964657215517));
#52178=CARTESIAN_POINT('Origin',(0.51781791838867,-35.5460995682007,-7.98721608782858));
#52179=CARTESIAN_POINT('Ctrl Pts',(1.46090085849,-35.2135310847,-7.94951679032));
#52180=CARTESIAN_POINT('Ctrl Pts',(1.48323559961,-35.2772019758,-7.94951679554));
#52181=CARTESIAN_POINT('Ctrl Pts',(1.50020012625,-35.3427566518,-7.94951680076));
#52182=CARTESIAN_POINT('Ctrl Pts',(1.51158239151,-35.4095912303,-7.94951680594));
#52183=CARTESIAN_POINT('Ctrl Pts',(1.51727342189,-35.4770658384,-7.94951681101));
#52184=CARTESIAN_POINT('Ctrl Pts',(1.5172734197,-35.5445404466,-7.94951681593));
#52185=CARTESIAN_POINT('Ctrl Pts',(1.46090084734,-35.2135310529,-7.95714134841));
#52186=CARTESIAN_POINT('Ctrl Pts',(1.48323559207,-35.2772019436,-7.95594579353));
#52187=CARTESIAN_POINT('Ctrl Pts',(1.50020012179,-35.3427566195,-7.95475023866));
#52188=CARTESIAN_POINT('Ctrl Pts',(1.51158238894,-35.4095911981,-7.95356602458));
#52189=CARTESIAN_POINT('Ctrl Pts',(1.51727341997,-35.4770658064,-7.95240448782));
#52190=CARTESIAN_POINT('Ctrl Pts',(1.51727341782,-35.5445404148,-7.95127632944));
#52191=CARTESIAN_POINT('Ctrl Pts',(1.46095673562,-35.2136903768,-7.96472994159));
#52192=CARTESIAN_POINT('Ctrl Pts',(1.48329083274,-35.277359414,-7.96234446573));
#52193=CARTESIAN_POINT('Ctrl Pts',(1.50025081243,-35.3429136053,-7.95995898987));
#52194=CARTESIAN_POINT('Ctrl Pts',(1.51162447777,-35.4097486473,-7.95759614371));
#52195=CARTESIAN_POINT('Ctrl Pts',(1.51730285882,-35.477224193,-7.95527854376));
#52196=CARTESIAN_POINT('Ctrl Pts',(1.51728631578,-35.5446997387,-7.9530275433));
#52197=CARTESIAN_POINT('Ctrl Pts',(1.46106747229,-35.2140060602,-7.97227569366));
#52198=CARTESIAN_POINT('Ctrl Pts',(1.48340028139,-35.277671426,-7.9687069317));
#52199=CARTESIAN_POINT('Ctrl Pts',(1.50035124089,-35.3432246581,-7.96513816975));
#52200=CARTESIAN_POINT('Ctrl Pts',(1.51170786352,-35.4100606172,-7.96160330128));
#52201=CARTESIAN_POINT('Ctrl Pts',(1.51736118389,-35.4775380197,-7.95813620969));
#52202=CARTESIAN_POINT('Ctrl Pts',(1.51731187088,-35.5450154221,-7.95476887067));
#52203=CARTESIAN_POINT('Ctrl Pts',(1.4612316362,-35.2144740518,-7.97977268509));
#52204=CARTESIAN_POINT('Ctrl Pts',(1.48356253349,-35.2781339746,-7.97502812195));
#52205=CARTESIAN_POINT('Ctrl Pts',(1.50050012169,-35.3436857837,-7.9702835588));
#52206=CARTESIAN_POINT('Ctrl Pts',(1.51183147778,-35.4105231034,-7.96558416229));
#52207=CARTESIAN_POINT('Ctrl Pts',(1.51744764399,-35.4780032585,-7.96097508922));
#52208=CARTESIAN_POINT('Ctrl Pts',(1.51734975497,-35.5454834136,-7.95649894554));
#52209=CARTESIAN_POINT('Ctrl Pts',(1.461447583,-35.2150896638,-7.9872159128));
#52210=CARTESIAN_POINT('Ctrl Pts',(1.48377596485,-35.2787424258,-7.98130374694));
#52211=CARTESIAN_POINT('Ctrl Pts',(1.50069596198,-35.3442923623,-7.97539158107));
#52212=CARTESIAN_POINT('Ctrl Pts',(1.51199407822,-35.4111314721,-7.96953589364));
#52213=CARTESIAN_POINT('Ctrl Pts',(1.51756136975,-35.4786152489,-7.963793149));
#52214=CARTESIAN_POINT('Ctrl Pts',(1.5173995886,-35.5460990256,-7.95821661336));
#52215=CARTESIAN_POINT('Origin',(2.95627559618279,-39.4764825794548,-7.94254325147619));
#52216=CARTESIAN_POINT('Ctrl Pts',(2.02882252548,-35.2583787857,-8.24404394735));
#52217=CARTESIAN_POINT('Ctrl Pts',(2.02793435434,-35.304849438,-8.23266211897));
#52218=CARTESIAN_POINT('Ctrl Pts',(2.0275994353,-35.3519981482,-8.22400554803));
#52219=CARTESIAN_POINT('Ctrl Pts',(2.02782201048,-35.3996032301,-8.21812855721));
#52220=CARTESIAN_POINT('Ctrl Pts',(2.02860101303,-35.4474365049,-8.21505931587));
#52221=CARTESIAN_POINT('Ctrl Pts',(2.02993009745,-35.4952697797,-8.21479904026));
#52222=CARTESIAN_POINT('Ctrl Pts',(2.7603704221,-35.2788135941,-8.09044877058));
#52223=CARTESIAN_POINT('Ctrl Pts',(2.75916038902,-35.3170950643,-8.08332087145));
#52224=CARTESIAN_POINT('Ctrl Pts',(2.75848926909,-35.3556762451,-8.07788965412));
#52225=CARTESIAN_POINT('Ctrl Pts',(2.75836124945,-35.3944575182,-8.07416878882));
#52226=CARTESIAN_POINT('Ctrl Pts',(2.75877734505,-35.4333388354,-8.07216551353));
#52227=CARTESIAN_POINT('Ctrl Pts',(2.75973535856,-35.4722201525,-8.07188072536));
#52228=CARTESIAN_POINT('Ctrl Pts',(3.46770746463,-35.2977417588,-7.8780751558));
#52229=CARTESIAN_POINT('Ctrl Pts',(3.46660967304,-35.3282659767,-7.87385395784));
#52230=CARTESIAN_POINT('Ctrl Pts',(3.46593509074,-35.3589261674,-7.87061653092));
#52231=CARTESIAN_POINT('Ctrl Pts',(3.4656850911,-35.3896774143,-7.8683685806));
#52232=CARTESIAN_POINT('Ctrl Pts',(3.46586006339,-35.420474191,-7.86711317222));
#52233=CARTESIAN_POINT('Ctrl Pts',(3.46645942733,-35.4512709677,-7.86685062308));
#52234=CARTESIAN_POINT('Ctrl Pts',(4.1448564034,-35.31305193,-7.60417987874));
#52235=CARTESIAN_POINT('Ctrl Pts',(4.14387911843,-35.3375078051,-7.60136146782));
#52236=CARTESIAN_POINT('Ctrl Pts',(4.14322007764,-35.3620512903,-7.59920530757));
#52237=CARTESIAN_POINT('Ctrl Pts',(4.14288053918,-35.3866532884,-7.59771461525));
#52238=CARTESIAN_POINT('Ctrl Pts',(4.14286096901,-35.4112845426,-7.59689108063));
#52239=CARTESIAN_POINT('Ctrl Pts',(4.14316103429,-35.4359157968,-7.59673486922));
#52240=CARTESIAN_POINT('Ctrl Pts',(5.21843923371,-35.3262967395,-7.044990155));
#52241=CARTESIAN_POINT('Ctrl Pts',(5.21754878579,-35.3454147425,-7.04339100369));
#52242=CARTESIAN_POINT('Ctrl Pts',(5.21690210383,-35.3645740899,-7.04217483695));
#52243=CARTESIAN_POINT('Ctrl Pts',(5.21649981226,-35.3837610519,-7.04134271025));
#52244=CARTESIAN_POINT('Ctrl Pts',(5.21634220772,-35.4029618215,-7.04089517538));
#52245=CARTESIAN_POINT('Ctrl Pts',(5.21642926006,-35.422162591,-7.04083226933));
#52246=CARTESIAN_POINT('Ctrl Pts',(6.21090480851,-35.3291957718,-6.34191684905));
#52247=CARTESIAN_POINT('Ctrl Pts',(6.20990218356,-35.347292328,-6.34059495831));
#52248=CARTESIAN_POINT('Ctrl Pts',(6.20914711064,-35.3654273382,-6.33960321184));
#52249=CARTESIAN_POINT('Ctrl Pts',(6.20864031997,-35.3835880114,-6.33894257829));
#52250=CARTESIAN_POINT('Ctrl Pts',(6.20838217516,-35.401761516,-6.33861353938));
#52251=CARTESIAN_POINT('Ctrl Pts',(6.20837267016,-35.4199350207,-6.33861609384));
#52252=CARTESIAN_POINT('Ctrl Pts',(6.59524089295,-35.3292320711,-6.04038307893));
#52253=CARTESIAN_POINT('Ctrl Pts',(6.59420777333,-35.3473355691,-6.03905690773));
#52254=CARTESIAN_POINT('Ctrl Pts',(6.59343802139,-35.3654739877,-6.03805312954));
#52255=CARTESIAN_POINT('Ctrl Pts',(6.59293154067,-35.3836356047,-6.03737283826));
#52256=CARTESIAN_POINT('Ctrl Pts',(6.59268825297,-35.4018088233,-6.03701670404));
#52257=CARTESIAN_POINT('Ctrl Pts',(6.59270812441,-35.4199820418,-6.03698498184));
#52258=CARTESIAN_POINT('Ctrl Pts',(7.36674622516,-35.3292429118,-5.37908303219));
#52259=CARTESIAN_POINT('Ctrl Pts',(7.36563384979,-35.3471062503,-5.37795639383));
#52260=CARTESIAN_POINT('Ctrl Pts',(7.36479211144,-35.3650081661,-5.37711871787));
#52261=CARTESIAN_POINT('Ctrl Pts',(7.36422260417,-35.3829359555,-5.37657056503));
#52262=CARTESIAN_POINT('Ctrl Pts',(7.36392615799,-35.4008766793,-5.37631208835));
#52263=CARTESIAN_POINT('Ctrl Pts',(7.36390280813,-35.4188174032,-5.37634302053));
#52264=CARTESIAN_POINT('Ctrl Pts',(8.06644392307,-35.3242511579,-4.63577831824));
#52265=CARTESIAN_POINT('Ctrl Pts',(8.06481498329,-35.3443613723,-4.63450682037));
#52266=CARTESIAN_POINT('Ctrl Pts',(8.06356784153,-35.3645192368,-4.63357464248));
#52267=CARTESIAN_POINT('Ctrl Pts',(8.06270291188,-35.3847087915,-4.63298305339));
#52268=CARTESIAN_POINT('Ctrl Pts',(8.06222041463,-35.4049141939,-4.63273277941));
#52269=CARTESIAN_POINT('Ctrl Pts',(8.06212040397,-35.4251195963,-4.63282401372));
#52270=CARTESIAN_POINT('Ctrl Pts',(8.40676939645,-35.318254221,-4.22563363488));
#52271=CARTESIAN_POINT('Ctrl Pts',(8.40459143683,-35.3405015468,-4.22453866256));
#52272=CARTESIAN_POINT('Ctrl Pts',(8.40288571682,-35.3628356427,-4.22380563891));
#52273=CARTESIAN_POINT('Ctrl Pts',(8.40165936546,-35.3852283571,-4.22343491308));
#52274=CARTESIAN_POINT('Ctrl Pts',(8.40091620766,-35.4076503711,-4.22342586623));
#52275=CARTESIAN_POINT('Ctrl Pts',(8.40065659496,-35.4300723851,-4.22377686476));
#52276=CARTESIAN_POINT('Ctrl Pts',(8.6986202738,-35.3007569312,-3.78649453504));
#52277=CARTESIAN_POINT('Ctrl Pts',(8.69512018043,-35.3302263046,-3.78463499808));
#52278=CARTESIAN_POINT('Ctrl Pts',(8.69237513121,-35.3597713122,-3.78337739168));
#52279=CARTESIAN_POINT('Ctrl Pts',(8.69038139929,-35.3893659949,-3.78272454109));
#52280=CARTESIAN_POINT('Ctrl Pts',(8.68913711634,-35.4189855209,-3.78267851397));
#52281=CARTESIAN_POINT('Ctrl Pts',(8.68864247336,-35.4486050468,-3.78324063488));
#52282=CARTESIAN_POINT('Ctrl Pts',(8.93444618031,-35.2748044449,-3.31652377072));
#52283=CARTESIAN_POINT('Ctrl Pts',(8.92616350743,-35.3147858017,-3.31461838858));
#52284=CARTESIAN_POINT('Ctrl Pts',(8.91971795914,-35.3551905608,-3.31361146728));
#52285=CARTESIAN_POINT('Ctrl Pts',(8.91513837409,-35.3958795596,-3.31350964329));
#52286=CARTESIAN_POINT('Ctrl Pts',(8.91244074774,-35.4367106808,-3.31431327227));
#52287=CARTESIAN_POINT('Ctrl Pts',(8.91162790031,-35.4775418019,-3.31601642165));
#52288=CARTESIAN_POINT('',(8.93444610724292,-35.2748049035046,-3.31652381528626));
#52289=CARTESIAN_POINT('Origin',(9.81418541109622,-35.4775497621699,-3.74658646986247));
#52290=CARTESIAN_POINT('',(2.0288222656268,-35.2583777618445,-8.24404425484976));
#52291=CARTESIAN_POINT('Ctrl Pts',(2.02882252548,-35.2583787857,-8.24404394735));
#52292=CARTESIAN_POINT('Ctrl Pts',(2.18677753481697,-35.2627910468336,-8.21087984737389));
#52293=CARTESIAN_POINT('Ctrl Pts',(2.33861437522826,-35.2669852055805,-8.17542519196724));
#52294=CARTESIAN_POINT('Ctrl Pts',(2.48435108055497,-35.2709319401419,-8.13825000100819));
#52295=CARTESIAN_POINT('Ctrl Pts',(2.64525208832679,-35.2752893432196,-8.0972066298409));
#52296=CARTESIAN_POINT('Ctrl Pts',(2.79871785488418,-35.2793444717014,-8.05406686887132));
#52297=CARTESIAN_POINT('Ctrl Pts',(2.94483454315409,-35.2830773158073,-8.00961262753664));
#52298=CARTESIAN_POINT('Ctrl Pts',(3.03413015126555,-35.2853585513621,-7.98244551500408));
#52299=CARTESIAN_POINT('Ctrl Pts',(3.12068223968935,-35.2875198737809,-7.9547877183841));
#52300=CARTESIAN_POINT('Ctrl Pts',(3.20451874330892,-35.2895609699308,-7.9268175468804));
#52301=CARTESIAN_POINT('Ctrl Pts',(3.3572398925257,-35.2932791420423,-7.8758655563821));
#52302=CARTESIAN_POINT('Ctrl Pts',(3.50096252004891,-35.2965988835363,-7.82387548219649));
#52303=CARTESIAN_POINT('Ctrl Pts',(3.63595726353252,-35.2995836082428,-7.77186522336913));
#52304=CARTESIAN_POINT('Ctrl Pts',(3.65356195398893,-35.2999728467658,-7.76508255551418));
#52305=CARTESIAN_POINT('Ctrl Pts',(3.67101823732379,-35.3003564000405,-7.75829947690513));
#52306=CARTESIAN_POINT('Ctrl Pts',(3.68832673200562,-35.3007344202451,-7.75151817837785));
#52307=CARTESIAN_POINT('Ctrl Pts',(3.76334271985672,-35.3023727810382,-7.72212764977972));
#52308=CARTESIAN_POINT('Ctrl Pts',(3.83558426198059,-35.3038950886041,-7.69277255023342));
#52309=CARTESIAN_POINT('Ctrl Pts',(3.90510884594964,-35.3052987785019,-7.66362553964167));
#52310=CARTESIAN_POINT('Ctrl Pts',(3.93987113793416,-35.3060006234508,-7.64905203434579));
#52311=CARTESIAN_POINT('Ctrl Pts',(3.97395414544796,-35.3066728111262,-7.63453043970357));
#52312=CARTESIAN_POINT('Ctrl Pts',(4.00736544039963,-35.3073153616589,-7.62008124899256));
#52313=CARTESIAN_POINT('Ctrl Pts',(4.02407108787547,-35.3076366369253,-7.61285665363705));
#52314=CARTESIAN_POINT('Ctrl Pts',(4.04060880379702,-35.3079505016349,-7.60565015095042));
#52315=CARTESIAN_POINT('Ctrl Pts',(4.05697952642894,-35.3082569556414,-7.59846424465178));
#52316=CARTESIAN_POINT('Ctrl Pts',(4.06516488774489,-35.3084101826446,-7.59487129150247));
#52317=CARTESIAN_POINT('Ctrl Pts',(4.07330850050044,-35.3085615568926,-7.59128348690469));
#52318=CARTESIAN_POINT('Ctrl Pts',(4.08141048278529,-35.308711078371,-7.58770113942753));
#52319=CARTESIAN_POINT('Ctrl Pts',(4.08951246507013,-35.3088605998495,-7.58411879195037));
#52320=CARTESIAN_POINT('Ctrl Pts',(4.09652997069631,-35.3089893052348,-7.58100632499581));
#52321=CARTESIAN_POINT('Ctrl Pts',(4.10559165594891,-35.3091540843135,-7.5769707743543));
#52322=CARTESIAN_POINT('Ctrl Pts',(4.23911785829849,-35.311582145319,-7.517505924657));
#52323=CARTESIAN_POINT('Ctrl Pts',(4.37541831829351,-35.3138080692197,-7.45326567496979));
#52324=CARTESIAN_POINT('Ctrl Pts',(4.51410564517436,-35.3158091474134,-7.38380419075587));
#52325=CARTESIAN_POINT('Ctrl Pts',(4.63203743674429,-35.3175107501608,-7.32473810690604));
#52326=CARTESIAN_POINT('Ctrl Pts',(4.75169471236088,-35.319048903818,-7.26189640866632));
#52327=CARTESIAN_POINT('Ctrl Pts',(4.87285226581732,-35.3204169420525,-7.19504100971907));
#52328=CARTESIAN_POINT('Ctrl Pts',(4.91863422188269,-35.320933884369,-7.1697782766082));
#52329=CARTESIAN_POINT('Ctrl Pts',(4.96463057429613,-35.321426680412,-7.14394286693305));
#52330=CARTESIAN_POINT('Ctrl Pts',(5.01082994297537,-35.3218956802795,-7.11752369939173));
#52331=CARTESIAN_POINT('Ctrl Pts',(5.11691531470315,-35.3229726219502,-7.05685864509589));
#52332=CARTESIAN_POINT('Ctrl Pts',(5.22405614828952,-35.3239068291055,-6.99312243979726));
#52333=CARTESIAN_POINT('Ctrl Pts',(5.3321129332859,-35.3247083121071,-6.92621787562441));
#52334=CARTESIAN_POINT('Ctrl Pts',(5.35606344132569,-35.3248859587498,-6.91138865132189));
#52335=CARTESIAN_POINT('Ctrl Pts',(5.38005902814711,-35.3250571708672,-6.89640393554172));
#52336=CARTESIAN_POINT('Ctrl Pts',(5.40409832085966,-35.325222215338,-6.88126296256034));
#52337=CARTESIAN_POINT('Ctrl Pts',(5.43121311996124,-35.3254083750442,-6.864184904337));
#52338=CARTESIAN_POINT('Ctrl Pts',(5.45838352251183,-35.3255866912149,-6.84690805936453));
#52339=CARTESIAN_POINT('Ctrl Pts',(5.48560720457396,-35.3257572756508,-6.82943126754002));
#52340=CARTESIAN_POINT('Ctrl Pts',(5.56573339667789,-35.3262593488549,-6.77799264230574));
#52341=CARTESIAN_POINT('Ctrl Pts',(5.64632318459152,-35.3266943011098,-6.7248203623343));
#52342=CARTESIAN_POINT('Ctrl Pts',(5.72732506573132,-35.3270730527021,-6.66988195870045));
#52343=CARTESIAN_POINT('Ctrl Pts',(5.77469456688971,-35.327294544768,-6.63775425082558));
#52344=CARTESIAN_POINT('Ctrl Pts',(5.82179076014501,-35.3274946126195,-6.60530886215643));
#52345=CARTESIAN_POINT('Ctrl Pts',(5.86933240137305,-35.3276745273873,-6.5720410809232));
#52346=CARTESIAN_POINT('Ctrl Pts',(5.90308700092806,-35.3278022670022,-6.54842093225764));
#52347=CARTESIAN_POINT('Ctrl Pts',(5.93706562713996,-35.3279197935568,-6.52438529273794));
#52348=CARTESIAN_POINT('Ctrl Pts',(5.97151741326441,-35.3280268927031,-6.49973981824754));
#52349=CARTESIAN_POINT('Ctrl Pts',(6.07625212176294,-35.3283524780829,-6.42481666107839));
#52350=CARTESIAN_POINT('Ctrl Pts',(6.17799261229962,-35.3286064804706,-6.34951475089196));
#52351=CARTESIAN_POINT('Ctrl Pts',(6.27687958650818,-35.3288007027633,-6.27407844529289));
#52352=CARTESIAN_POINT('Ctrl Pts',(6.37620699077342,-35.3289957900975,-6.19830615594454));
#52353=CARTESIAN_POINT('Ctrl Pts',(6.47265578885625,-35.3291307886013,-6.12239783657176));
#52354=CARTESIAN_POINT('Ctrl Pts',(6.56633397049423,-35.3292071010504,-6.04656264049156));
#52355=CARTESIAN_POINT('Ctrl Pts',(6.66238066294141,-35.329285342944,-5.96881006644252));
#52356=CARTESIAN_POINT('Ctrl Pts',(6.75551494837276,-35.3293019838777,-5.89113406093224));
#52357=CARTESIAN_POINT('Ctrl Pts',(6.84581317853924,-35.3292450759539,-5.81372510819961));
#52358=CARTESIAN_POINT('Ctrl Pts',(6.85762114423611,-35.3292376343151,-5.8036026256569));
#52359=CARTESIAN_POINT('Ctrl Pts',(6.8693805591948,-35.3292289157708,-5.79348466563219));
#52360=CARTESIAN_POINT('Ctrl Pts',(6.88109154574958,-35.3292188763152,-5.78337161550293));
#52361=CARTESIAN_POINT('Ctrl Pts',(6.97439721443612,-35.3291388883386,-5.70279728469339));
#52362=CARTESIAN_POINT('Ctrl Pts',(7.06464238906416,-35.328985179861,-5.62252753578287));
#52363=CARTESIAN_POINT('Ctrl Pts',(7.15189748092528,-35.3287608286773,-5.54270464046465));
#52364=CARTESIAN_POINT('Ctrl Pts',(7.19349553981168,-35.3286538713233,-5.50464981261326));
#52365=CARTESIAN_POINT('Ctrl Pts',(7.23441338506565,-35.3285306520656,-5.46669605227421));
#52366=CARTESIAN_POINT('Ctrl Pts',(7.27465557605091,-35.3283904889136,-5.42885630951328));
#52367=CARTESIAN_POINT('Ctrl Pts',(7.29187189551032,-35.3283305246437,-5.41266779980036));
#52368=CARTESIAN_POINT('Ctrl Pts',(7.30896477210815,-35.3282674437883,-5.39649991143824));
#52369=CARTESIAN_POINT('Ctrl Pts',(7.32593406851701,-35.3282013929398,-5.38035392747592));
#52370=CARTESIAN_POINT('Ctrl Pts',(7.37039712118064,-35.3280283261088,-5.33804812304389));
#52371=CARTESIAN_POINT('Ctrl Pts',(7.41401265050169,-35.3278349578144,-5.29589242088803));
#52372=CARTESIAN_POINT('Ctrl Pts',(7.45679370714464,-35.3276206689168,-5.25389496570991));
#52373=CARTESIAN_POINT('Ctrl Pts',(7.48634791730271,-35.3274726328556,-5.22488208679023));
#52374=CARTESIAN_POINT('Ctrl Pts',(7.51550525137304,-35.3273147314449,-5.19594320056072));
#52375=CARTESIAN_POINT('Ctrl Pts',(7.54427073978588,-35.3271469506249,-5.16707824386914));
#52376=CARTESIAN_POINT('Ctrl Pts',(7.55865348399229,-35.3270630602149,-5.15264576552336));
#52377=CARTESIAN_POINT('Ctrl Pts',(7.57293825488062,-35.3269766983596,-5.1382317579152));
#52378=CARTESIAN_POINT('Ctrl Pts',(7.58712538578354,-35.3268878654927,-5.12383639135977));
#52379=CARTESIAN_POINT('Ctrl Pts',(7.59421895123501,-35.3268434490592,-5.11663870808206));
#52380=CARTESIAN_POINT('Ctrl Pts',(7.60128810618754,-35.3267984148055,-5.10944568456635));
#52381=CARTESIAN_POINT('Ctrl Pts',(7.60833288566123,-35.3267527624904,-5.10225734327071));
#52382=CARTESIAN_POINT('Ctrl Pts',(7.61185527539808,-35.3267299363328,-5.09866317262288));
#52383=CARTESIAN_POINT('Ctrl Pts',(7.61537157123757,-35.3267069556562,-5.09507017250368));
#52384=CARTESIAN_POINT('Ctrl Pts',(7.61888177667662,-35.3266838204384,-5.09147834630862));
#52385=CARTESIAN_POINT('Ctrl Pts',(7.62239198211567,-35.3266606852206,-5.08788652011355));
#52386=CARTESIAN_POINT('Ctrl Pts',(7.62478543468777,-35.3266448392919,-5.08543556574044));
#52387=CARTESIAN_POINT('Ctrl Pts',(7.62939412499817,-35.3266139511337,-5.08070639299966));
#52388=CARTESIAN_POINT('Ctrl Pts',(7.71724388637304,-35.3260251683897,-4.99056002411896));
#52389=CARTESIAN_POINT('Ctrl Pts',(7.80012523544823,-35.3252426647832,-4.90232735910713));
#52390=CARTESIAN_POINT('Ctrl Pts',(7.8781402873884,-35.3242422108242,-4.81627017606473));
#52391=CARTESIAN_POINT('Ctrl Pts',(7.93109327299415,-35.3235631492486,-4.7578585662332));
#52392=CARTESIAN_POINT('Ctrl Pts',(7.98180352905179,-35.3227842492524,-4.70045011363536));
#52393=CARTESIAN_POINT('Ctrl Pts',(8.0303108006439,-35.3219088916018,-4.64413249332142));
#52394=CARTESIAN_POINT('Ctrl Pts',(8.09029705160267,-35.3208263853717,-4.57448761751889));
#52395=CARTESIAN_POINT('Ctrl Pts',(8.14690751976985,-35.3195837043465,-4.50651864413491));
#52396=CARTESIAN_POINT('Ctrl Pts',(8.20023454467272,-35.3181885095926,-4.44041955605619));
#52397=CARTESIAN_POINT('Ctrl Pts',(8.22689805712416,-35.3174909122157,-4.40737001201683));
#52398=CARTESIAN_POINT('Ctrl Pts',(8.25274132262907,-35.3167554667997,-4.37478808215928));
#52399=CARTESIAN_POINT('Ctrl Pts',(8.27777958112633,-35.3159868446467,-4.34269824029458));
#52400=CARTESIAN_POINT('Ctrl Pts',(8.29029871037496,-35.3156025335702,-4.32665331936224));
#52401=CARTESIAN_POINT('Ctrl Pts',(8.30261653001456,-35.315210720873,-4.31073139713076));
#52402=CARTESIAN_POINT('Ctrl Pts',(8.31473547083024,-35.3148096730619,-4.29493563233504));
#52403=CARTESIAN_POINT('Ctrl Pts',(8.32079494123809,-35.3146091491563,-4.28703774993718));
#52404=CARTESIAN_POINT('Ctrl Pts',(8.32680469431384,-35.3144063137906,-4.2791714082933));
#52405=CARTESIAN_POINT('Ctrl Pts',(8.33276502615426,-35.3142011670248,-4.27133699140478));
#52406=CARTESIAN_POINT('Ctrl Pts',(8.33781611184359,-35.3140273153132,-4.26469771156446));
#52407=CARTESIAN_POINT('Ctrl Pts',(8.34198825082389,-35.3138816669016,-4.25919659070227));
#52408=CARTESIAN_POINT('Ctrl Pts',(8.34742624935289,-35.3136885395028,-4.25199874874118));
#52409=CARTESIAN_POINT('Ctrl Pts',(8.34840514370081,-35.3136537746315,-4.25070306490172));
#52410=CARTESIAN_POINT('Ctrl Pts',(8.34942495171374,-35.3136174507336,-4.24935232555719));
#52411=CARTESIAN_POINT('Ctrl Pts',(8.35049802910589,-35.3135790959847,-4.24792988360141));
#52412=CARTESIAN_POINT('Ctrl Pts',(8.41512795258716,-35.3112690440657,-4.16225822987801));
#52413=CARTESIAN_POINT('Ctrl Pts',(8.47750701667447,-35.30858490516,-4.07557038676447));
#52414=CARTESIAN_POINT('Ctrl Pts',(8.53739064535456,-35.3054895764863,-3.98787969849236));
#52415=CARTESIAN_POINT('Ctrl Pts',(8.5933670495396,-35.3025962085868,-3.9059105607134));
#52416=CARTESIAN_POINT('Ctrl Pts',(8.64716225878082,-35.2993434776791,-3.82306535457545));
#52417=CARTESIAN_POINT('Ctrl Pts',(8.69861273070644,-35.2957235257303,-3.73936182375594));
#52418=CARTESIAN_POINT('Ctrl Pts',(8.74688779638733,-35.2923269889922,-3.66082428470525));
#52419=CARTESIAN_POINT('Ctrl Pts',(8.7930983233281,-35.2886071906419,-3.58153121200422));
#52420=CARTESIAN_POINT('Ctrl Pts',(8.83714924844075,-35.2845783406043,-3.50150150967928));
#52421=CARTESIAN_POINT('Ctrl Pts',(8.87085295372428,-35.2814958361177,-3.44027016222879));
#52422=CARTESIAN_POINT('Ctrl Pts',(8.90329318573489,-35.2782328112362,-3.37860768781965));
#52423=CARTESIAN_POINT('Ctrl Pts',(8.93444613770044,-35.2748044495892,-3.31652385563538));
#52424=CARTESIAN_POINT('Origin',(2.2221106022258,-35.495269847715,-9.19615921132892));
#52425=CARTESIAN_POINT('Ctrl Pts',(8.93444595596,-35.2748053687,-3.31652394249));
#52426=CARTESIAN_POINT('Ctrl Pts',(8.92616317166,-35.3147866052,-3.31461891577));
#52427=CARTESIAN_POINT('Ctrl Pts',(8.91971750036,-35.3551912403,-3.31361234962));
#52428=CARTESIAN_POINT('Ctrl Pts',(8.91513778092,-35.3958801128,-3.31351087925));
#52429=CARTESIAN_POINT('Ctrl Pts',(8.91244000919,-35.4367111064,-3.31431485906));
#52430=CARTESIAN_POINT('Ctrl Pts',(8.91162700591,-35.4775421,-3.31601835533));
#52431=CARTESIAN_POINT('Ctrl Pts',(8.94734368663,-35.2728133782,-3.29109023634));
#52432=CARTESIAN_POINT('Ctrl Pts',(8.93895107582,-35.3135017401,-3.28875572575));
#52433=CARTESIAN_POINT('Ctrl Pts',(8.93246763725,-35.3546364096,-3.28733586636));
#52434=CARTESIAN_POINT('Ctrl Pts',(8.9279236303,-35.3960707679,-3.28683902656));
#52435=CARTESIAN_POINT('Ctrl Pts',(8.92533550226,-35.4376549725,-3.28726695529));
#52436=CARTESIAN_POINT('Ctrl Pts',(8.92470553582,-35.4792391771,-3.28861474271));
#52437=CARTESIAN_POINT('Ctrl Pts',(8.95983458954,-35.2711079221,-3.26569669172));
#52438=CARTESIAN_POINT('Ctrl Pts',(8.95141175919,-35.3123562177,-3.2628807422));
#52439=CARTESIAN_POINT('Ctrl Pts',(8.94495906105,-35.354070024,-3.26098724776));
#52440=CARTESIAN_POINT('Ctrl Pts',(8.94050773142,-35.3960964758,-3.260026589));
#52441=CARTESIAN_POINT('Ctrl Pts',(8.93807435022,-35.4382792543,-3.26000227455));
#52442=CARTESIAN_POINT('Ctrl Pts',(8.93766047318,-35.4804620328,-3.26091086944));
#52443=CARTESIAN_POINT('Ctrl Pts',(8.97214212604,-35.2697920542,-3.23978066277));
#52444=CARTESIAN_POINT('Ctrl Pts',(8.9637190734,-35.311417995,-3.23656869462));
#52445=CARTESIAN_POINT('Ctrl Pts',(8.95731138416,-35.3535230656,-3.23427864864));
#52446=CARTESIAN_POINT('Ctrl Pts',(8.95295080025,-35.3959499382,-3.2329226531));
#52447=CARTESIAN_POINT('Ctrl Pts',(8.95065387904,-35.4385377451,-3.23250578662));
#52448=CARTESIAN_POINT('Ctrl Pts',(8.95042158697,-35.481125552,-3.23302610121));
#52449=CARTESIAN_POINT('Ctrl Pts',(8.98911618271,-35.268630653,-3.20263013659));
#52450=CARTESIAN_POINT('Ctrl Pts',(8.98077765617,-35.3105436223,-3.19892614932));
#52451=CARTESIAN_POINT('Ctrl Pts',(8.97449392264,-35.3529460311,-3.19613159274));
#52452=CARTESIAN_POINT('Ctrl Pts',(8.97029699893,-35.3956772608,-3.19426066196));
#52453=CARTESIAN_POINT('Ctrl Pts',(8.96820302947,-35.4385728912,-3.19332056844));
#52454=CARTESIAN_POINT('Ctrl Pts',(8.96821193143,-35.4814685217,-3.19331131722));
#52455=CARTESIAN_POINT('Ctrl Pts',(9.00517206358,-35.2680735988,-3.16566118546));
#52456=CARTESIAN_POINT('Ctrl Pts',(8.99706509175,-35.3099657558,-3.16142494219));
#52457=CARTESIAN_POINT('Ctrl Pts',(8.99102314624,-35.3523468191,-3.15807110791));
#52458=CARTESIAN_POINT('Ctrl Pts',(8.98707727301,-35.395056319,-3.15561591639));
#52459=CARTESIAN_POINT('Ctrl Pts',(8.9852426452,-35.4379300459,-3.15406880151));
#52460=CARTESIAN_POINT('Ctrl Pts',(8.98551821082,-35.4808037728,-3.15343220651));
#52461=CARTESIAN_POINT('Ctrl Pts',(9.00990494748,-35.2680166859,-3.15455724964));
#52462=CARTESIAN_POINT('Ctrl Pts',(9.00187362208,-35.3098646744,-3.1501873274));
#52463=CARTESIAN_POINT('Ctrl Pts',(8.99590638677,-35.3522000159,-3.14669037035));
#52464=CARTESIAN_POINT('Ctrl Pts',(8.99203402793,-35.3948627823,-3.14408308561));
#52465=CARTESIAN_POINT('Ctrl Pts',(8.9902713955,-35.4376892422,-3.1423755103));
#52466=CARTESIAN_POINT('Ctrl Pts',(8.9906170886,-35.480515702,-3.141570683));
#52467=CARTESIAN_POINT('Ctrl Pts',(9.01453522232,-35.2679213672,-3.1435714055));
#52468=CARTESIAN_POINT('Ctrl Pts',(9.00660223792,-35.3097130029,-3.13902110731));
#52469=CARTESIAN_POINT('Ctrl Pts',(9.00073178209,-35.3519900952,-3.13533334259));
#52470=CARTESIAN_POINT('Ctrl Pts',(8.99695406159,-35.3945932824,-3.13252547117));
#52471=CARTESIAN_POINT('Ctrl Pts',(8.99528353801,-35.4373595352,-3.13060822223));
#52472=CARTESIAN_POINT('Ctrl Pts',(8.99571858313,-35.480125788,-3.12958551692));
#52473=CARTESIAN_POINT('Ctrl Pts',(9.01911869111,-35.2680072167,-3.13244884091));
#52474=CARTESIAN_POINT('Ctrl Pts',(9.01128168784,-35.3096922673,-3.12777947274));
#52475=CARTESIAN_POINT('Ctrl Pts',(9.00550009533,-35.3518590427,-3.12396085378));
#52476=CARTESIAN_POINT('Ctrl Pts',(9.00180365501,-35.3943494134,-3.12101070215));
#52477=CARTESIAN_POINT('Ctrl Pts',(9.00020644216,-35.4370015851,-3.1189402514));
#52478=CARTESIAN_POINT('Ctrl Pts',(9.0007065476,-35.4796537567,-3.11775399652));
#52479=CARTESIAN_POINT('',(9.01911881647387,-35.2680071588897,-3.13244858247421));
#52480=CARTESIAN_POINT('Origin',(9.92280365052534,-35.4797729820442,-3.5071455175773));
#52481=CARTESIAN_POINT('Ctrl Pts',(8.93444605244327,-35.2748053537986,-3.3165237522296));
#52482=CARTESIAN_POINT('Ctrl Pts',(8.93943079272288,-35.2740354916699,-3.30669407905226));
#52483=CARTESIAN_POINT('Ctrl Pts',(8.94434450694004,-35.2733170876845,-3.29686746416126));
#52484=CARTESIAN_POINT('Ctrl Pts',(8.94920327991744,-35.2726626041066,-3.28699933631088));
#52485=CARTESIAN_POINT('Ctrl Pts',(8.95476984379752,-35.2719127800951,-3.27569369097379));
#52486=CARTESIAN_POINT('Ctrl Pts',(8.96026395103588,-35.2712474673185,-3.26433388324753));
#52487=CARTESIAN_POINT('Ctrl Pts',(8.96568210534835,-35.2706788951834,-3.25291678406206));
#52488=CARTESIAN_POINT('Ctrl Pts',(8.97215885291872,-35.269999236026,-3.23926902411549));
#52489=CARTESIAN_POINT('Ctrl Pts',(8.97852555524635,-35.2694597083162,-3.22554138045548));
#52490=CARTESIAN_POINT('Ctrl Pts',(8.98475329027834,-35.2690516149317,-3.21179771950845));
#52491=CARTESIAN_POINT('Ctrl Pts',(8.98837850251731,-35.2688140606484,-3.20379742925564));
#52492=CARTESIAN_POINT('Ctrl Pts',(8.99195633450091,-35.2686203519649,-3.19579280171345));
#52493=CARTESIAN_POINT('Ctrl Pts',(8.99548251952631,-35.2684610265365,-3.18779854407026));
#52494=CARTESIAN_POINT('Ctrl Pts',(8.9985837231518,-35.2683209032609,-3.18076776701017));
#52495=CARTESIAN_POINT('Ctrl Pts',(9.00164600869916,-35.2682110262086,-3.17374049995815));
#52496=CARTESIAN_POINT('Ctrl Pts',(9.00466972421821,-35.2681329993825,-3.16671499647348));
#52497=CARTESIAN_POINT('Ctrl Pts',(9.00712768751884,-35.2680695717637,-3.16100399964687));
#52498=CARTESIAN_POINT('Ctrl Pts',(9.00955950605995,-35.2680241990286,-3.15529745602052));
#52499=CARTESIAN_POINT('Ctrl Pts',(9.0119661489852,-35.2679980780999,-3.14959278684721));
#52500=CARTESIAN_POINT('Ctrl Pts',(9.01413745424937,-35.2679745114506,-3.14444595842639));
#52501=CARTESIAN_POINT('Ctrl Pts',(9.0162880259156,-35.2679655281606,-3.13930185415533));
#52502=CARTESIAN_POINT('Ctrl Pts',(9.01842446912663,-35.267995823019,-3.13413122667487));
#52503=CARTESIAN_POINT('Ctrl Pts',(9.01865602825218,-35.2679991065376,-3.13357080645318));
#52504=CARTESIAN_POINT('Ctrl Pts',(9.01888742951289,-35.2680028851188,-3.13301003640059));
#52505=CARTESIAN_POINT('Ctrl Pts',(9.01911868766448,-35.2680072166355,-3.13244884927113));
#52506=CARTESIAN_POINT('Ctrl Pts',(9.01911953995,-35.2680044421,-3.13244837682));
#52507=CARTESIAN_POINT('Ctrl Pts',(9.01128290018,-35.3096899679,-3.12777753845));
#52508=CARTESIAN_POINT('Ctrl Pts',(9.00550173203,-35.3518572367,-3.12395745117));
#52509=CARTESIAN_POINT('Ctrl Pts',(9.00180577632,-35.3943481132,-3.12100583911));
#52510=CARTESIAN_POINT('Ctrl Pts',(9.00020910686,-35.4370007968,-3.11893394172));
#52511=CARTESIAN_POINT('Ctrl Pts',(9.00070981215,-35.4796534803,-3.1177462595));
#52512=CARTESIAN_POINT('Ctrl Pts',(9.17544595344,-35.2835018925,-2.74597776201));
#52513=CARTESIAN_POINT('Ctrl Pts',(9.16933554333,-35.3193494556,-2.74372235315));
#52514=CARTESIAN_POINT('Ctrl Pts',(9.16476148349,-35.3554672008,-2.74189804713));
#52515=CARTESIAN_POINT('Ctrl Pts',(9.1617381998,-35.3917657165,-2.74050818076));
#52516=CARTESIAN_POINT('Ctrl Pts',(9.1602730438,-35.428154617,-2.73955472374));
#52517=CARTESIAN_POINT('Ctrl Pts',(9.16036621938,-35.4645435174,-2.73903830807));
#52518=CARTESIAN_POINT('Ctrl Pts',(9.29269126807,-35.2907452551,-2.34477529883));
#52519=CARTESIAN_POINT('Ctrl Pts',(9.28707239127,-35.3238061129,-2.34352966982));
#52520=CARTESIAN_POINT('Ctrl Pts',(9.282834933,-35.3571174391,-2.34257541991));
#52521=CARTESIAN_POINT('Ctrl Pts',(9.27999356004,-35.3905967652,-2.34191674071));
#52522=CARTESIAN_POINT('Ctrl Pts',(9.27855558309,-35.424160093,-2.3415559411));
#52523=CARTESIAN_POINT('Ctrl Pts',(9.27852082014,-35.4577234207,-2.34149337034));
#52524=CARTESIAN_POINT('Ctrl Pts',(9.36191429928,-35.2893802972,-1.92981468559));
#52525=CARTESIAN_POINT('Ctrl Pts',(9.3560452611,-35.3232454878,-1.92921642136));
#52526=CARTESIAN_POINT('Ctrl Pts',(9.35161541947,-35.3573586818,-1.92882344418));
#52527=CARTESIAN_POINT('Ctrl Pts',(9.34863880943,-35.3916379824,-1.92863719423));
#52528=CARTESIAN_POINT('Ctrl Pts',(9.3471225791,-35.4260003368,-1.92865812789));
#52529=CARTESIAN_POINT('Ctrl Pts',(9.3470668903,-35.4603626911,-1.92888572013));
#52530=CARTESIAN_POINT('Ctrl Pts',(9.4171903904,-35.2789856765,-1.18748239275));
#52531=CARTESIAN_POINT('Ctrl Pts',(9.40981639515,-35.3169659165,-1.18801696878));
#52532=CARTESIAN_POINT('Ctrl Pts',(9.40425718706,-35.3552891517,-1.18859518921));
#52533=CARTESIAN_POINT('Ctrl Pts',(9.40053397643,-35.3938423214,-1.18921641071));
#52534=CARTESIAN_POINT('Ctrl Pts',(9.39865750897,-35.4325104595,-1.18987939995));
#52535=CARTESIAN_POINT('Ctrl Pts',(9.39862789646,-35.4711785976,-1.19058233503));
#52536=CARTESIAN_POINT('Ctrl Pts',(9.38314539193,-35.2631816303,-0.439456405049));
#52537=CARTESIAN_POINT('Ctrl Pts',(9.37293597078,-35.3077684071,-0.441248963721));
#52538=CARTESIAN_POINT('Ctrl Pts',(9.36525594777,-35.3529358557,-0.442871125473));
#52539=CARTESIAN_POINT('Ctrl Pts',(9.36014835673,-35.3984936385,-0.444315444411));
#52540=CARTESIAN_POINT('Ctrl Pts',(9.35763482817,-35.4442465927,-0.44557584201));
#52541=CARTESIAN_POINT('Ctrl Pts',(9.3577150604,-35.489999547,-0.446647757649));
#52542=CARTESIAN_POINT('Ctrl Pts',(9.3558891039,-35.2557890156,-0.116721794816));
#52543=CARTESIAN_POINT('Ctrl Pts',(9.34426128655,-35.3033050214,-0.118995176137));
#52544=CARTESIAN_POINT('Ctrl Pts',(9.33551278911,-35.3515333802,-0.120988679218));
#52545=CARTESIAN_POINT('Ctrl Pts',(9.3296998933,-35.4002411909,-0.122691582222));
#52546=CARTESIAN_POINT('Ctrl Pts',(9.32685085926,-35.4491887348,-0.124095735733));
#52547=CARTESIAN_POINT('Ctrl Pts',(9.32696513263,-35.4981362787,-0.12519578818));
#52548=CARTESIAN_POINT('Ctrl Pts',(9.3192256268,-35.2483585547,0.204089324846));
#52549=CARTESIAN_POINT('Ctrl Pts',(9.30607279618,-35.2988047548,0.201137625763));
#52550=CARTESIAN_POINT('Ctrl Pts',(9.29617649939,-35.3501183672,0.198586534665));
#52551=CARTESIAN_POINT('Ctrl Pts',(9.28960975953,-35.4020166188,0.196452114669));
#52552=CARTESIAN_POINT('Ctrl Pts',(9.28640921473,-35.4542072015,0.194746107875));
#52553=CARTESIAN_POINT('Ctrl Pts',(9.28657394094,-35.5063977842,0.193475565417));
#52554=CARTESIAN_POINT('Ctrl Pts',(9.27386188307,-35.2408046524,0.522899877563));
#52555=CARTESIAN_POINT('Ctrl Pts',(9.25898070398,-35.2942887044,0.519158422332));
#52556=CARTESIAN_POINT('Ctrl Pts',(9.24778010992,-35.3488352241,0.515965853737));
#52557=CARTESIAN_POINT('Ctrl Pts',(9.24035614705,-35.4040992505,0.513346313675));
#52558=CARTESIAN_POINT('Ctrl Pts',(9.2367570062,-35.4597220507,0.511316806249));
#52559=CARTESIAN_POINT('Ctrl Pts',(9.23698117834,-35.5153448509,0.509886546917));
#52560=CARTESIAN_POINT('',(9.27386188271851,-35.2408046524422,0.522899877211493));
#52561=CARTESIAN_POINT('Origin',(10.2249210130936,-35.5153449925992,0.664731557103899));
#52562=CARTESIAN_POINT('Ctrl Pts',(9.01911901239593,-35.2680072483449,-3.13244806238356));
#52563=CARTESIAN_POINT('Ctrl Pts',(9.04723758683849,-35.2707933216705,-3.06293411125694));
#52564=CARTESIAN_POINT('Ctrl Pts',(9.07420491323081,-35.2732952866302,-2.99193253005062));
#52565=CARTESIAN_POINT('Ctrl Pts',(9.09979229073556,-35.2754876019786,-2.91946334446916));
#52566=CARTESIAN_POINT('Ctrl Pts',(9.12398764134561,-35.2775606490697,-2.85093669091733));
#52567=CARTESIAN_POINT('Ctrl Pts',(9.1469491132796,-35.2793568774923,-2.78109788353282));
#52568=CARTESIAN_POINT('Ctrl Pts',(9.16852081216598,-35.2808658327816,-2.7099817552574));
#52569=CARTESIAN_POINT('Ctrl Pts',(9.19071305145076,-35.2824181953018,-2.63681987106791));
#52570=CARTESIAN_POINT('Ctrl Pts',(9.21143546536842,-35.2836665588565,-2.56230237824364));
#52571=CARTESIAN_POINT('Ctrl Pts',(9.2305669901781,-35.2846122497235,-2.48646441291759));
#52572=CARTESIAN_POINT('Ctrl Pts',(9.24491563378535,-35.2853215178737,-2.42958593892305));
#52573=CARTESIAN_POINT('Ctrl Pts',(9.25837039520488,-35.285860794621,-2.37196477580435));
#52574=CARTESIAN_POINT('Ctrl Pts',(9.27089709582343,-35.2862350344547,-2.31361779737502));
#52575=CARTESIAN_POINT('Ctrl Pts',(9.27207147400642,-35.2862701194391,-2.30814776814727));
#52576=CARTESIAN_POINT('Ctrl Pts',(9.27323770564116,-35.2863037565467,-2.30267136109724));
#52577=CARTESIAN_POINT('Ctrl Pts',(9.27439576888682,-35.2863359514877,-2.29718859098508));
#52578=CARTESIAN_POINT('Ctrl Pts',(9.27495670577144,-35.2863515459122,-2.294532874212));
#52579=CARTESIAN_POINT('Ctrl Pts',(9.27551572621074,-35.286366801981,-2.29187566454904));
#52580=CARTESIAN_POINT('Ctrl Pts',(9.2760728278078,-35.2863817203657,-2.28921696370895));
#52581=CARTESIAN_POINT('Ctrl Pts',(9.27630406080572,-35.286387912455,-2.28811343184139));
#52582=CARTESIAN_POINT('Ctrl Pts',(9.27653496322923,-35.2863940463689,-2.28700964307651));
#52583=CARTESIAN_POINT('Ctrl Pts',(9.27676553490977,-35.286400122156,-2.28590559753794));
#52584=CARTESIAN_POINT('Ctrl Pts',(9.27697890363755,-35.2864057446287,-2.28488392483543));
#52585=CARTESIAN_POINT('Ctrl Pts',(9.27719124975535,-35.2864112984818,-2.28386559649145));
#52586=CARTESIAN_POINT('Ctrl Pts',(9.27740737627875,-35.2864169073712,-2.28282750369869));
#52587=CARTESIAN_POINT('Ctrl Pts',(9.27850111635318,-35.2864452919815,-2.27757408236655));
#52588=CARTESIAN_POINT('Ctrl Pts',(9.27966393451027,-35.2864742483586,-2.27194332303056));
#52589=CARTESIAN_POINT('Ctrl Pts',(9.28075079770566,-35.2865001446825,-2.26663647342955));
#52590=CARTESIAN_POINT('Ctrl Pts',(9.28127724706593,-35.2865126882144,-2.26406596815406));
#52591=CARTESIAN_POINT('Ctrl Pts',(9.2817860161204,-35.2865245364181,-2.26157149447093));
#52592=CARTESIAN_POINT('Ctrl Pts',(9.28226134927632,-35.2865353930508,-2.25923293064942));
#52593=CARTESIAN_POINT('Ctrl Pts',(9.28253429611568,-35.28654162717,-2.25789007544194));
#52594=CARTESIAN_POINT('Ctrl Pts',(9.28279622640398,-35.2865475356617,-2.25659863067582));
#52595=CARTESIAN_POINT('Ctrl Pts',(9.28304421219757,-35.2865530711993,-2.25537373436067));
#52596=CARTESIAN_POINT('Ctrl Pts',(9.28313947183165,-35.2865551975844,-2.25490321073473));
#52597=CARTESIAN_POINT('Ctrl Pts',(9.28323306243032,-35.2865572778078,-2.25444059493792));
#52598=CARTESIAN_POINT('Ctrl Pts',(9.28332724213507,-35.2865593623391,-2.25397473534079));
#52599=CARTESIAN_POINT('Ctrl Pts',(9.29788837172528,-35.2868816518457,-2.18194815613067));
#52600=CARTESIAN_POINT('Ctrl Pts',(9.31146872667869,-35.2869688785728,-2.10674755967947));
#52601=CARTESIAN_POINT('Ctrl Pts',(9.32376997890423,-35.2868002832768,-2.02836049238632));
#52602=CARTESIAN_POINT('Ctrl Pts',(9.33390631642818,-35.2866613593043,-1.9637688754494));
#52603=CARTESIAN_POINT('Ctrl Pts',(9.34317423335416,-35.2863489237478,-1.89701404272316));
#52604=CARTESIAN_POINT('Ctrl Pts',(9.35142640756365,-35.2858605440817,-1.82810511544412));
#52605=CARTESIAN_POINT('Ctrl Pts',(9.36058428003333,-35.2853185634369,-1.75163324851255));
#52606=CARTESIAN_POINT('Ctrl Pts',(9.36849034355677,-35.2845592448402,-1.67250678259968));
#52607=CARTESIAN_POINT('Ctrl Pts',(9.37497292578257,-35.283623339191,-1.59076151627657));
#52608=CARTESIAN_POINT('Ctrl Pts',(9.37821421689547,-35.2831553863665,-1.54988888311502));
#52609=CARTESIAN_POINT('Ctrl Pts',(9.38110084025768,-35.282640335853,-1.50836204477103));
#52610=CARTESIAN_POINT('Ctrl Pts',(9.38361747795923,-35.2820739559404,-1.4661885577414));
#52611=CARTESIAN_POINT('Ctrl Pts',(9.38487579681,-35.2817907659841,-1.44510181422658));
#52612=CARTESIAN_POINT('Ctrl Pts',(9.38604167032792,-35.2814947469656,-1.42385340943051));
#52613=CARTESIAN_POINT('Ctrl Pts',(9.38711338690994,-35.2811858908628,-1.40244454238854));
#52614=CARTESIAN_POINT('Ctrl Pts',(9.38764924520095,-35.2810314628114,-1.39174010886756));
#52615=CARTESIAN_POINT('Ctrl Pts',(9.38816156747465,-35.2808738260956,-1.38099555997792));
#52616=CARTESIAN_POINT('Ctrl Pts',(9.38865015904411,-35.2807129817596,-1.37021105531062));
#52617=CARTESIAN_POINT('Ctrl Pts',(9.38889445482884,-35.2806325595916,-1.36481880297698));
#52618=CARTESIAN_POINT('Ctrl Pts',(9.38913281813932,-35.2805513355577,-1.35941656170578));
#52619=CARTESIAN_POINT('Ctrl Pts',(9.38936522585477,-35.2804693098204,-1.35400435240585));
#52620=CARTESIAN_POINT('Ctrl Pts',(9.38948142971249,-35.2804282969518,-1.35129824775589));
#52621=CARTESIAN_POINT('Ctrl Pts',(9.38959614468414,-35.2803870836597,-1.34858965109911));
#52622=CARTESIAN_POINT('Ctrl Pts',(9.38970936795586,-35.2803456699662,-1.34587856511458));
#52623=CARTESIAN_POINT('Ctrl Pts',(9.38982259122758,-35.2803042562727,-1.34316747913004));
#52624=CARTESIAN_POINT('Ctrl Pts',(9.38998713981212,-35.280242607951,-1.33915257906503));
#52625=CARTESIAN_POINT('Ctrl Pts',(9.39004455990828,-35.2802208277092,-1.33773784187776));
#52626=CARTESIAN_POINT('Ctrl Pts',(9.39247225065664,-35.2792999708152,-1.27792351535704));
#52627=CARTESIAN_POINT('Ctrl Pts',(9.39441622714332,-35.2781841374586,-1.21105163812287));
#52628=CARTESIAN_POINT('Ctrl Pts',(9.39537367391675,-35.2768634271352,-1.13709139363227));
#52629=CARTESIAN_POINT('Ctrl Pts',(9.39559420549972,-35.2765592239707,-1.12005590900016));
#52630=CARTESIAN_POINT('Ctrl Pts',(9.39576230582339,-35.2762442449781,-1.10264453707456));
#52631=CARTESIAN_POINT('Ctrl Pts',(9.39587173465696,-35.2759185569207,-1.08485724332022));
#52632=CARTESIAN_POINT('Ctrl Pts',(9.39630799718663,-35.2746201286072,-1.0139442168714));
#52633=CARTESIAN_POINT('Ctrl Pts',(9.39581034995002,-35.2731508427485,-0.937053566237884));
#52634=CARTESIAN_POINT('Ctrl Pts',(9.39399461730175,-35.2715038208048,-0.85419236772634));
#52635=CARTESIAN_POINT('Ctrl Pts',(9.39225680407881,-35.2699274783212,-0.774887032450933));
#52636=CARTESIAN_POINT('Ctrl Pts',(9.38931064280304,-35.2681881426592,-0.690112287146941));
#52637=CARTESIAN_POINT('Ctrl Pts',(9.38484507129186,-35.2662900810482,-0.599909998384288));
#52638=CARTESIAN_POINT('Ctrl Pts',(9.38024844937121,-35.2643363173282,-0.50706055754988));
#52639=CARTESIAN_POINT('Ctrl Pts',(9.37404580640433,-35.2622003616864,-0.408474248060987));
#52640=CARTESIAN_POINT('Ctrl Pts',(9.36593741539263,-35.2598862246104,-0.304192156387564));
#52641=CARTESIAN_POINT('Ctrl Pts',(9.3564241061767,-35.2571711234836,-0.181841398716708));
#52642=CARTESIAN_POINT('Ctrl Pts',(9.34428932059871,-35.2542113363005,-0.0516501610174696));
#52643=CARTESIAN_POINT('Ctrl Pts',(9.32909395555769,-35.2510260462912,0.0862479119727824));
#52644=CARTESIAN_POINT('Ctrl Pts',(9.31796381762815,-35.2486929192453,0.187254012744678));
#52645=CARTESIAN_POINT('Ctrl Pts',(9.3051945285179,-35.2462396541912,0.292392266742369));
#52646=CARTESIAN_POINT('Ctrl Pts',(9.29059844484657,-35.2436690517339,0.401604163680389));
#52647=CARTESIAN_POINT('Ctrl Pts',(9.28526729841894,-35.2427301520663,0.441493261833483));
#52648=CARTESIAN_POINT('Ctrl Pts',(9.2796920959383,-35.2417754911663,0.481925890883731));
#52649=CARTESIAN_POINT('Ctrl Pts',(9.27386188313803,-35.2408046525553,0.522899876806236));
#52650=CARTESIAN_POINT('Ctrl Pts',(1.88364028582742,-35.2522336654635,-8.27268614758859));
#52651=CARTESIAN_POINT('Ctrl Pts',(1.87976663689926,-35.2997052295165,-8.26132512102646));
#52652=CARTESIAN_POINT('Ctrl Pts',(1.87638081507785,-35.3479026421397,-8.25283069221518));
#52653=CARTESIAN_POINT('Ctrl Pts',(1.87350217466588,-35.3965887842191,-8.24725963970389));
#52654=CARTESIAN_POINT('Ctrl Pts',(1.87114516584333,-35.4455192584089,-8.24463992898022));
#52655=CARTESIAN_POINT('Ctrl Pts',(1.86931890580546,-35.4944496516172,-8.24496988273828));
#52656=CARTESIAN_POINT('Ctrl Pts',(1.91281732676632,-35.2526046602642,-8.26762695724934));
#52657=CARTESIAN_POINT('Ctrl Pts',(1.90952279963636,-35.3002628262793,-8.25608047625197));
#52658=CARTESIAN_POINT('Ctrl Pts',(1.90673790621558,-35.348655083091,-8.24741759078021));
#52659=CARTESIAN_POINT('Ctrl Pts',(1.90447924341404,-35.3975416565539,-8.24169641976602));
#52660=CARTESIAN_POINT('Ctrl Pts',(1.90275826638143,-35.4466753525817,-8.23894588545803));
#52661=CARTESIAN_POINT('Ctrl Pts',(1.90158091110236,-35.4958089664898,-8.23916485303755));
#52662=CARTESIAN_POINT('Ctrl Pts',(1.94211315375089,-35.2533826883717,-8.26220387826513));
#52663=CARTESIAN_POINT('Ctrl Pts',(1.93941688088205,-35.3010369730568,-8.25055875462903));
#52664=CARTESIAN_POINT('Ctrl Pts',(1.9372487324096,-35.3494248319395,-8.24179185740762));
#52665=CARTESIAN_POINT('Ctrl Pts',(1.93562271894448,-35.3983065050355,-8.23596172652887));
#52666=CARTESIAN_POINT('Ctrl Pts',(1.9345461395142,-35.4474352783484,-8.23309792984346));
#52667=CARTESIAN_POINT('Ctrl Pts',(1.93402206538774,-35.4965639696529,-8.23319987074611));
#52668=CARTESIAN_POINT('Ctrl Pts',(1.97257776832187,-35.2536956114026,-8.25641928888991));
#52669=CARTESIAN_POINT('Ctrl Pts',(1.96997955469349,-35.3013407205115,-8.24478001979218));
#52670=CARTESIAN_POINT('Ctrl Pts',(1.96792030384476,-35.3497176962493,-8.23601266253125));
#52671=CARTESIAN_POINT('Ctrl Pts',(1.96638937419042,-35.3985953585765,-8.23017817576157));
#52672=CARTESIAN_POINT('Ctrl Pts',(1.96544075319438,-35.447711491921,-8.22730061263402));
#52673=CARTESIAN_POINT('Ctrl Pts',(1.9650528772274,-35.4968275462247,-8.22738250085497));
#52674=CARTESIAN_POINT('Ctrl Pts',(2.00055083481923,-35.2562298992234,-8.25032497229716));
#52675=CARTESIAN_POINT('Ctrl Pts',(1.99912539370006,-35.3032976000604,-8.238749237339));
#52676=CARTESIAN_POINT('Ctrl Pts',(1.99825185783193,-35.3510704148417,-8.22997224725792));
#52677=CARTESIAN_POINT('Ctrl Pts',(1.99793777759489,-35.399317719028,-8.22405070694943));
#52678=CARTESIAN_POINT('Ctrl Pts',(1.99818337980841,-35.4478025374972,-8.22101390379241));
#52679=CARTESIAN_POINT('Ctrl Pts',(1.99898528943331,-35.496287277138,-8.2208624116822));
#52680=CARTESIAN_POINT('Ctrl Pts',(2.02983724854675,-35.2580732139914,-8.24391392449866));
#52681=CARTESIAN_POINT('Ctrl Pts',(2.02896194525648,-35.3045999801645,-8.23250120504607));
#52682=CARTESIAN_POINT('Ctrl Pts',(2.02864185425062,-35.3518073286936,-8.22382046327515));
#52683=CARTESIAN_POINT('Ctrl Pts',(2.0288811566285,-35.3994727360757,-8.21792630872739));
#52684=CARTESIAN_POINT('Ctrl Pts',(2.02967872348038,-35.4473671370956,-8.21484706320934));
#52685=CARTESIAN_POINT('Ctrl Pts',(2.03102808564287,-35.4952614620131,-8.21458396353363));
#52686=CARTESIAN_POINT('Ctrl Pts',(1.88461534316315,-35.2526204924184,-8.2724222202528));
#52687=CARTESIAN_POINT('Ctrl Pts',(1.93258700263877,-35.2532511304555,-8.26408746050993));
#52688=CARTESIAN_POINT('Ctrl Pts',(1.98073381621476,-35.2553235421864,-8.25456655856178));
#52689=CARTESIAN_POINT('Ctrl Pts',(2.02882173043,-35.2583763205,-8.24404472212));
#52690=CARTESIAN_POINT('Ctrl Pts',(9.26569107955,-35.2394341184,0.579579770152));
#52691=CARTESIAN_POINT('Ctrl Pts',(9.25048970237,-35.2934597015,0.575763550708));
#52692=CARTESIAN_POINT('Ctrl Pts',(9.23904466522,-35.3485828761,0.57252289393));
#52693=CARTESIAN_POINT('Ctrl Pts',(9.23145625045,-35.4044474883,0.569882968796));
#52694=CARTESIAN_POINT('Ctrl Pts',(9.22777481195,-35.4606828414,0.567861292872));
#52695=CARTESIAN_POINT('Ctrl Pts',(9.22799880569,-35.5169181946,0.566467047136));
#52696=CARTESIAN_POINT('Ctrl Pts',(9.26734254057,-35.2397154298,0.568265288566));
#52697=CARTESIAN_POINT('Ctrl Pts',(9.25220700276,-35.2936330337,0.564453943744));
#52698=CARTESIAN_POINT('Ctrl Pts',(9.24081265384,-35.3486411511,0.561212799914));
#52699=CARTESIAN_POINT('Ctrl Pts',(9.23325890658,-35.4043858824,0.558566884261));
#52700=CARTESIAN_POINT('Ctrl Pts',(9.22959566517,-35.4604989426,0.556533678149));
#52701=CARTESIAN_POINT('Ctrl Pts',(9.22982138229,-35.5166120028,0.55512243494));
#52702=CARTESIAN_POINT('Ctrl Pts',(9.26898307793,-35.2399973473,0.556947742073));
#52703=CARTESIAN_POINT('Ctrl Pts',(9.25391368938,-35.2938057049,0.55314265644));
#52704=CARTESIAN_POINT('Ctrl Pts',(9.24257020144,-35.3486974567,0.549902346095));
#52705=CARTESIAN_POINT('Ctrl Pts',(9.23505116442,-35.4043209585,0.547251660046));
#52706=CARTESIAN_POINT('Ctrl Pts',(9.23140601814,-35.4603103757,0.54520808798));
#52707=CARTESIAN_POINT('Ctrl Pts',(9.23163322063,-35.516299793,0.543780919912));
#52708=CARTESIAN_POINT('Ctrl Pts',(9.2706134925,-35.2402652369,0.545649357377));
#52709=CARTESIAN_POINT('Ctrl Pts',(9.25560999309,-35.2939662109,0.541842800001));
#52710=CARTESIAN_POINT('Ctrl Pts',(9.24431742891,-35.3487436319,0.53859575027));
#52711=CARTESIAN_POINT('Ctrl Pts',(9.23683343793,-35.4042480754,0.535933346844));
#52712=CARTESIAN_POINT('Ctrl Pts',(9.23320713925,-35.460116063,0.533872309581));
#52713=CARTESIAN_POINT('Ctrl Pts',(9.23343691736,-35.5159840505,0.532422414623));
#52714=CARTESIAN_POINT('Ctrl Pts',(9.2722446143,-35.2405353461,0.534265835364));
#52715=CARTESIAN_POINT('Ctrl Pts',(9.25730181761,-35.294127701,0.530496224362));
#52716=CARTESIAN_POINT('Ctrl Pts',(9.24605472348,-35.3487894773,0.527280786202));
#52717=CARTESIAN_POINT('Ctrl Pts',(9.2386001998,-35.4041734976,0.524643949807));
#52718=CARTESIAN_POINT('Ctrl Pts',(9.23498684878,-35.4599186602,0.522602910424));
#52719=CARTESIAN_POINT('Ctrl Pts',(9.23521314025,-35.5156638228,0.521166956934));
#52720=CARTESIAN_POINT('Ctrl Pts',(9.27386188355,-35.2408046483,0.522899878387));
#52721=CARTESIAN_POINT('Ctrl Pts',(9.25898070438,-35.2942887003,0.519158423034));
#52722=CARTESIAN_POINT('Ctrl Pts',(9.24778011027,-35.34883522,0.515965854318));
#52723=CARTESIAN_POINT('Ctrl Pts',(9.24035614735,-35.4040992464,0.513346314134));
#52724=CARTESIAN_POINT('Ctrl Pts',(9.23675700648,-35.4597220466,0.511316806589));
#52725=CARTESIAN_POINT('Ctrl Pts',(9.23698117862,-35.5153448469,0.509886547139));
#52726=CARTESIAN_POINT('',(9.26569106343796,-35.239434108596,0.579579885999606));
#52727=CARTESIAN_POINT('Origin',(10.2153393707933,-35.5169183517482,0.725089002244375));
#52728=CARTESIAN_POINT('Ctrl Pts',(9.27386188241726,-35.2408046523711,0.522899878102206));
#52729=CARTESIAN_POINT('Ctrl Pts',(9.27283706818152,-35.2406340032975,0.530102139560715));
#52730=CARTESIAN_POINT('Ctrl Pts',(9.27180627580663,-35.2404633709726,0.537307422065));
#52731=CARTESIAN_POINT('Ctrl Pts',(9.27077304606167,-35.2402915867397,0.544494586134051));
#52732=CARTESIAN_POINT('Ctrl Pts',(9.26926926806017,-35.2400415694016,0.554954892056214));
#52733=CARTESIAN_POINT('Ctrl Pts',(9.26775968832857,-35.2397868315245,0.565385481138434));
#52734=CARTESIAN_POINT('Ctrl Pts',(9.26623927281631,-35.2395275672319,0.575820625922912));
#52735=CARTESIAN_POINT('Ctrl Pts',(9.26605669997065,-35.2394964345453,0.577073687380689));
#52736=CARTESIAN_POINT('Ctrl Pts',(9.26587397022987,-35.2394652727112,0.578326749393097));
#52737=CARTESIAN_POINT('Ctrl Pts',(9.26569107942698,-35.2394341188372,0.579579770121116));
#52738=CARTESIAN_POINT('Ctrl Pts',(8.84973117353,-35.1509193731,2.1670354781));
#52739=CARTESIAN_POINT('Ctrl Pts',(8.80995437067,-35.2405490067,2.13392896451));
#52740=CARTESIAN_POINT('Ctrl Pts',(8.78039938016,-35.3367791654,2.10641082417));
#52741=CARTESIAN_POINT('Ctrl Pts',(8.76195606614,-35.4376104406,2.08522113231));
#52742=CARTESIAN_POINT('Ctrl Pts',(8.75504494547,-35.5407438285,2.07084302459));
#52743=CARTESIAN_POINT('Ctrl Pts',(8.75956295656,-35.6438772164,2.06344039042));
#52744=CARTESIAN_POINT('Ctrl Pts',(8.91091202313,-35.1598372898,2.04459467569));
#52745=CARTESIAN_POINT('Ctrl Pts',(8.87455647002,-35.246237181,2.01484191076));
#52746=CARTESIAN_POINT('Ctrl Pts',(8.84773035639,-35.3382711138,1.98987130618));
#52747=CARTESIAN_POINT('Ctrl Pts',(8.83115765576,-35.4342118768,1.97027362582));
#52748=CARTESIAN_POINT('Ctrl Pts',(8.82517322934,-35.532107067,1.95644630565));
#52749=CARTESIAN_POINT('Ctrl Pts',(8.82968488575,-35.6300022572,1.94854820039));
#52750=CARTESIAN_POINT('Ctrl Pts',(8.96795816735,-35.1710296589,1.91634945111));
#52751=CARTESIAN_POINT('Ctrl Pts',(8.93494048323,-35.2532459987,1.89161496085));
#52752=CARTESIAN_POINT('Ctrl Pts',(8.91060835461,-35.3400086156,1.87063336475));
#52753=CARTESIAN_POINT('Ctrl Pts',(8.89552405555,-35.4299031373,1.85381398232));
#52754=CARTESIAN_POINT('Ctrl Pts',(8.88994864311,-35.5213641494,1.84144178963));
#52755=CARTESIAN_POINT('Ctrl Pts',(8.89381707546,-35.6128251616,1.83365112687));
#52756=CARTESIAN_POINT('Ctrl Pts',(9.01653709076,-35.1835781664,1.78332507658));
#52757=CARTESIAN_POINT('Ctrl Pts',(8.98711360766,-35.260897748,1.76325201128));
#52758=CARTESIAN_POINT('Ctrl Pts',(8.96538998881,-35.341846639,1.74604152846));
#52759=CARTESIAN_POINT('Ctrl Pts',(8.95179602076,-35.4252853121,1.73198094156));
#52760=CARTESIAN_POINT('Ctrl Pts',(8.94653331601,-35.5099692034,1.72127486801));
#52761=CARTESIAN_POINT('Ctrl Pts',(8.9495584777,-35.5946530947,1.71402843838));
#52762=CARTESIAN_POINT('Ctrl Pts',(9.1140028877,-35.2108461818,1.46157810716));
#52763=CARTESIAN_POINT('Ctrl Pts',(9.09197113076,-35.2771127336,1.45066936239));
#52764=CARTESIAN_POINT('Ctrl Pts',(9.07556758896,-35.3453927996,1.44108450365));
#52765=CARTESIAN_POINT('Ctrl Pts',(9.06500040952,-35.4150382685,1.43291495679));
#52766=CARTESIAN_POINT('Ctrl Pts',(9.06037122564,-35.4853665076,1.42623124853));
#52767=CARTESIAN_POINT('Ctrl Pts',(9.06167021042,-35.5556947466,1.4210802448));
#52768=CARTESIAN_POINT('Ctrl Pts',(9.17852891179,-35.2281865303,1.13254165139));
#52769=CARTESIAN_POINT('Ctrl Pts',(9.16069403398,-35.2869558429,1.12639249526));
#52770=CARTESIAN_POINT('Ctrl Pts',(9.14729128577,-35.3471459486,1.12104732689));
#52771=CARTESIAN_POINT('Ctrl Pts',(9.13845933491,-35.4082985485,1.1165532711));
#52772=CARTESIAN_POINT('Ctrl Pts',(9.13426752236,-35.4699324162,1.11294417189));
#52773=CARTESIAN_POINT('Ctrl Pts',(9.13471251897,-35.531566284,1.1102388653));
#52774=CARTESIAN_POINT('Ctrl Pts',(9.20897519651,-35.2324135956,0.943972367435));
#52775=CARTESIAN_POINT('Ctrl Pts',(9.19209813045,-35.2892087111,0.939475719579));
#52776=CARTESIAN_POINT('Ctrl Pts',(9.17938477515,-35.3472963111,0.935686471687));
#52777=CARTESIAN_POINT('Ctrl Pts',(9.17095916069,-35.4062580486,0.93263706468));
#52778=CARTESIAN_POINT('Ctrl Pts',(9.16688368582,-35.4656570006,0.930349922162));
#52779=CARTESIAN_POINT('Ctrl Pts',(9.1671566108,-35.5250559527,0.928836133483));
#52780=CARTESIAN_POINT('Ctrl Pts',(9.23916608575,-35.2348774759,0.761379139513));
#52781=CARTESIAN_POINT('Ctrl Pts',(9.22290027765,-35.2906450094,0.757499573794));
#52782=CARTESIAN_POINT('Ctrl Pts',(9.21063507987,-35.3476242625,0.754282164424));
#52783=CARTESIAN_POINT('Ctrl Pts',(9.20248495391,-35.4054228352,0.75175437252));
#52784=CARTESIAN_POINT('Ctrl Pts',(9.19850755669,-35.4636310173,0.749934120027));
#52785=CARTESIAN_POINT('Ctrl Pts',(9.19870123297,-35.5218391995,0.748829315604));
#52786=CARTESIAN_POINT('Ctrl Pts',(9.26569123725,-35.2394333704,0.579580156823));
#52787=CARTESIAN_POINT('Ctrl Pts',(9.25048972376,-35.2934591001,0.575764245003));
#52788=CARTESIAN_POINT('Ctrl Pts',(9.23904456924,-35.3485824305,0.57252390595));
#52789=CARTESIAN_POINT('Ctrl Pts',(9.2314560575,-35.4044472049,0.569884306758));
#52790=CARTESIAN_POINT('Ctrl Pts',(9.22777454338,-35.4606827234,0.567862962924));
#52791=CARTESIAN_POINT('Ctrl Pts',(9.22799848318,-35.5169182418,0.566469053265));
#52792=CARTESIAN_POINT('',(8.84973118842306,-35.1509193774195,2.16703548709451));
#52793=CARTESIAN_POINT('Origin',(9.6131533587965,-35.6438801033176,2.58440681741808));
#52794=CARTESIAN_POINT('Ctrl Pts',(9.26569102913818,-35.2394341100243,0.579580104582361));
#52795=CARTESIAN_POINT('Ctrl Pts',(9.26403312974663,-35.239148763037,0.590944194137194));
#52796=CARTESIAN_POINT('Ctrl Pts',(9.26158621847309,-35.2387686053236,0.607559540293847));
#52797=CARTESIAN_POINT('Ctrl Pts',(9.25830217899466,-35.2382951410448,0.629427757030632));
#52798=CARTESIAN_POINT('Ctrl Pts',(9.25728445574588,-35.2381484145492,0.636204713498013));
#52799=CARTESIAN_POINT('Ctrl Pts',(9.25618617187326,-35.2379926909596,0.643486454517567));
#52800=CARTESIAN_POINT('Ctrl Pts',(9.25500551801042,-35.2378276994222,0.651274021297969));
#52801=CARTESIAN_POINT('Ctrl Pts',(9.25251029507681,-35.2374790022462,0.667732456610143));
#52802=CARTESIAN_POINT('Ctrl Pts',(9.24964752807473,-35.2370897742068,0.686448362167339));
#52803=CARTESIAN_POINT('Ctrl Pts',(9.24639629512545,-35.2366600504234,0.707433024476164));
#52804=CARTESIAN_POINT('Ctrl Pts',(9.24477067865081,-35.2364451885317,0.717925355630576));
#52805=CARTESIAN_POINT('Ctrl Pts',(9.24304788749146,-35.2362201852664,0.728984866587668));
#52806=CARTESIAN_POINT('Ctrl Pts',(9.24122449748462,-35.2359850638432,0.740613678664237));
#52807=CARTESIAN_POINT('Ctrl Pts',(9.2403128024812,-35.2358675031317,0.746428084702522));
#52808=CARTESIAN_POINT('Ctrl Pts',(9.23937594908501,-35.2357474102751,0.75238481461629));
#52809=CARTESIAN_POINT('Ctrl Pts',(9.23841343596212,-35.2356247874065,0.758484137541625));
#52810=CARTESIAN_POINT('Ctrl Pts',(9.23745092283922,-35.2355021645378,0.764583460466961));
#52811=CARTESIAN_POINT('Ctrl Pts',(9.23624270504607,-35.23534931158,0.772210386989164));
#52812=CARTESIAN_POINT('Ctrl Pts',(9.23544835714733,-35.2352493232179,0.777210152233157));
#52813=CARTESIAN_POINT('Ctrl Pts',(9.2296892981416,-35.2345244029677,0.813458681499608));
#52814=CARTESIAN_POINT('Ctrl Pts',(9.2242637536647,-35.2338115087621,0.84699597042143));
#52815=CARTESIAN_POINT('Ctrl Pts',(9.21920351523641,-35.2331082401535,0.87779962226023));
#52816=CARTESIAN_POINT('Ctrl Pts',(9.21868007791685,-35.2330354931791,0.880985990092489));
#52817=CARTESIAN_POINT('Ctrl Pts',(9.2181605375375,-35.2329628898038,0.884143095226426));
#52818=CARTESIAN_POINT('Ctrl Pts',(9.21764492303421,-35.2328904534041,0.887270906919236));
#52819=CARTESIAN_POINT('Ctrl Pts',(9.2148948094202,-35.2325041021135,0.903953598084017));
#52820=CARTESIAN_POINT('Ctrl Pts',(9.21225671553722,-35.2321211437485,0.919803009731216));
#52821=CARTESIAN_POINT('Ctrl Pts',(9.20973657646034,-35.23174158003,0.934814873904563));
#52822=CARTESIAN_POINT('Ctrl Pts',(9.20847650692191,-35.2315517981708,0.942320805991237));
#52823=CARTESIAN_POINT('Ctrl Pts',(9.20724593921839,-35.2313628690998,0.949617353531283));
#52824=CARTESIAN_POINT('Ctrl Pts',(9.2060456977663,-35.2311747873243,0.956704051708735));
#52825=CARTESIAN_POINT('Ctrl Pts',(9.20492302971948,-35.230998861556,0.963332725953723));
#52826=CARTESIAN_POINT('Ctrl Pts',(9.20413921238186,-35.2308745790399,0.967947012534467));
#52827=CARTESIAN_POINT('Ctrl Pts',(9.20281860737665,-35.230659138175,0.975683911631795));
#52828=CARTESIAN_POINT('Ctrl Pts',(9.20272735704886,-35.2306442517786,0.976218510982836));
#52829=CARTESIAN_POINT('Ctrl Pts',(9.20263352908835,-35.2306289206566,0.976768030388192));
#52830=CARTESIAN_POINT('Ctrl Pts',(9.20253682703764,-35.2306130927847,0.977334170225671));
#52831=CARTESIAN_POINT('Ctrl Pts',(9.19494660137613,-35.2293707497539,1.02177096438316));
#52832=CARTESIAN_POINT('Ctrl Pts',(9.18720958723024,-35.227937253375,1.06580927001366));
#52833=CARTESIAN_POINT('Ctrl Pts',(9.17923290862162,-35.2263185653215,1.1093899606357));
#52834=CARTESIAN_POINT('Ctrl Pts',(9.17463050828737,-35.2253846113785,1.13453523662425));
#52835=CARTESIAN_POINT('Ctrl Pts',(9.16994791914426,-35.2243897599338,1.15952755468674));
#52836=CARTESIAN_POINT('Ctrl Pts',(9.1651653249338,-35.2233416856826,1.18435181583264));
#52837=CARTESIAN_POINT('Ctrl Pts',(9.15590037782223,-35.2213113331001,1.23244192268248));
#52838=CARTESIAN_POINT('Ctrl Pts',(9.14628071238575,-35.2190081024355,1.27991064809126));
#52839=CARTESIAN_POINT('Ctrl Pts',(9.13619487560413,-35.216439543141,1.32666161021856));
#52840=CARTESIAN_POINT('Ctrl Pts',(9.1344163009029,-35.2159865936556,1.33490585214889));
#52841=CARTESIAN_POINT('Ctrl Pts',(9.13262326977988,-35.2155255178236,1.34312777745214));
#52842=CARTESIAN_POINT('Ctrl Pts',(9.1308152324794,-35.2150565146126,1.3513268688895));
#52843=CARTESIAN_POINT('Ctrl Pts',(9.13034074638857,-35.2149334333576,1.35347856943432));
#52844=CARTESIAN_POINT('Ctrl Pts',(9.1298652269346,-35.2148098063821,1.35562869749501));
#52845=CARTESIAN_POINT('Ctrl Pts',(9.12938866444621,-35.2146856377966,1.35777724388487));
#52846=CARTESIAN_POINT('Ctrl Pts',(9.12915808535601,-35.2146255603037,1.35881679249367));
#52847=CARTESIAN_POINT('Ctrl Pts',(9.12892834647673,-35.2145656396722,1.35985110818999));
#52848=CARTESIAN_POINT('Ctrl Pts',(9.12869331410367,-35.2145042736238,1.36090772293837));
#52849=CARTESIAN_POINT('Ctrl Pts',(9.12716376995017,-35.2141049155298,1.36778396253803));
#52850=CARTESIAN_POINT('Ctrl Pts',(9.12545911347254,-35.2136565503212,1.37536892283862));
#52851=CARTESIAN_POINT('Ctrl Pts',(9.12407478426825,-35.2132904462239,1.38147563434889));
#52852=CARTESIAN_POINT('Ctrl Pts',(9.12389028593192,-35.213241653208,1.38228951453764));
#52853=CARTESIAN_POINT('Ctrl Pts',(9.12371152874733,-35.2131943436618,1.38307714187556));
#52854=CARTESIAN_POINT('Ctrl Pts',(9.12353972887807,-35.2131488468471,1.38383334339462));
#52855=CARTESIAN_POINT('Ctrl Pts',(9.12344070744131,-35.2131226235444,1.38426920030895));
#52856=CARTESIAN_POINT('Ctrl Pts',(9.12334213194895,-35.2130965085466,1.3847028303091));
#52857=CARTESIAN_POINT('Ctrl Pts',(9.12324311753217,-35.2130702675231,1.38513812626634));
#52858=CARTESIAN_POINT('Ctrl Pts',(9.11672349360445,-35.2113424221221,1.41380027497812));
#52859=CARTESIAN_POINT('Ctrl Pts',(9.10953876734521,-35.2093940202451,1.44425287213694));
#52860=CARTESIAN_POINT('Ctrl Pts',(9.10153909374284,-35.207196182716,1.47643777477174));
#52861=CARTESIAN_POINT('Ctrl Pts',(9.09880004859498,-35.2064436549856,1.48745771205645));
#52862=CARTESIAN_POINT('Ctrl Pts',(9.09596512280942,-35.2056620167299,1.49868049535259));
#52863=CARTESIAN_POINT('Ctrl Pts',(9.09302722159292,-35.2048506613793,1.51010300502745));
#52864=CARTESIAN_POINT('Ctrl Pts',(9.08824275573008,-35.203529343305,1.52870492646046));
#52865=CARTESIAN_POINT('Ctrl Pts',(9.08318537894781,-35.2021290648566,1.54783677119873));
#52866=CARTESIAN_POINT('Ctrl Pts',(9.0778220040167,-35.2006482493061,1.56748158480479));
#52867=CARTESIAN_POINT('Ctrl Pts',(9.06907659420416,-35.1982336616607,1.59951401734633));
#52868=CARTESIAN_POINT('Ctrl Pts',(9.05951839809739,-35.1956030107588,1.63291380893745));
#52869=CARTESIAN_POINT('Ctrl Pts',(9.04897509399545,-35.1927822459941,1.66759275186022));
#52870=CARTESIAN_POINT('Ctrl Pts',(9.04841969275742,-35.192633653463,1.669419572717));
#52871=CARTESIAN_POINT('Ctrl Pts',(9.04786155274224,-35.1924845407158,1.67124993504131));
#52872=CARTESIAN_POINT('Ctrl Pts',(9.04730064717397,-35.1923349140887,1.67308382316031));
#52873=CARTESIAN_POINT('Ctrl Pts',(9.04169629738177,-35.1908399031566,1.69140731837926));
#52874=CARTESIAN_POINT('Ctrl Pts',(9.03580768079979,-35.1893154100858,1.71007792331351));
#52875=CARTESIAN_POINT('Ctrl Pts',(9.02961873353496,-35.1877372787726,1.72908730537306));
#52876=CARTESIAN_POINT('Ctrl Pts',(9.02652425990255,-35.1869482131159,1.73859199640283));
#52877=CARTESIAN_POINT('Ctrl Pts',(9.02335473459722,-35.1861456853932,1.74818142355523));
#52878=CARTESIAN_POINT('Ctrl Pts',(9.02010710682159,-35.1853296928105,1.75785384236612));
#52879=CARTESIAN_POINT('Ctrl Pts',(9.01848329293377,-35.1849216965191,1.76269005177156));
#52880=CARTESIAN_POINT('Ctrl Pts',(9.01683995395626,-35.1845103342624,1.76754700928818));
#52881=CARTESIAN_POINT('Ctrl Pts',(9.01517671455472,-35.1840956050493,1.77242449837224));
#52882=CARTESIAN_POINT('Ctrl Pts',(9.01369720400855,-35.183726688678,1.77676319822028));
#52883=CARTESIAN_POINT('Ctrl Pts',(9.01254229787951,-35.1834395465047,1.78013185822244));
#52884=CARTESIAN_POINT('Ctrl Pts',(9.01080363646111,-35.1830088514207,1.78516241231019));
#52885=CARTESIAN_POINT('Ctrl Pts',(9.01058772568367,-35.1829553667633,1.7857871175188));
#52886=CARTESIAN_POINT('Ctrl Pts',(9.01036275395945,-35.1828996662518,1.78643742390526));
#52887=CARTESIAN_POINT('Ctrl Pts',(9.01012692462632,-35.1828413166113,1.78711834497098));
#52888=CARTESIAN_POINT('Ctrl Pts',(8.99742837262227,-35.1796994006595,1.82378346821384));
#52889=CARTESIAN_POINT('Ctrl Pts',(8.98486577871898,-35.1767195613466,1.85788716927598));
#52890=CARTESIAN_POINT('Ctrl Pts',(8.9726706290217,-35.1739608658519,1.88948106381597));
#52891=CARTESIAN_POINT('Ctrl Pts',(8.96009192469607,-35.1711154054997,1.92206863082239));
#52892=CARTESIAN_POINT('Ctrl Pts',(8.94790633959043,-35.1685046108467,1.9519871584884));
#52893=CARTESIAN_POINT('Ctrl Pts',(8.93635103932819,-35.1661507431013,1.97932121069418));
#52894=CARTESIAN_POINT('Ctrl Pts',(8.92494704640639,-35.1638276973562,2.00629734552448));
#52895=CARTESIAN_POINT('Ctrl Pts',(8.91415801263107,-35.1617538398625,2.03075731440233));
#52896=CARTESIAN_POINT('Ctrl Pts',(8.90417118313868,-35.1599231615189,2.05279228655344));
#52897=CARTESIAN_POINT('Ctrl Pts',(8.89418444606352,-35.1580925001162,2.07482705479488));
#52898=CARTESIAN_POINT('Ctrl Pts',(8.88500010790469,-35.15650417239,2.09443764578029));
#52899=CARTESIAN_POINT('Ctrl Pts',(8.8767549321914,-35.1551387966204,2.11171147529049));
#52900=CARTESIAN_POINT('Ctrl Pts',(8.8682619698602,-35.1537323881481,2.1295044233667));
#52901=CARTESIAN_POINT('Ctrl Pts',(8.8607651973453,-35.1525618856043,2.14481872320988));
#52902=CARTESIAN_POINT('Ctrl Pts',(8.8543606995376,-35.1516033707736,2.15773475299162));
#52903=CARTESIAN_POINT('Ctrl Pts',(8.85274816285252,-35.1513620340796,2.16098677562852));
#52904=CARTESIAN_POINT('Ctrl Pts',(8.85120462911029,-35.1511341487073,2.16408666184874));
#52905=CARTESIAN_POINT('Ctrl Pts',(8.84973117353,-35.1509193731,2.1670354781));
#52906=CARTESIAN_POINT('Ctrl Pts',(8.84972761074,-35.1509187546,2.16704276679));
#52907=CARTESIAN_POINT('Ctrl Pts',(8.80995141052,-35.2405485577,2.13393459289));
#52908=CARTESIAN_POINT('Ctrl Pts',(8.78039709025,-35.3367789605,2.10641485522));
#52909=CARTESIAN_POINT('Ctrl Pts',(8.7619545083,-35.4376105338,2.08522367244));
#52910=CARTESIAN_POINT('Ctrl Pts',(8.75504416849,-35.5407442468,2.0708442184));
#52911=CARTESIAN_POINT('Ctrl Pts',(8.75956299023,-35.6438779598,2.0634404101));
#52912=CARTESIAN_POINT('Ctrl Pts',(8.84456885861,-35.1501669799,2.17736664036));
#52913=CARTESIAN_POINT('Ctrl Pts',(8.80450316343,-35.2400691335,2.14397755154));
#52914=CARTESIAN_POINT('Ctrl Pts',(8.77471769299,-35.3366533562,2.11624485706));
#52915=CARTESIAN_POINT('Ctrl Pts',(8.75611631291,-35.437897274,2.0949212219));
#52916=CARTESIAN_POINT('Ctrl Pts',(8.74912677261,-35.5414726393,2.08049700356));
#52917=CARTESIAN_POINT('Ctrl Pts',(8.75364509765,-35.6450480046,2.07313650893));
#52918=CARTESIAN_POINT('Ctrl Pts',(8.83934134903,-35.1494257084,2.1877279664));
#52919=CARTESIAN_POINT('Ctrl Pts',(8.79900028815,-35.2395949404,2.15403728116));
#52920=CARTESIAN_POINT('Ctrl Pts',(8.76899769743,-35.3365278505,2.12607022447));
#52921=CARTESIAN_POINT('Ctrl Pts',(8.75025126803,-35.4381791278,2.10459258862));
#52922=CARTESIAN_POINT('Ctrl Pts',(8.74319574656,-35.5421912387,2.09010248095));
#52923=CARTESIAN_POINT('Ctrl Pts',(8.74772599292,-35.6462033496,2.08276502103));
#52924=CARTESIAN_POINT('Ctrl Pts',(8.83403961773,-35.1487041475,2.19812825065));
#52925=CARTESIAN_POINT('Ctrl Pts',(8.79343976066,-35.2391345884,2.16411346789));
#52926=CARTESIAN_POINT('Ctrl Pts',(8.76323651939,-35.3364102747,2.1358885387));
#52927=CARTESIAN_POINT('Ctrl Pts',(8.74436113276,-35.4384630225,2.11423302609));
#52928=CARTESIAN_POINT('Ctrl Pts',(8.73725504684,-35.5429059973,2.0996533862));
#52929=CARTESIAN_POINT('Ctrl Pts',(8.74181161845,-35.6473489721,2.09231606717));
#52930=CARTESIAN_POINT('Ctrl Pts',(8.82866432718,-35.1480081194,2.20856250217));
#52931=CARTESIAN_POINT('Ctrl Pts',(8.78782272692,-35.2386939519,2.17420118315));
#52932=CARTESIAN_POINT('Ctrl Pts',(8.75743582295,-35.3363065177,2.14569487681));
#52933=CARTESIAN_POINT('Ctrl Pts',(8.73844810187,-35.4387548314,2.12383756828));
#52934=CARTESIAN_POINT('Ctrl Pts',(8.73130736324,-35.5436227636,2.10914471028));
#52935=CARTESIAN_POINT('Ctrl Pts',(8.73590510583,-35.6484906957,2.1017846051));
#52936=CARTESIAN_POINT('Ctrl Pts',(8.82321744436,-35.1473421125,2.21902489656));
#52937=CARTESIAN_POINT('Ctrl Pts',(8.78215104537,-35.2382777414,2.18429511356));
#52938=CARTESIAN_POINT('Ctrl Pts',(8.75159740651,-35.3362215383,2.15548447298));
#52939=CARTESIAN_POINT('Ctrl Pts',(8.73251395256,-35.4390597803,2.13340204369));
#52940=CARTESIAN_POINT('Ctrl Pts',(8.72535447592,-35.5443470397,2.11857293178));
#52941=CARTESIAN_POINT('Ctrl Pts',(8.73000824887,-35.6496342991,2.1111678244));
#52942=CARTESIAN_POINT('',(8.82321718811955,-35.1473420531381,2.21902512680689));
#52943=CARTESIAN_POINT('Origin',(9.57670448652795,-35.6496380550362,2.64327392285592));
#52944=CARTESIAN_POINT('Ctrl Pts',(8.84972757036633,-35.1509188455761,2.16704273318452));
#52945=CARTESIAN_POINT('Ctrl Pts',(8.84266601721309,-35.1498897248256,2.18117462196919));
#52946=CARTESIAN_POINT('Ctrl Pts',(8.83544640067731,-35.148886344665,2.19539418957044));
#52947=CARTESIAN_POINT('Ctrl Pts',(8.82806096535708,-35.1479465542617,2.20968655179896));
#52948=CARTESIAN_POINT('Ctrl Pts',(8.82645413028913,-35.1477420858572,2.21279611377288));
#52949=CARTESIAN_POINT('Ctrl Pts',(8.82483957760491,-35.1475405449177,2.21590899096587));
#52950=CARTESIAN_POINT('Ctrl Pts',(8.82321740410989,-35.1473422016281,2.21902486252055));
#52951=CARTESIAN_POINT('Ctrl Pts',(8.82321783753,-35.1473399652,2.21902634713));
#52952=CARTESIAN_POINT('Ctrl Pts',(8.78215068074,-35.2382758927,2.18429700681));
#52953=CARTESIAN_POINT('Ctrl Pts',(8.75159630524,-35.3362200688,2.15548691366));
#52954=CARTESIAN_POINT('Ctrl Pts',(8.73251216058,-35.4390587483,2.13340513227));
#52955=CARTESIAN_POINT('Ctrl Pts',(8.72535205902,-35.5443464741,2.11857675734));
#52956=CARTESIAN_POINT('Ctrl Pts',(8.73000528472,-35.6496341999,2.11117245845));
#52957=CARTESIAN_POINT('Ctrl Pts',(8.7950132494,-35.1439026605,2.27318832802));
#52958=CARTESIAN_POINT('Ctrl Pts',(8.75278762749,-35.2361296908,2.23654747651));
#52959=CARTESIAN_POINT('Ctrl Pts',(8.72137526051,-35.3357860213,2.20615712169));
#52960=CARTESIAN_POINT('Ctrl Pts',(8.70180041036,-35.4406403454,2.18290446914));
#52961=CARTESIAN_POINT('Ctrl Pts',(8.69454777529,-35.548095721,2.16736469093));
#52962=CARTESIAN_POINT('Ctrl Pts',(8.69949502688,-35.6555510966,2.15972094562));
#52963=CARTESIAN_POINT('Ctrl Pts',(8.76584958693,-35.140386513,2.32745356943));
#52964=CARTESIAN_POINT('Ctrl Pts',(8.72246681666,-35.2339199765,2.28869203429));
#52965=CARTESIAN_POINT('Ctrl Pts',(8.69020329348,-35.3353435452,2.25654623894));
#52966=CARTESIAN_POINT('Ctrl Pts',(8.67015581074,-35.4422984936,2.23199348318));
#52967=CARTESIAN_POINT('Ctrl Pts',(8.66284221447,-35.5520214947,2.21566670729));
#52968=CARTESIAN_POINT('Ctrl Pts',(8.66812648429,-35.6617444959,2.20776307897));
#52969=CARTESIAN_POINT('Ctrl Pts',(8.7356657971,-35.1367480171,2.38172554964));
#52970=CARTESIAN_POINT('Ctrl Pts',(8.69113780582,-35.2316121539,2.34057114953));
#52971=CARTESIAN_POINT('Ctrl Pts',(8.65803763705,-35.3348781572,2.30644499517));
#52972=CARTESIAN_POINT('Ctrl Pts',(8.63754180367,-35.4440469154,2.28042962134));
#52973=CARTESIAN_POINT('Ctrl Pts',(8.63020353714,-35.5561701517,2.26322602866));
#52974=CARTESIAN_POINT('Ctrl Pts',(8.63587110442,-35.668293388,2.25504712403));
#52975=CARTESIAN_POINT('Ctrl Pts',(8.69114735744,-35.1314764865,2.45847308227));
#52976=CARTESIAN_POINT('Ctrl Pts',(8.64510845073,-35.2282535188,2.41340322951));
#52977=CARTESIAN_POINT('Ctrl Pts',(8.61094346222,-35.3342411346,2.37601936382));
#52978=CARTESIAN_POINT('Ctrl Pts',(8.58994905716,-35.4467225347,2.34758564448));
#52979=CARTESIAN_POINT('Ctrl Pts',(8.58273119234,-35.5624541016,2.32891916373));
#52980=CARTESIAN_POINT('Ctrl Pts',(8.58910725848,-35.6781856686,2.32025995821));
#52981=CARTESIAN_POINT('Ctrl Pts',(8.64411242258,-35.1256902423,2.53413655954));
#52982=CARTESIAN_POINT('Ctrl Pts',(8.59671994041,-35.2244531785,2.48429647903));
#52983=CARTESIAN_POINT('Ctrl Pts',(8.56161211733,-35.333412859,2.44298795985));
#52984=CARTESIAN_POINT('Ctrl Pts',(8.54022333506,-35.4495924912,2.41171677405));
#52985=CARTESIAN_POINT('Ctrl Pts',(8.53321738738,-35.5693865938,2.39145291764));
#52986=CARTESIAN_POINT('Ctrl Pts',(8.54037362589,-35.6891806965,2.38246370607));
#52987=CARTESIAN_POINT('Ctrl Pts',(8.62993676763,-35.1239763388,2.55637951988));
#52988=CARTESIAN_POINT('Ctrl Pts',(8.58219189761,-35.2233231665,2.50503392418));
#52989=CARTESIAN_POINT('Ctrl Pts',(8.54685013234,-35.3331714269,2.46248222847));
#52990=CARTESIAN_POINT('Ctrl Pts',(8.52538633662,-35.4504650834,2.43030855578));
#52991=CARTESIAN_POINT('Ctrl Pts',(8.51848133158,-35.5714859455,2.4095318701));
#52992=CARTESIAN_POINT('Ctrl Pts',(8.52590127043,-35.6925068075,2.40042817508));
#52993=CARTESIAN_POINT('Ctrl Pts',(8.61560772534,-35.1221440943,2.57842131078));
#52994=CARTESIAN_POINT('Ctrl Pts',(8.56749228928,-35.2220926432,2.52550930797));
#52995=CARTESIAN_POINT('Ctrl Pts',(8.53188890827,-35.3328708509,2.48168265536));
#52996=CARTESIAN_POINT('Ctrl Pts',(8.5103168202,-35.4513369446,2.44860878814));
#52997=CARTESIAN_POINT('Ctrl Pts',(8.50347493534,-35.5736522798,2.42735915225));
#52998=CARTESIAN_POINT('Ctrl Pts',(8.51111753906,-35.695967615,2.41821700034));
#52999=CARTESIAN_POINT('Ctrl Pts',(8.60091081429,-35.1203221009,2.60032838611));
#53000=CARTESIAN_POINT('Ctrl Pts',(8.55250194661,-35.2208633123,2.54573382886));
#53001=CARTESIAN_POINT('Ctrl Pts',(8.51670661225,-35.3325772847,2.50053061213));
#53002=CARTESIAN_POINT('Ctrl Pts',(8.49508702343,-35.4522342523,2.46647865078));
#53003=CARTESIAN_POINT('Ctrl Pts',(8.4883597474,-35.5758682626,2.44470657499));
#53004=CARTESIAN_POINT('Ctrl Pts',(8.49626469614,-35.699502273,2.4355053823));
#53005=CARTESIAN_POINT('',(8.60091080648026,-35.1203221517964,2.60032836406496));
#53006=CARTESIAN_POINT('Origin',(9.25479801252791,-35.6995101749192,3.0871775403849));
#53007=CARTESIAN_POINT('Ctrl Pts',(8.8232168869647,-35.1473420700646,2.219025543263));
#53008=CARTESIAN_POINT('Ctrl Pts',(8.79610687645427,-35.1440374725036,2.27108634121779));
#53009=CARTESIAN_POINT('Ctrl Pts',(8.76980417777782,-35.1408675387765,2.31968006431244));
#53010=CARTESIAN_POINT('Ctrl Pts',(8.74448255430243,-35.1378266460975,2.36475221674184));
#53011=CARTESIAN_POINT('Ctrl Pts',(8.72419021923815,-35.1353897244209,2.40087230280402));
#53012=CARTESIAN_POINT('Ctrl Pts',(8.7045250357025,-35.1330382006051,2.43472924958153));
#53013=CARTESIAN_POINT('Ctrl Pts',(8.68559135386596,-35.1307504362116,2.46631895241685));
#53014=CARTESIAN_POINT('Ctrl Pts',(8.6808987964871,-35.1301834326157,2.47414820054808));
#53015=CARTESIAN_POINT('Ctrl Pts',(8.67625129609282,-35.1296202164936,2.4818383635054));
#53016=CARTESIAN_POINT('Ctrl Pts',(8.67165065750585,-35.1290602421153,2.48938977693137));
#53017=CARTESIAN_POINT('Ctrl Pts',(8.6629063577104,-35.1279959151206,2.50374252853918));
#53018=CARTESIAN_POINT('Ctrl Pts',(8.6543265999625,-35.1269464169891,2.51759656768404));
#53019=CARTESIAN_POINT('Ctrl Pts',(8.64591696339239,-35.1259138536027,2.5309581417663));
#53020=CARTESIAN_POINT('Ctrl Pts',(8.63747144758885,-35.1248768848437,2.54437672224015));
#53021=CARTESIAN_POINT('Ctrl Pts',(8.62920242176465,-35.1238537026323,2.55729591434691));
#53022=CARTESIAN_POINT('Ctrl Pts',(8.62111895312701,-35.1228449173309,2.56972204618431));
#53023=CARTESIAN_POINT('Ctrl Pts',(8.61425477167297,-35.121988294306,2.58027385599854));
#53024=CARTESIAN_POINT('Ctrl Pts',(8.60752448890165,-35.1211420059566,2.59047010569892));
#53025=CARTESIAN_POINT('Ctrl Pts',(8.60091082397732,-35.1203221021009,2.60032837167017));
#53026=CARTESIAN_POINT('Ctrl Pts',(8.60091079918,-35.1203221982,2.60032832802));
#53027=CARTESIAN_POINT('Ctrl Pts',(8.55250196755,-35.2208633974,2.5457337616));
#53028=CARTESIAN_POINT('Ctrl Pts',(8.51670667214,-35.3325773527,2.50053052804));
#53029=CARTESIAN_POINT('Ctrl Pts',(8.49508712358,-35.4522342996,2.46647854203));
#53030=CARTESIAN_POINT('Ctrl Pts',(8.48835988758,-35.5758682873,2.44470643423));
#53031=CARTESIAN_POINT('Ctrl Pts',(8.49626487495,-35.6995022751,2.43550520334));
#53032=CARTESIAN_POINT('Ctrl Pts',(8.56160117875,-35.1140346808,2.66060541831));
#53033=CARTESIAN_POINT('Ctrl Pts',(8.51158038352,-35.2164638336,2.60178050099));
#53034=CARTESIAN_POINT('Ctrl Pts',(8.47440952478,-35.3311106273,2.55334779448));
#53035=CARTESIAN_POINT('Ctrl Pts',(8.45180416694,-35.454476252,2.51731779839));
#53036=CARTESIAN_POINT('Ctrl Pts',(8.44456120074,-35.5822080931,2.49495976327));
#53037=CARTESIAN_POINT('Ctrl Pts',(8.45240512852,-35.7099399342,2.48655698047));
#53038=CARTESIAN_POINT('Ctrl Pts',(8.51829161967,-35.1086508497,2.71924356476));
#53039=CARTESIAN_POINT('Ctrl Pts',(8.4676782837,-35.2126508331,2.65547482048));
#53040=CARTESIAN_POINT('Ctrl Pts',(8.42997337302,-35.3299187074,2.6031885652));
#53041=CARTESIAN_POINT('Ctrl Pts',(8.40701812301,-35.4566921944,2.56468900549));
#53042=CARTESIAN_POINT('Ctrl Pts',(8.39967272263,-35.5882267707,2.5414121675));
#53043=CARTESIAN_POINT('Ctrl Pts',(8.40764108873,-35.7197613468,2.53363446576));
#53044=CARTESIAN_POINT('Ctrl Pts',(8.47165311425,-35.1035435988,2.77475885702));
#53045=CARTESIAN_POINT('Ctrl Pts',(8.42103112523,-35.2090000749,2.7055559059));
#53046=CARTESIAN_POINT('Ctrl Pts',(8.38318247508,-35.3288584812,2.64914965253));
#53047=CARTESIAN_POINT('Ctrl Pts',(8.36006509714,-35.4590804193,2.60819117966));
#53048=CARTESIAN_POINT('Ctrl Pts',(8.35259991719,-35.5944943118,2.58430328363));
#53049=CARTESIAN_POINT('Ctrl Pts',(8.36047222003,-35.7299082045,2.5777319381));
#53050=CARTESIAN_POINT('Ctrl Pts',(8.35159188251,-35.0922845623,2.89275323394));
#53051=CARTESIAN_POINT('Ctrl Pts',(8.3050322624,-35.2005432762,2.80975608337));
#53052=CARTESIAN_POINT('Ctrl Pts',(8.26959869952,-35.3257180408,2.7430273545));
#53053=CARTESIAN_POINT('Ctrl Pts',(8.2473160419,-35.4631716043,2.69610840641));
#53054=CARTESIAN_POINT('Ctrl Pts',(8.23918506507,-35.6067794199,2.67107903223));
#53055=CARTESIAN_POINT('Ctrl Pts',(8.24494252704,-35.7503872354,2.66806485365));
#53056=CARTESIAN_POINT('Ctrl Pts',(8.20219946581,-35.0869079403,2.96964215712));
#53057=CARTESIAN_POINT('Ctrl Pts',(8.17044511261,-35.196070615,2.87494321335));
#53058=CARTESIAN_POINT('Ctrl Pts',(8.14524485361,-35.3234854768,2.79971065515));
#53059=CARTESIAN_POINT('Ctrl Pts',(8.12806473503,-35.4642227883,2.74824760952));
#53060=CARTESIAN_POINT('Ctrl Pts',(8.11972374517,-35.6116396625,2.72298240153));
#53061=CARTESIAN_POINT('Ctrl Pts',(8.12018530542,-35.7590565367,2.723855906));
#53062=CARTESIAN_POINT('Ctrl Pts',(8.10597427981,-35.0887550559,2.98941073315));
#53063=CARTESIAN_POINT('Ctrl Pts',(8.08828816032,-35.1976252196,2.89277147723));
#53064=CARTESIAN_POINT('Ctrl Pts',(8.07262669454,-35.3241767484,2.81647388405));
#53065=CARTESIAN_POINT('Ctrl Pts',(8.05970660483,-35.4635970156,2.76481016119));
#53066=CARTESIAN_POINT('Ctrl Pts',(8.05010223161,-35.6094680649,2.74015988873));
#53067=CARTESIAN_POINT('Ctrl Pts',(8.0441099093,-35.7553391142,2.74240669266));
#53068=CARTESIAN_POINT('Ctrl Pts',(7.82075728158,-35.1140008873,2.95981413055));
#53069=CARTESIAN_POINT('Ctrl Pts',(7.83753302833,-35.2174511648,2.88177682176));
#53070=CARTESIAN_POINT('Ctrl Pts',(7.84624727736,-35.3324220766,2.81978760483));
#53071=CARTESIAN_POINT('Ctrl Pts',(7.84611816579,-35.4555224941,2.77624706117));
#53072=CARTESIAN_POINT('Ctrl Pts',(7.83704746541,-35.5826911821,2.75255272839));
#53073=CARTESIAN_POINT('Ctrl Pts',(7.81966214074,-35.7098598702,2.74888110871));
#53074=CARTESIAN_POINT('Ctrl Pts',(7.56538653659,-35.1573736159,2.76989788484));
#53075=CARTESIAN_POINT('Ctrl Pts',(7.58792144694,-35.2456787757,2.72783328434));
#53076=CARTESIAN_POINT('Ctrl Pts',(7.60265321273,-35.3389337113,2.69350582125));
#53077=CARTESIAN_POINT('Ctrl Pts',(7.60913119693,-35.4355529064,2.66745188002));
#53078=CARTESIAN_POINT('Ctrl Pts',(7.60718914349,-35.5338539365,2.65003275892));
#53079=CARTESIAN_POINT('Ctrl Pts',(7.59696106493,-35.6321549665,2.64143245401));
#53080=CARTESIAN_POINT('Ctrl Pts',(7.43180190579,-35.1865123729,2.62065670169));
#53081=CARTESIAN_POINT('Ctrl Pts',(7.44817986306,-35.2646063876,2.59073345827));
#53082=CARTESIAN_POINT('Ctrl Pts',(7.45830517498,-35.3457624596,2.56600593478));
#53083=CARTESIAN_POINT('Ctrl Pts',(7.46204607379,-35.4290060284,2.5468488602));
#53084=CARTESIAN_POINT('Ctrl Pts',(7.45940380717,-35.5132946093,2.53351481199));
#53085=CARTESIAN_POINT('Ctrl Pts',(7.45050807009,-35.5975831903,2.52611015512));
#53086=CARTESIAN_POINT('Ctrl Pts',(7.32065041948,-35.231204862,2.4495725015));
#53087=CARTESIAN_POINT('Ctrl Pts',(7.32870713782,-35.2926200315,2.43080253154));
#53088=CARTESIAN_POINT('Ctrl Pts',(7.33308472128,-35.3551340146,2.41429805269));
#53089=CARTESIAN_POINT('Ctrl Pts',(7.33374284515,-35.4183882264,2.40016471574));
#53090=CARTESIAN_POINT('Ctrl Pts',(7.33068095224,-35.4820120082,2.3884845177));
#53091=CARTESIAN_POINT('Ctrl Pts',(7.3239386903,-35.5456357901,2.37931366962));
#53092=CARTESIAN_POINT('Ctrl Pts',(7.23545016815,-35.2863172732,2.26690461593));
#53093=CARTESIAN_POINT('Ctrl Pts',(7.23845227406,-35.3245433701,2.25650461508));
#53094=CARTESIAN_POINT('Ctrl Pts',(7.23974688842,-35.3631516089,2.24701631825));
#53095=CARTESIAN_POINT('Ctrl Pts',(7.23932413184,-35.4020162898,2.23847392839));
#53096=CARTESIAN_POINT('Ctrl Pts',(7.23718539906,-35.4410091937,2.23090562784));
#53097=CARTESIAN_POINT('Ctrl Pts',(7.23334333153,-35.4800020975,2.22433302544));
#53098=CARTESIAN_POINT('',(7.23545016824,-35.2863172732,2.26690461571));
#53099=CARTESIAN_POINT('Origin',(6.36960344412454,-35.479838822465,2.72827074076366));
#53100=CARTESIAN_POINT('Ctrl Pts',(8.60091078277638,-35.1203221955763,2.60032835317319));
#53101=CARTESIAN_POINT('Ctrl Pts',(8.58917610193419,-35.1184452509957,2.61832222716226));
#53102=CARTESIAN_POINT('Ctrl Pts',(8.57728470874417,-35.1167058413131,2.63573050335558));
#53103=CARTESIAN_POINT('Ctrl Pts',(8.56529427331913,-35.1150637609194,2.65251831753478));
#53104=CARTESIAN_POINT('Ctrl Pts',(8.55099972592246,-35.1131061342624,2.67253211995018));
#53105=CARTESIAN_POINT('Ctrl Pts',(8.53656330828631,-35.111286670445,2.69166387430586));
#53106=CARTESIAN_POINT('Ctrl Pts',(8.52202055329917,-35.1095697609073,2.70987559519324));
#53107=CARTESIAN_POINT('Ctrl Pts',(8.50426881377531,-35.1074740004461,2.73210588964294));
#53108=CARTESIAN_POINT('Ctrl Pts',(8.486356211608,-35.1055309944711,2.75296492849583));
#53109=CARTESIAN_POINT('Ctrl Pts',(8.46829397397454,-35.1037232384762,2.77241831890468));
#53110=CARTESIAN_POINT('Ctrl Pts',(8.46261694272413,-35.1031550537648,2.77853259486088));
#53111=CARTESIAN_POINT('Ctrl Pts',(8.45692495431307,-35.1026005215558,2.78450824985457));
#53112=CARTESIAN_POINT('Ctrl Pts',(8.45121810078767,-35.1020597946337,2.79034482063747));
#53113=CARTESIAN_POINT('Ctrl Pts',(8.43432545266925,-35.1004592086746,2.80762144005914));
#53114=CARTESIAN_POINT('Ctrl Pts',(8.41733375422917,-35.0989820350092,2.82364203030634));
#53115=CARTESIAN_POINT('Ctrl Pts',(8.40032031728529,-35.0976458319203,2.83837096012391));
#53116=CARTESIAN_POINT('Ctrl Pts',(8.38795424262058,-35.0966746238558,2.84907655984819));
#53117=CARTESIAN_POINT('Ctrl Pts',(8.37557737559973,-35.0957782495222,2.85910048902354));
#53118=CARTESIAN_POINT('Ctrl Pts',(8.3632291411423,-35.0949650753447,2.86844300309122));
#53119=CARTESIAN_POINT('Ctrl Pts',(8.3539353921421,-35.0943530496559,2.87547453307028));
#53120=CARTESIAN_POINT('Ctrl Pts',(8.34465680857996,-35.093788343402,2.88212050144329));
#53121=CARTESIAN_POINT('Ctrl Pts',(8.3354083784926,-35.0932769063359,2.88837545665666));
#53122=CARTESIAN_POINT('Ctrl Pts',(8.32900129505229,-35.0929225953959,2.89270873480106));
#53123=CARTESIAN_POINT('Ctrl Pts',(8.32260855403078,-35.092593762051,2.89685478584779));
#53124=CARTESIAN_POINT('Ctrl Pts',(8.31623077045352,-35.0923064282237,2.90080259475859));
#53125=CARTESIAN_POINT('Ctrl Pts',(8.31280674181222,-35.0921521678536,2.90292204748338));
#53126=CARTESIAN_POINT('Ctrl Pts',(8.30969504858464,-35.0920187697158,2.90480270397685));
#53127=CARTESIAN_POINT('Ctrl Pts',(8.30640603496327,-35.0918832744635,2.90674804194051));
#53128=CARTESIAN_POINT('Ctrl Pts',(8.30356875138995,-35.091766388826,2.90842619718226));
#53129=CARTESIAN_POINT('Ctrl Pts',(8.30059929606858,-35.091647958914,2.91015229702004));
#53130=CARTESIAN_POINT('Ctrl Pts',(8.29716922778335,-35.0915180419732,2.91209426874943));
#53131=CARTESIAN_POINT('Ctrl Pts',(8.27979366790461,-35.090859926916,2.92193163735584));
#53132=CARTESIAN_POINT('Ctrl Pts',(8.26173356240834,-35.0904306146764,2.93082766696923));
#53133=CARTESIAN_POINT('Ctrl Pts',(8.24304079174056,-35.0902526066801,2.93858623998578));
#53134=CARTESIAN_POINT('Ctrl Pts',(8.22466218351964,-35.090077590398,2.94621441755019));
#53135=CARTESIAN_POINT('Ctrl Pts',(8.20567267299626,-35.0901458262032,2.95274233402127));
#53136=CARTESIAN_POINT('Ctrl Pts',(8.18615591579075,-35.0904679947241,2.95801774934341));
#53137=CARTESIAN_POINT('Ctrl Pts',(8.16746736263975,-35.090776491851,2.96306929958833));
#53138=CARTESIAN_POINT('Ctrl Pts',(8.14829603416996,-35.0913180639787,2.96697197928371));
#53139=CARTESIAN_POINT('Ctrl Pts',(8.12873716243942,-35.0920882419806,2.96963148379715));
#53140=CARTESIAN_POINT('Ctrl Pts',(8.11865524740541,-35.0924852418322,2.97100236545671));
#53141=CARTESIAN_POINT('Ctrl Pts',(8.10847066029314,-35.0929427332427,2.97204361753943));
#53142=CARTESIAN_POINT('Ctrl Pts',(8.0981980181784,-35.0934582459642,2.97274725844121));
#53143=CARTESIAN_POINT('Ctrl Pts',(8.08015267138847,-35.0943638168709,2.97398330306794));
#53144=CARTESIAN_POINT('Ctrl Pts',(8.06184274437113,-35.0954494821579,2.97417418802722));
#53145=CARTESIAN_POINT('Ctrl Pts',(8.04334631915808,-35.0967195517063,2.97328424046987));
#53146=CARTESIAN_POINT('Ctrl Pts',(8.02484989394504,-35.0979896212546,2.97239429291251));
#53147=CARTESIAN_POINT('Ctrl Pts',(8.00616731932893,-35.0994444577115,2.97042256570926));
#53148=CARTESIAN_POINT('Ctrl Pts',(7.98738597285875,-35.1010686618494,2.9673822556833));
#53149=CARTESIAN_POINT('Ctrl Pts',(7.97066809495794,-35.1025144179621,2.96467597837378));
#53150=CARTESIAN_POINT('Ctrl Pts',(7.95387087369368,-35.1040979718286,2.96112003542471));
#53151=CARTESIAN_POINT('Ctrl Pts',(7.93704940278452,-35.1058237688537,2.95673871879764));
#53152=CARTESIAN_POINT('Ctrl Pts',(7.93497314784849,-35.1060367820089,2.95619793789196));
#53153=CARTESIAN_POINT('Ctrl Pts',(7.93289652996833,-35.1062519371957,2.95564464311045));
#53154=CARTESIAN_POINT('Ctrl Pts',(7.93081965722235,-35.1064692208014,2.95507893330937));
#53155=CARTESIAN_POINT('Ctrl Pts',(7.92521992861369,-35.1070550675875,2.95355364902636));
#53156=CARTESIAN_POINT('Ctrl Pts',(7.91978314717724,-35.1076390206973,2.95198445505272));
#53157=CARTESIAN_POINT('Ctrl Pts',(7.91436359224073,-35.10823574807,2.95033900501678));
#53158=CARTESIAN_POINT('Ctrl Pts',(7.90716727929602,-35.1090281077686,2.94815410726553));
#53159=CARTESIAN_POINT('Ctrl Pts',(7.90000082482723,-35.109842835178,2.94583637364108));
#53160=CARTESIAN_POINT('Ctrl Pts',(7.89252934979934,-35.1107229006809,2.94326130335969));
#53161=CARTESIAN_POINT('Ctrl Pts',(7.88663293685535,-35.1114174395241,2.94122908379365));
#53162=CARTESIAN_POINT('Ctrl Pts',(7.88054664524848,-35.1121527743485,2.93903571473777));
#53163=CARTESIAN_POINT('Ctrl Pts',(7.87411160248055,-35.1129524516452,2.93659796655904));
#53164=CARTESIAN_POINT('Ctrl Pts',(7.85178409221608,-35.1157270723736,2.92813977141633));
#53165=CARTESIAN_POINT('Ctrl Pts',(7.83002035558917,-35.1185929240505,2.91859695159043));
#53166=CARTESIAN_POINT('Ctrl Pts',(7.80885347336691,-35.1215334987328,2.90819436721776));
#53167=CARTESIAN_POINT('Ctrl Pts',(7.78669331944508,-35.1246120620703,2.89730363383233));
#53168=CARTESIAN_POINT('Ctrl Pts',(7.76518706636089,-35.1277727811105,2.8854701648589));
#53169=CARTESIAN_POINT('Ctrl Pts',(7.74434798348236,-35.131009993278,2.87289903692657));
#53170=CARTESIAN_POINT('Ctrl Pts',(7.72194176304155,-35.1344906497859,2.85938253693071));
#53171=CARTESIAN_POINT('Ctrl Pts',(7.70030659658197,-35.13805998044,2.84501305436895));
#53172=CARTESIAN_POINT('Ctrl Pts',(7.67943512205773,-35.1417219917774,2.82999016953254));
#53173=CARTESIAN_POINT('Ctrl Pts',(7.66940064330848,-35.1434825945035,2.82276754525325));
#53174=CARTESIAN_POINT('Ctrl Pts',(7.65954237285627,-35.145264752053,2.81539312665641));
#53175=CARTESIAN_POINT('Ctrl Pts',(7.64985798668585,-35.1470694734924,2.80788525165147));
#53176=CARTESIAN_POINT('Ctrl Pts',(7.62746593570419,-35.1512423156082,2.79052568782199));
#53177=CARTESIAN_POINT('Ctrl Pts',(7.605962048854,-35.1555301903078,2.77243218743555));
#53178=CARTESIAN_POINT('Ctrl Pts',(7.58531700118153,-35.1599302545228,2.75379953157052));
#53179=CARTESIAN_POINT('Ctrl Pts',(7.56258151710616,-35.1647758519502,2.73328020618935));
#53180=CARTESIAN_POINT('Ctrl Pts',(7.54088706090647,-35.1697577951558,2.71210682642349));
#53181=CARTESIAN_POINT('Ctrl Pts',(7.52017550611949,-35.1748791194298,2.69047562713645));
#53182=CARTESIAN_POINT('Ctrl Pts',(7.50387682178431,-35.1789092778886,2.67345324071511));
#53183=CARTESIAN_POINT('Ctrl Pts',(7.48818634156458,-35.1830259232671,2.65614587070935));
#53184=CARTESIAN_POINT('Ctrl Pts',(7.47307198757317,-35.1872314367054,2.63862717712488));
#53185=CARTESIAN_POINT('Ctrl Pts',(7.44966633781327,-35.1937439727128,2.61149823687892));
#53186=CARTESIAN_POINT('Ctrl Pts',(7.42764987581756,-35.2004199946401,2.5839035859179));
#53187=CARTESIAN_POINT('Ctrl Pts',(7.40692166842936,-35.2073161032801,2.55604515563927));
#53188=CARTESIAN_POINT('Ctrl Pts',(7.38524454731482,-35.2145279079194,2.52691139815117));
#53189=CARTESIAN_POINT('Ctrl Pts',(7.36497569430883,-35.2219812711745,2.49748815499357));
#53190=CARTESIAN_POINT('Ctrl Pts',(7.34600061535571,-35.2297053851017,2.46796359042044));
#53191=CARTESIAN_POINT('Ctrl Pts',(7.32695265854947,-35.2374591651421,2.43832563043612));
#53192=CARTESIAN_POINT('Ctrl Pts',(7.30920790752505,-35.2454861433858,2.40858460195775));
#53193=CARTESIAN_POINT('Ctrl Pts',(7.29266038923334,-35.2537717794306,2.37890422579583));
#53194=CARTESIAN_POINT('Ctrl Pts',(7.27609198391715,-35.2620678739792,2.34918638572348));
#53195=CARTESIAN_POINT('Ctrl Pts',(7.26072345811695,-35.2706233461039,2.31952874737719));
#53196=CARTESIAN_POINT('Ctrl Pts',(7.24646506941255,-35.2793763104888,2.29008084435969));
#53197=CARTESIAN_POINT('Ctrl Pts',(7.24271708980018,-35.281677126713,2.28234012818025));
#53198=CARTESIAN_POINT('Ctrl Pts',(7.23904592126134,-35.2839913349288,2.2746138487812));
#53199=CARTESIAN_POINT('Ctrl Pts',(7.23545016815,-35.2863172732,2.26690461593));
#53200=CARTESIAN_POINT('Ctrl Pts',(7.23545146011,-35.2863120169,2.26690923839));
#53201=CARTESIAN_POINT('Ctrl Pts',(7.2384543,-35.3245396537,2.25650943661));
#53202=CARTESIAN_POINT('Ctrl Pts',(7.23974953205,-35.3631494767,2.24702142178));
#53203=CARTESIAN_POINT('Ctrl Pts',(7.23932727374,-35.4020157716,2.23847939875));
#53204=CARTESIAN_POINT('Ctrl Pts',(7.23718891826,-35.4410103045,2.23091155076));
#53205=CARTESIAN_POINT('Ctrl Pts',(7.23334710717,-35.4800048374,2.2243394865));
#53206=CARTESIAN_POINT('Ctrl Pts',(7.23162479878,-35.288610995,2.25877896783));
#53207=CARTESIAN_POINT('Ctrl Pts',(7.23442685161,-35.3258445567,2.2487681051));
#53208=CARTESIAN_POINT('Ctrl Pts',(7.23560643854,-35.3634294381,2.2396106895));
#53209=CARTESIAN_POINT('Ctrl Pts',(7.2351548746,-35.4012499853,2.23133779585));
#53210=CARTESIAN_POINT('Ctrl Pts',(7.2330735745,-35.4391883682,2.22397519179));
#53211=CARTESIAN_POINT('Ctrl Pts',(7.22937402512,-35.477126751,2.21754286118));
#53212=CARTESIAN_POINT('Ctrl Pts',(7.22786970762,-35.291024056,2.2506285999));
#53213=CARTESIAN_POINT('Ctrl Pts',(7.23046153941,-35.32723074,2.24098939513));
#53214=CARTESIAN_POINT('Ctrl Pts',(7.23151609908,-35.3637591309,2.23214656382));
#53215=CARTESIAN_POINT('Ctrl Pts',(7.23102584019,-35.4005032431,2.22412829997));
#53216=CARTESIAN_POINT('Ctrl Pts',(7.22899220964,-35.437355218,2.21695813089));
#53217=CARTESIAN_POINT('Ctrl Pts',(7.22542564343,-35.4742071929,2.21065452768));
#53218=CARTESIAN_POINT('Ctrl Pts',(7.22418450574,-35.2935251725,2.24246594859));
#53219=CARTESIAN_POINT('Ctrl Pts',(7.22656046023,-35.328675405,2.23318153594));
#53220=CARTESIAN_POINT('Ctrl Pts',(7.22748386956,-35.3641192075,2.22463810729));
#53221=CARTESIAN_POINT('Ctrl Pts',(7.22694822371,-35.3997598036,2.21686121842));
#53222=CARTESIAN_POINT('Ctrl Pts',(7.22495501199,-35.4354987894,2.20987233634));
#53223=CARTESIAN_POINT('Ctrl Pts',(7.22151371785,-35.4712377752,2.20368850558));
#53224=CARTESIAN_POINT('Ctrl Pts',(7.22057030307,-35.2960900286,2.23430349206));
#53225=CARTESIAN_POINT('Ctrl Pts',(7.22272782881,-35.3301573964,2.22535702652));
#53226=CARTESIAN_POINT('Ctrl Pts',(7.22351653394,-35.364491827,2.21709818648));
#53227=CARTESIAN_POINT('Ctrl Pts',(7.22293085753,-35.3990052196,2.20955010655));
#53228=CARTESIAN_POINT('Ctrl Pts',(7.22097232999,-35.4336080936,2.20273236154));
#53229=CARTESIAN_POINT('Ctrl Pts',(7.21764954964,-35.4682109676,2.19666066586));
#53230=CARTESIAN_POINT('Ctrl Pts',(7.21702826363,-35.2986939836,2.22615331206));
#53231=CARTESIAN_POINT('Ctrl Pts',(7.21896725362,-35.3316545144,2.21752775213));
#53232=CARTESIAN_POINT('Ctrl Pts',(7.21961969567,-35.3648573041,2.20953871906));
#53233=CARTESIAN_POINT('Ctrl Pts',(7.21898088241,-35.3982223851,2.20220714146));
#53234=CARTESIAN_POINT('Ctrl Pts',(7.21705236747,-35.4316686126,2.19555084997));
#53235=CARTESIAN_POINT('Ctrl Pts',(7.2138419429,-35.46511484,2.18958431883));
#53236=CARTESIAN_POINT('',(7.21702820316688,-35.2986940627524,2.2261532291923));
#53237=CARTESIAN_POINT('Origin',(6.33322480789846,-35.4651139210737,2.66341322968104));
#53238=CARTESIAN_POINT('Ctrl Pts',(7.23545016822504,-35.2863172732034,2.26690461571799));
#53239=CARTESIAN_POINT('Ctrl Pts',(7.22907209381996,-35.2901447245619,2.25335534879862));
#53240=CARTESIAN_POINT('Ctrl Pts',(7.22293091414826,-35.2943546089202,2.23973522296192));
#53241=CARTESIAN_POINT('Ctrl Pts',(7.21702826419444,-35.298693983185,2.22615331335877));
#53242=CARTESIAN_POINT('Ctrl Pts',(7.07911993306,-35.3742356128,1.41233341424));
#53243=CARTESIAN_POINT('Ctrl Pts',(7.50890612221,-32.4742356128,3.82595376918));
#53244=CARTESIAN_POINT('Ctrl Pts',(7.09439816601,-35.3742356128,1.56936058085));
#53245=CARTESIAN_POINT('Ctrl Pts',(7.59518497882,-32.4742356128,4.00539873882));
#53246=CARTESIAN_POINT('Ctrl Pts',(7.10532841684,-35.3742356128,1.72680313633));
#53247=CARTESIAN_POINT('Ctrl Pts',(7.6797307274,-32.4742356128,4.18568800425));
#53248=CARTESIAN_POINT('Ctrl Pts',(7.08904842402,-35.3742356128,1.89842406838));
#53249=CARTESIAN_POINT('Ctrl Pts',(7.76642508589,-32.4742356128,4.37540694872));
#53250=CARTESIAN_POINT('Ctrl Pts',(7.1390862001,-35.3742356128,2.05065495714));
#53251=CARTESIAN_POINT('Ctrl Pts',(7.84739395748,-32.4742356128,4.5573230698));
#53252=CARTESIAN_POINT('Ctrl Pts',(7.21384189758,-35.3742356128,2.18958432614));
#53253=CARTESIAN_POINT('Ctrl Pts',(7.92659403983,-32.4742356128,4.74000601033));
#53254=CARTESIAN_POINT('Ctrl Pts',(7.21702817531,-35.2986941477,2.22615317529));
#53255=CARTESIAN_POINT('Ctrl Pts',(7.20692741189441,-35.3061131910589,2.20294516691052));
#53256=CARTESIAN_POINT('Ctrl Pts',(7.19719329525834,-35.3141912841077,2.17900438661006));
#53257=CARTESIAN_POINT('Ctrl Pts',(7.18796980246911,-35.3226070668248,2.15465538142052));
#53258=CARTESIAN_POINT('Ctrl Pts',(7.18234237094649,-35.3277416987947,2.1397995819442));
#53259=CARTESIAN_POINT('Ctrl Pts',(7.17690465211826,-35.3330009806929,2.12479257546628));
#53260=CARTESIAN_POINT('Ctrl Pts',(7.17168536591732,-35.3383049690758,2.10971258769397));
#53261=CARTESIAN_POINT('Ctrl Pts',(7.16774304131616,-35.342311272444,2.0983221016215));
#53262=CARTESIAN_POINT('Ctrl Pts',(7.16392050826559,-35.3463755747386,2.08687105022291));
#53263=CARTESIAN_POINT('Ctrl Pts',(7.160224977354,-35.3504229454298,2.07538760256753));
#53264=CARTESIAN_POINT('Ctrl Pts',(7.15647459950107,-35.3545303848657,2.06373372419597));
#53265=CARTESIAN_POINT('Ctrl Pts',(7.15285530677851,-35.3586203097449,2.05204630782424));
#53266=CARTESIAN_POINT('Ctrl Pts',(7.14937553131797,-35.3626673165653,2.0403417618537));
#53267=CARTESIAN_POINT('Ctrl Pts',(7.14731388684394,-35.3650650256538,2.0334072303603));
#53268=CARTESIAN_POINT('Ctrl Pts',(7.14530121097212,-35.3674486946293,2.02646644336296));
#53269=CARTESIAN_POINT('Ctrl Pts',(7.14333877168014,-35.3698214557652,2.01952124225387));
#53270=CARTESIAN_POINT('Ctrl Pts',(7.14233333890139,-35.3710371121333,2.01596294983756));
#53271=CARTESIAN_POINT('Ctrl Pts',(7.14133929086511,-35.3722572507634,2.01239698022069));
#53272=CARTESIAN_POINT('Ctrl Pts',(7.14035958693292,-35.3734664689908,2.00883384018665));
#53273=CARTESIAN_POINT('Ctrl Pts',(7.1401507215652,-35.3737242650467,2.00807420604723));
#53274=CARTESIAN_POINT('Ctrl Pts',(7.13994249884667,-35.3739817495794,2.00731466330882));
#53275=CARTESIAN_POINT('Ctrl Pts',(7.13973493084178,-35.3742390721046,2.00655525500559));
#53276=CARTESIAN_POINT('',(7.50890612221,-32.4742356128,3.82595376918));
#53277=CARTESIAN_POINT('',(7.07911993306,-35.3742356128,1.41233341424));
#53278=CARTESIAN_POINT('',(7.92659403983,-32.4742356128,4.74000601033));
#53279=CARTESIAN_POINT('Ctrl Pts',(7.92659403983,-32.4742356128,4.74000601033));
#53280=CARTESIAN_POINT('Ctrl Pts',(7.85943746120676,-32.4742356128,4.5851026201465));
#53281=CARTESIAN_POINT('Ctrl Pts',(7.79122837465513,-32.4742356128,4.43204332025208));
#53282=CARTESIAN_POINT('Ctrl Pts',(7.65314300948379,-32.4742356128,4.12986259549018));
#53283=CARTESIAN_POINT('Ctrl Pts',(7.58206613679357,-32.4742356128,3.97811383610292));
#53284=CARTESIAN_POINT('Ctrl Pts',(7.50890612221,-32.4742356128,3.82595376918));
#53285=CARTESIAN_POINT('',(7.23545016824,-35.2863172732,2.26690461571));
#53286=CARTESIAN_POINT('Ctrl Pts',(7.21702817531,-35.2986941477,2.22615317529));
#53287=CARTESIAN_POINT('Ctrl Pts',(7.21896716995,-35.3316547085,2.21752764579));
#53288=CARTESIAN_POINT('Ctrl Pts',(7.21961961863,-35.364857528,2.20953864245));
#53289=CARTESIAN_POINT('Ctrl Pts',(7.218980814,-35.3982226387,2.20220709377));
#53290=CARTESIAN_POINT('Ctrl Pts',(7.21705230964,-35.4316688958,2.19555083028));
#53291=CARTESIAN_POINT('Ctrl Pts',(7.21384189758,-35.4651151528,2.18958432614));
#53292=CARTESIAN_POINT('Ctrl Pts',(7.18673962782,-35.3208994409,2.15657660598));
#53293=CARTESIAN_POINT('Ctrl Pts',(7.18679863605,-35.3444227249,2.15079574742));
#53294=CARTESIAN_POINT('Ctrl Pts',(7.18629633971,-35.3679639778,2.14519357364));
#53295=CARTESIAN_POINT('Ctrl Pts',(7.18523498451,-35.3915169062,2.13977082956));
#53296=CARTESIAN_POINT('Ctrl Pts',(7.18361579364,-35.4150756718,2.13452906411));
#53297=CARTESIAN_POINT('Ctrl Pts',(7.18143896677,-35.4386344375,2.12947072768));
#53298=CARTESIAN_POINT('Ctrl Pts',(7.16019775778,-35.3488473737,2.08142068745));
#53299=CARTESIAN_POINT('Ctrl Pts',(7.15961328066171,-35.3598678430844,2.07926829342153));
#53300=CARTESIAN_POINT('Ctrl Pts',(7.15902631490073,-35.370880846883,2.07710680880288));
#53301=CARTESIAN_POINT('Ctrl Pts',(7.15843669056073,-35.3818889651522,2.07493560863704));
#53302=CARTESIAN_POINT('Ctrl Pts',(7.15784419952897,-35.3928946462221,2.07275392853839));
#53303=CARTESIAN_POINT('Ctrl Pts',(7.15724858875,-35.4039003382,2.07056083977));
#53304=CARTESIAN_POINT('Ctrl Pts',(7.13973478936,-35.3742392475,2.00655473738));
#53305=CARTESIAN_POINT('Ctrl Pts',(7.13973478936,-35.3742392475,2.00655473738));
#53306=CARTESIAN_POINT('Ctrl Pts',(7.13973478936,-35.3742392475,2.00655473738));
#53307=CARTESIAN_POINT('Ctrl Pts',(7.13973478936,-35.3742392475,2.00655473738));
#53308=CARTESIAN_POINT('Ctrl Pts',(7.13973478936,-35.3742392475,2.00655473738));
#53309=CARTESIAN_POINT('Ctrl Pts',(7.13973478936,-35.3742392475,2.00655473738));
#53310=CARTESIAN_POINT('Ctrl Pts',(3.67755458085804,-35.3742402223328,-3.05915165400695));
#53311=CARTESIAN_POINT('Ctrl Pts',(3.32386409198,-32.4742356128,-2.36922853848));
#53312=CARTESIAN_POINT('Ctrl Pts',(4.22884588785004,-35.3742402223328,-2.83736811841901));
#53313=CARTESIAN_POINT('Ctrl Pts',(3.82968047509,-32.4742356128,-1.81532491987));
#53314=CARTESIAN_POINT('Ctrl Pts',(4.75872544102183,-35.3742402223328,-2.56236102730882));
#53315=CARTESIAN_POINT('Ctrl Pts',(4.31529317605,-32.4742356128,-1.24297128633));
#53316=CARTESIAN_POINT('Ctrl Pts',(5.25779635164618,-35.3742402223328,-2.22278760948228));
#53317=CARTESIAN_POINT('Ctrl Pts',(4.78073424536,-32.4742356128,-0.651925339842));
#53318=CARTESIAN_POINT('Ctrl Pts',(6.13376882180498,-35.3742402223328,-1.39617398295829));
#53319=CARTESIAN_POINT('Ctrl Pts',(5.66596200411,-32.4742356128,0.560784091783));
#53320=CARTESIAN_POINT('Ctrl Pts',(6.70708269922301,-35.3742402223328,-0.336673954678897));
#53321=CARTESIAN_POINT('Ctrl Pts',(6.46037298138,-32.4742356128,1.83459706183));
#53322=CARTESIAN_POINT('Ctrl Pts',(6.9022352637703,-35.3742402223328,0.234415037002724));
#53323=CARTESIAN_POINT('Ctrl Pts',(6.83383584614,-32.4742356128,2.48513748583));
#53324=CARTESIAN_POINT('Ctrl Pts',(7.02153268112224,-35.3742402223328,0.820426030514367));
#53325=CARTESIAN_POINT('Ctrl Pts',(7.18368375786,-32.4742356128,3.149547989));
#53326=CARTESIAN_POINT('Ctrl Pts',(7.07911924991741,-35.3742402223328,1.41232957780478));
#53327=CARTESIAN_POINT('Ctrl Pts',(7.50890612221,-32.4742356128,3.82595376918));
#53328=CARTESIAN_POINT('',(3.68960640636,-35.2436867043,-3.0159715009));
#53329=CARTESIAN_POINT('Ctrl Pts',(7.05021190275,-35.3742261151,1.16209541223));
#53330=CARTESIAN_POINT('Ctrl Pts',(7.04171869097663,-35.3624916648819,1.09881053133014));
#53331=CARTESIAN_POINT('Ctrl Pts',(7.03181610669979,-35.3514001191425,1.03686583093715));
#53332=CARTESIAN_POINT('Ctrl Pts',(7.0207453922348,-35.3409464539044,0.976289133858449));
#53333=CARTESIAN_POINT('Ctrl Pts',(7.01066574355577,-35.3314286153456,0.921135347115895));
#53334=CARTESIAN_POINT('Ctrl Pts',(6.99961668359083,-35.3224388134776,0.867117344000881));
#53335=CARTESIAN_POINT('Ctrl Pts',(6.98777529211479,-35.313982662876,0.814283056917023));
#53336=CARTESIAN_POINT('Ctrl Pts',(6.97535175743496,-35.3051107933437,0.758851345264047));
#53337=CARTESIAN_POINT('Ctrl Pts',(6.96205390136742,-35.296823127841,0.704712867921782));
#53338=CARTESIAN_POINT('Ctrl Pts',(6.94807400250197,-35.2891198857226,0.651894013352573));
#53339=CARTESIAN_POINT('Ctrl Pts',(6.94099303581381,-35.2852181120863,0.625140704669078));
#53340=CARTESIAN_POINT('Ctrl Pts',(6.9338550959053,-35.2815270633348,0.599156040997984));
#53341=CARTESIAN_POINT('Ctrl Pts',(6.92651065807691,-35.2779519219061,0.573287683597755));
#53342=CARTESIAN_POINT('Ctrl Pts',(6.91935502796454,-35.2744686887082,0.548084339040236));
#53343=CARTESIAN_POINT('Ctrl Pts',(6.91200294794405,-35.2710955431516,0.522991274887046));
#53344=CARTESIAN_POINT('Ctrl Pts',(6.90427337831988,-35.2677637793526,0.497412802476387));
#53345=CARTESIAN_POINT('Ctrl Pts',(6.88496491533278,-35.2594410342163,0.433517784794682));
#53346=CARTESIAN_POINT('Ctrl Pts',(6.86393740024656,-35.2516146076784,0.368816956298559));
#53347=CARTESIAN_POINT('Ctrl Pts',(6.84113206475727,-35.2442990466695,0.30341006480746));
#53348=CARTESIAN_POINT('Ctrl Pts',(6.8269378687566,-35.2397457917145,0.262700370444246));
#53349=CARTESIAN_POINT('Ctrl Pts',(6.81205496222768,-35.2353893754627,0.221717668954711));
#53350=CARTESIAN_POINT('Ctrl Pts',(6.79646754329069,-35.2312242157789,0.180490035754024));
#53351=CARTESIAN_POINT('Ctrl Pts',(6.77615194395067,-35.2257956252171,0.126756695986382));
#53352=CARTESIAN_POINT('Ctrl Pts',(6.75464085353844,-35.2206974783671,0.0726059083119251));
#53353=CARTESIAN_POINT('Ctrl Pts',(6.73190164180915,-35.215929423835,0.018102116016296));
#53354=CARTESIAN_POINT('Ctrl Pts',(6.72053203594451,-35.213545396569,-0.00914978013151847));
#53355=CARTESIAN_POINT('Ctrl Pts',(6.70885536061968,-35.2112439023798,-0.0364899155650709));
#53356=CARTESIAN_POINT('Ctrl Pts',(6.69686742451631,-35.2090249653309,-0.0639095636244658));
#53357=CARTESIAN_POINT('Ctrl Pts',(6.69087345646463,-35.2079154968065,-0.0776193876541635));
#53358=CARTESIAN_POINT('Ctrl Pts',(6.68480166933077,-35.2068266690482,-0.0913490882232204));
#53359=CARTESIAN_POINT('Ctrl Pts',(6.67865151973405,-35.2057584963529,-0.105097545261577));
#53360=CARTESIAN_POINT('Ctrl Pts',(6.67557644493569,-35.2052244100052,-0.111971773780756));
#53361=CARTESIAN_POINT('Ctrl Pts',(6.67248177922061,-35.2046954875616,-0.118850691268574));
#53362=CARTESIAN_POINT('Ctrl Pts',(6.66936745357457,-35.2041717316032,-0.125734154730951));
#53363=CARTESIAN_POINT('Ctrl Pts',(6.66656635998883,-35.2037006538733,-0.131925294497191));
#53364=CARTESIAN_POINT('Ctrl Pts',(6.66323174472111,-35.2031491115,-0.139253712594071));
#53365=CARTESIAN_POINT('Ctrl Pts',(6.66076014103221,-35.2027456430887,-0.144660488535147));
#53366=CARTESIAN_POINT('Ctrl Pts',(6.66048375415258,-35.2027005252668,-0.145265100810923));
#53367=CARTESIAN_POINT('Ctrl Pts',(6.66021820472302,-35.202657240603,-0.145845705952771));
#53368=CARTESIAN_POINT('Ctrl Pts',(6.65996547595427,-35.2026160964162,-0.146398041643693));
#53369=CARTESIAN_POINT('Ctrl Pts',(6.65530185568993,-35.201856860086,-0.156590327760148));
#53370=CARTESIAN_POINT('Ctrl Pts',(6.65058095734713,-35.201106489467,-0.166823005033949));
#53371=CARTESIAN_POINT('Ctrl Pts',(6.64580190445704,-35.2003651216435,-0.177095363302161));
#53372=CARTESIAN_POINT('Ctrl Pts',(6.61069329351012,-35.1949187716898,-0.252559736314997));
#53373=CARTESIAN_POINT('Ctrl Pts',(6.57244820855811,-35.1899609730455,-0.330168424696878));
#53374=CARTESIAN_POINT('Ctrl Pts',(6.53073543904713,-35.1855053802243,-0.409584960026447));
#53375=CARTESIAN_POINT('Ctrl Pts',(6.48776104603538,-35.1809150257778,-0.491403488043048));
#53376=CARTESIAN_POINT('Ctrl Pts',(6.44110689190624,-35.1768571692308,-0.57514009064432));
#53377=CARTESIAN_POINT('Ctrl Pts',(6.39037514193269,-35.1733163496887,-0.660398503439087));
#53378=CARTESIAN_POINT('Ctrl Pts',(6.38148185565513,-35.1726956432897,-0.67534432086013));
#53379=CARTESIAN_POINT('Ctrl Pts',(6.37246316017652,-35.1720907665111,-0.690336853378118));
#53380=CARTESIAN_POINT('Ctrl Pts',(6.36331677581195,-35.1715015691976,-0.705373909880942));
#53381=CARTESIAN_POINT('Ctrl Pts',(6.30388704247073,-35.1676731887326,-0.803078994489163));
#53382=CARTESIAN_POINT('Ctrl Pts',(6.23908435969954,-35.1645227437922,-0.902647167291049));
#53383=CARTESIAN_POINT('Ctrl Pts',(6.16840308024187,-35.1620509040348,-1.00331561529873));
#53384=CARTESIAN_POINT('Ctrl Pts',(6.13306244051303,-35.160814984156,-1.05364983930258));
#53385=CARTESIAN_POINT('Ctrl Pts',(6.09625340225616,-35.1597487257998,-1.10425697375371));
#53386=CARTESIAN_POINT('Ctrl Pts',(6.05792492906513,-35.1588540447982,-1.15502954954102));
#53387=CARTESIAN_POINT('Ctrl Pts',(6.03876069246962,-35.1584067042974,-1.18041583743468));
#53388=CARTESIAN_POINT('Ctrl Pts',(6.01921696940969,-35.1580026386106,-1.20584339585966));
#53389=CARTESIAN_POINT('Ctrl Pts',(5.99928741736408,-35.1576402865646,-1.23129781727104));
#53390=CARTESIAN_POINT('Ctrl Pts',(5.9930558832247,-35.1575269870213,-1.2392568569755));
#53391=CARTESIAN_POINT('Ctrl Pts',(5.98678662972843,-35.1574177663938,-1.24721852373888));
#53392=CARTESIAN_POINT('Ctrl Pts',(5.98047948632145,-35.1573126270196,-1.25518239795847));
#53393=CARTESIAN_POINT('Ctrl Pts',(5.97709234955469,-35.1572561638291,-1.25945925190557));
#53394=CARTESIAN_POINT('Ctrl Pts',(5.97369428525231,-35.1572008777147,-1.26373674254876));
#53395=CARTESIAN_POINT('Ctrl Pts',(5.97028526725492,-35.1571467692569,-1.26801480530466));
#53396=CARTESIAN_POINT('Ctrl Pts',(5.9693721506115,-35.1571322761291,-1.26916069843488));
#53397=CARTESIAN_POINT('Ctrl Pts',(5.96845945509689,-35.1571178857888,-1.2703051263329));
#53398=CARTESIAN_POINT('Ctrl Pts',(5.96753501358586,-35.1571034095411,-1.27146331299833));
#53399=CARTESIAN_POINT('Ctrl Pts',(5.96178354348352,-35.15701334467,-1.27866904305232));
#53400=CARTESIAN_POINT('Ctrl Pts',(5.95569562279192,-35.156922109887,-1.28625626414113));
#53401=CARTESIAN_POINT('Ctrl Pts',(5.94987658651169,-35.1568387908094,-1.29347002265334));
#53402=CARTESIAN_POINT('Ctrl Pts',(5.94714891325534,-35.1567997349917,-1.29685147195594));
#53403=CARTESIAN_POINT('Ctrl Pts',(5.94448055637157,-35.1567623743348,-1.30015103597856));
#53404=CARTESIAN_POINT('Ctrl Pts',(5.94193503261732,-35.1567274276868,-1.30329182385335));
#53405=CARTESIAN_POINT('Ctrl Pts',(5.94114899344845,-35.1567166364169,-1.30426167624093));
#53406=CARTESIAN_POINT('Ctrl Pts',(5.94037467162046,-35.1567060744422,-1.30521639244965));
#53407=CARTESIAN_POINT('Ctrl Pts',(5.93961394956819,-35.1566957606942,-1.30615371755976));
#53408=CARTESIAN_POINT('Ctrl Pts',(5.93911292116412,-35.1566889678311,-1.30677106065191));
#53409=CARTESIAN_POINT('Ctrl Pts',(5.93861924218642,-35.1566823021108,-1.30737907499651));
#53410=CARTESIAN_POINT('Ctrl Pts',(5.93812871462457,-35.156675705061,-1.30798294841254));
#53411=CARTESIAN_POINT('Ctrl Pts',(5.87593085307289,-35.1558392130501,-1.38455282551269));
#53412=CARTESIAN_POINT('Ctrl Pts',(5.8117184053166,-35.1553981914991,-1.45937109845001));
#53413=CARTESIAN_POINT('Ctrl Pts',(5.74566148136113,-35.1553170792143,-1.53233725834745));
#53414=CARTESIAN_POINT('Ctrl Pts',(5.73362228837958,-35.1553022961092,-1.54563569290247));
#53415=CARTESIAN_POINT('Ctrl Pts',(5.72152191691934,-35.1552995512701,-1.55887267409941));
#53416=CARTESIAN_POINT('Ctrl Pts',(5.70936152340078,-35.1553087395002,-1.57204767529075));
#53417=CARTESIAN_POINT('Ctrl Pts',(5.64244874495201,-35.1553592978972,-1.64454335024017));
#53418=CARTESIAN_POINT('Ctrl Pts',(5.57371424926814,-35.1557687251983,-1.71516187978632));
#53419=CARTESIAN_POINT('Ctrl Pts',(5.50335441612892,-35.1565210085082,-1.78383223993651));
#53420=CARTESIAN_POINT('Ctrl Pts',(5.42259868323553,-35.1573844441835,-1.86264887457815));
#53421=CARTESIAN_POINT('Ctrl Pts',(5.33970816688366,-35.1586996156632,-1.9388943604782));
#53422=CARTESIAN_POINT('Ctrl Pts',(5.25498407598778,-35.1604819759236,-2.01253312819369));
#53423=CARTESIAN_POINT('Ctrl Pts',(5.23950411866333,-35.1608076313597,-2.02598768367616));
#53424=CARTESIAN_POINT('Ctrl Pts',(5.22396310231098,-35.1611489673329,-2.03935522430689));
#53425=CARTESIAN_POINT('Ctrl Pts',(5.20836307072808,-35.1615061778703,-2.05263552943471));
#53426=CARTESIAN_POINT('Ctrl Pts',(5.16450464390509,-35.1625104509792,-2.08997220324466));
#53427=CARTESIAN_POINT('Ctrl Pts',(5.1201784455238,-35.1636401475021,-2.12662037226471));
#53428=CARTESIAN_POINT('Ctrl Pts',(5.07542573898653,-35.1649015036721,-2.16258044277949));
#53429=CARTESIAN_POINT('Ctrl Pts',(5.0530493857179,-35.165532181757,-2.18056047803688));
#53430=CARTESIAN_POINT('Ctrl Pts',(5.03056805256408,-35.1662020708006,-2.19837117024708));
#53431=CARTESIAN_POINT('Ctrl Pts',(5.00798440517391,-35.1669035211473,-2.21600920760725));
#53432=CARTESIAN_POINT('Ctrl Pts',(4.99669258147882,-35.1672542463207,-2.22482822628733));
#53433=CARTESIAN_POINT('Ctrl Pts',(4.9853751902225,-35.1676128672095,-2.23360408292936));
#53434=CARTESIAN_POINT('Ctrl Pts',(4.97403283155191,-35.1679793842306,-2.24233677376295));
#53435=CARTESIAN_POINT('Ctrl Pts',(4.96545811282785,-35.168256467724,-2.24893860762987));
#53436=CARTESIAN_POINT('Ctrl Pts',(4.95768844276382,-35.1685110573609,-2.25489001680632));
#53437=CARTESIAN_POINT('Ctrl Pts',(4.94886665918735,-35.1688042254875,-2.26161082038719));
#53438=CARTESIAN_POINT('Ctrl Pts',(4.94601927475276,-35.168898850611,-2.26378007690297));
#53439=CARTESIAN_POINT('Ctrl Pts',(4.94306199125833,-35.1689975616605,-2.26602925228609));
#53440=CARTESIAN_POINT('Ctrl Pts',(4.93993145158124,-35.1691026237342,-2.26840534922387));
#53441=CARTESIAN_POINT('Ctrl Pts',(4.84275788847932,-35.1723638045837,-2.34216062132897));
#53442=CARTESIAN_POINT('Ctrl Pts',(4.74472048608218,-35.1762164066117,-2.4121183656713));
#53443=CARTESIAN_POINT('Ctrl Pts',(4.64620631975456,-35.1806916453217,-2.47851432158574));
#53444=CARTESIAN_POINT('Ctrl Pts',(4.54898668486911,-35.1851080768831,-2.54403779737098));
#53445=CARTESIAN_POINT('Ctrl Pts',(4.45130321877941,-35.1901317337284,-2.60609180771767));
#53446=CARTESIAN_POINT('Ctrl Pts',(4.35349606022021,-35.1957786691155,-2.66486634866325));
#53447=CARTESIAN_POINT('Ctrl Pts',(4.25606761878344,-35.2014037391182,-2.72341330989639));
#53448=CARTESIAN_POINT('Ctrl Pts',(4.15851669162129,-35.2076476179274,-2.77870563852987));
#53449=CARTESIAN_POINT('Ctrl Pts',(4.06114220912171,-35.2145035862827,-2.83090328273477));
#53450=CARTESIAN_POINT('Ctrl Pts',(3.96303037677852,-35.2214114701611,-2.88349618372362));
#53451=CARTESIAN_POINT('Ctrl Pts',(3.86509781141783,-35.2289408247001,-2.93294695745577));
#53452=CARTESIAN_POINT('Ctrl Pts',(3.76760937528583,-35.2370586591497,-2.97939765302607));
#53453=CARTESIAN_POINT('Ctrl Pts',(3.74157542818244,-35.2392264985473,-2.99180214938864));
#53454=CARTESIAN_POINT('Ctrl Pts',(3.71557292416585,-35.2414361600975,-3.00399259842331));
#53455=CARTESIAN_POINT('Ctrl Pts',(3.68960640636835,-35.2436867042943,-3.01597150091916));
#53456=CARTESIAN_POINT('',(3.66207294829051,-35.2473021020985,-3.02895254909592));
#53457=CARTESIAN_POINT('Origin',(3.70338411396943,-35.4162358614354,-3.04861059388952));
#53458=CARTESIAN_POINT('',(3.32386409198,-32.4742356128,-2.36922853848));
#53459=CARTESIAN_POINT('',(3.66207294829,-35.2473021021,-3.02895254909));
#53460=CARTESIAN_POINT('Ctrl Pts',(7.50890612221,-32.4742356128,3.82595376918));
#53461=CARTESIAN_POINT('Ctrl Pts',(6.96684511245223,-32.4742356128,2.69856143580474));
#53462=CARTESIAN_POINT('Ctrl Pts',(6.3432119791806,-32.4742356128,1.61223864180823));
#53463=CARTESIAN_POINT('Ctrl Pts',(4.94263675758286,-32.4742356128,-0.46110591833064));
#53464=CARTESIAN_POINT('Ctrl Pts',(4.16753771932367,-32.4742356128,-1.44534807371885));
#53465=CARTESIAN_POINT('Ctrl Pts',(3.32386409198,-32.4742356128,-2.36922853848));
#53466=CARTESIAN_POINT('Ctrl Pts',(7.05021190275,-35.3742261151,1.16209541223));
#53467=CARTESIAN_POINT('Ctrl Pts',(7.05021190275,-35.3742261151,1.16209541223));
#53468=CARTESIAN_POINT('Ctrl Pts',(7.05021190275,-35.3742261151,1.16209541223));
#53469=CARTESIAN_POINT('Ctrl Pts',(7.05021190275,-35.3742261151,1.16209541223));
#53470=CARTESIAN_POINT('Ctrl Pts',(7.05021190275,-35.3742261151,1.16209541223));
#53471=CARTESIAN_POINT('Ctrl Pts',(7.05021190275,-35.3742261151,1.16209541223));
#53472=CARTESIAN_POINT('Ctrl Pts',(7.01340171355,-35.3233663073,0.887814197822));
#53473=CARTESIAN_POINT('Ctrl Pts',(7.01381986471783,-35.3413180972,0.890929938671949));
#53474=CARTESIAN_POINT('Ctrl Pts',(7.01423801594781,-35.3592698878,0.894045679984952));
#53475=CARTESIAN_POINT('Ctrl Pts',(7.01465616709811,-35.377221677,0.897161420704254));
#53476=CARTESIAN_POINT('Ctrl Pts',(7.01507431822199,-35.3951734669,0.900277161226733));
#53477=CARTESIAN_POINT('Ctrl Pts',(7.01549246939,-35.4131252568,0.903392902078));
#53478=CARTESIAN_POINT('Ctrl Pts',(6.95185482919,-35.2775995372,0.614848488511));
#53479=CARTESIAN_POINT('Ctrl Pts',(6.95711039026,-35.3122184667,0.620033495106));
#53480=CARTESIAN_POINT('Ctrl Pts',(6.96131634916,-35.3468297586,0.625353240693));
#53481=CARTESIAN_POINT('Ctrl Pts',(6.96447793891,-35.3814361808,0.630808421027));
#53482=CARTESIAN_POINT('Ctrl Pts',(6.96659784091,-35.4160401708,0.636399696014));
#53483=CARTESIAN_POINT('Ctrl Pts',(6.96767646618,-35.4506441608,0.642127552041));
#53484=CARTESIAN_POINT('Ctrl Pts',(6.8673530143,-35.2439788226,0.343363482131));
#53485=CARTESIAN_POINT('Ctrl Pts',(6.87994051011,-35.2916209137,0.34796525773));
#53486=CARTESIAN_POINT('Ctrl Pts',(6.88986767191,-35.3397700495,0.353240035009));
#53487=CARTESIAN_POINT('Ctrl Pts',(6.89711069428,-35.38825575,0.359155938781));
#53488=CARTESIAN_POINT('Ctrl Pts',(6.90165550114,-35.4369097195,0.365681814414));
#53489=CARTESIAN_POINT('Ctrl Pts',(6.90349674466,-35.485563689,0.372787607728));
#53490=CARTESIAN_POINT('Ctrl Pts',(6.64187024435,-35.1886753155,-0.23870995558));
#53491=CARTESIAN_POINT('Ctrl Pts',(6.66955139679,-35.2585364198,-0.239842936739));
#53492=CARTESIAN_POINT('Ctrl Pts',(6.691390474,-35.3305802147,-0.238616506959));
#53493=CARTESIAN_POINT('Ctrl Pts',(6.70712809876,-35.4041022846,-0.23504887133));
#53494=CARTESIAN_POINT('Ctrl Pts',(6.71661554426,-35.4783635248,-0.229196354076));
#53495=CARTESIAN_POINT('Ctrl Pts',(6.71982081074,-35.5526247648,-0.221149174844));
#53496=CARTESIAN_POINT('Ctrl Pts',(6.335633879,-35.1655247078,-0.779903703387));
#53497=CARTESIAN_POINT('Ctrl Pts',(6.37258533768,-35.2460676029,-0.793096558606));
#53498=CARTESIAN_POINT('Ctrl Pts',(6.40175618506,-35.3308011559,-0.801727405553));
#53499=CARTESIAN_POINT('Ctrl Pts',(6.42255691503,-35.4184152395,-0.805611032625));
#53500=CARTESIAN_POINT('Ctrl Pts',(6.43465051901,-35.5074700242,-0.804704006103));
#53501=CARTESIAN_POINT('Ctrl Pts',(6.43798249823,-35.5965248091,-0.799107100072));
#53502=CARTESIAN_POINT('Ctrl Pts',(6.1477485618,-35.1585065417,-1.0593892471));
#53503=CARTESIAN_POINT('Ctrl Pts',(6.1862455007,-35.2425122041,-1.07972455995));
#53504=CARTESIAN_POINT('Ctrl Pts',(6.21657209688,-35.331564736,-1.09437680653));
#53505=CARTESIAN_POINT('Ctrl Pts',(6.23800931387,-35.4241081414,-1.10297704478));
#53506=CARTESIAN_POINT('Ctrl Pts',(6.25014939755,-35.5183977765,-1.10536973107));
#53507=CARTESIAN_POINT('Ctrl Pts',(6.25293978467,-35.6126874115,-1.1016283265));
#53508=CARTESIAN_POINT('Ctrl Pts',(5.64263928747,-35.1503549657,-1.69778761613));
#53509=CARTESIAN_POINT('Ctrl Pts',(5.6781072677,-35.2388302664,-1.73263418024));
#53510=CARTESIAN_POINT('Ctrl Pts',(5.70553308479,-35.3334375132,-1.75965360778));
#53511=CARTESIAN_POINT('Ctrl Pts',(5.72416357539,-35.4323082835,-1.77811755991));
#53512=CARTESIAN_POINT('Ctrl Pts',(5.7335949111,-35.5333121034,-1.78763419493));
#53513=CARTESIAN_POINT('Ctrl Pts',(5.73382235555,-35.6343159234,-1.78819570677));
#53514=CARTESIAN_POINT('Ctrl Pts',(5.01710815157,-35.1629277461,-2.24626629333));
#53515=CARTESIAN_POINT('Ctrl Pts',(5.03812134505,-35.2465940911,-2.28433468893));
#53516=CARTESIAN_POINT('Ctrl Pts',(5.05330548672,-35.3352292266,-2.31441076458));
#53517=CARTESIAN_POINT('Ctrl Pts',(5.06229638123,-35.4272996663,-2.33577662822));
#53518=CARTESIAN_POINT('Ctrl Pts',(5.06494250992,-35.5210885082,-2.34802021045));
#53519=CARTESIAN_POINT('Ctrl Pts',(5.06131871348,-35.6148773502,-2.35107992573));
#53520=CARTESIAN_POINT('Ctrl Pts',(4.60859161999,-35.1762367254,-2.53785301358));
#53521=CARTESIAN_POINT('Ctrl Pts',(4.61998718798,-35.2544472454,-2.57156731299));
#53522=CARTESIAN_POINT('Ctrl Pts',(4.62723219199,-35.3360986017,-2.59812098394));
#53523=CARTESIAN_POINT('Ctrl Pts',(4.63022512886,-35.4200944121,-2.61708014375));
#53524=CARTESIAN_POINT('Ctrl Pts',(4.62896118843,-35.5052625726,-2.62819842135));
#53525=CARTESIAN_POINT('Ctrl Pts',(4.62352979415,-35.5904307331,-2.63143094545));
#53526=CARTESIAN_POINT('Ctrl Pts',(4.16372827527,-35.2025940852,-2.79724907986));
#53527=CARTESIAN_POINT('Ctrl Pts',(4.16779886982,-35.2702188379,-2.82151459563));
#53528=CARTESIAN_POINT('Ctrl Pts',(4.16935260067,-35.3397404397,-2.84063625327));
#53529=CARTESIAN_POINT('Ctrl Pts',(4.16836377754,-35.4105469366,-2.8544077757));
#53530=CARTESIAN_POINT('Ctrl Pts',(4.16484831327,-35.4819959329,-2.86271080605));
#53531=CARTESIAN_POINT('Ctrl Pts',(4.15886281142,-35.5534449291,-2.86552034537));
#53532=CARTESIAN_POINT('Ctrl Pts',(3.68960640598,-35.2436867043,-3.01597150109));
#53533=CARTESIAN_POINT('Ctrl Pts',(3.68994006034,-35.2950048916,-3.03107790462));
#53534=CARTESIAN_POINT('Ctrl Pts',(3.68889543294,-35.347263528,-3.04301993645));
#53535=CARTESIAN_POINT('Ctrl Pts',(3.68647051499,-35.4001566504,-3.05170748242));
#53536=CARTESIAN_POINT('Ctrl Pts',(3.68267984997,-35.4533670311,-3.0570884388));
#53537=CARTESIAN_POINT('Ctrl Pts',(3.67755401867,-35.5065774118,-3.05915055738));
#53538=CARTESIAN_POINT('Origin',(3.30432478182257,-35.5065775309065,-2.13141045451377));
#53539=CARTESIAN_POINT('Ctrl Pts',(3.50597880735,-35.2696545374,-3.18321831335));
#53540=CARTESIAN_POINT('Ctrl Pts',(3.51333803189,-35.3113514663,-3.18868569298));
#53541=CARTESIAN_POINT('Ctrl Pts',(3.51870881162,-35.353530752,-3.19315085121));
#53542=CARTESIAN_POINT('Ctrl Pts',(3.52206318971,-35.3960340603,-3.19659302084));
#53543=CARTESIAN_POINT('Ctrl Pts',(3.52338838043,-35.4386993829,-3.1989990815));
#53544=CARTESIAN_POINT('Ctrl Pts',(3.52268705855,-35.4813647056,-3.20036385665));
#53545=CARTESIAN_POINT('Ctrl Pts',(3.50256004198,-35.268393509,-3.18939410052));
#53546=CARTESIAN_POINT('Ctrl Pts',(3.51052316476,-35.3102955518,-3.1938621313));
#53547=CARTESIAN_POINT('Ctrl Pts',(3.51648359784,-35.3526863763,-3.19731644996));
#53548=CARTESIAN_POINT('Ctrl Pts',(3.52041085984,-35.3954055593,-3.19973991273));
#53549=CARTESIAN_POINT('Ctrl Pts',(3.52228987577,-35.4382889251,-3.2011231722));
#53550=CARTESIAN_POINT('Ctrl Pts',(3.52212131885,-35.4811722908,-3.20146489487));
#53551=CARTESIAN_POINT('Ctrl Pts',(3.49913203155,-35.2673150056,-3.1956382498));
#53552=CARTESIAN_POINT('Ctrl Pts',(3.50770826391,-35.3094204104,-3.19910017162));
#53553=CARTESIAN_POINT('Ctrl Pts',(3.51426388564,-35.3520219724,-3.20153494382));
#53554=CARTESIAN_POINT('Ctrl Pts',(3.5187657727,-35.3949568785,-3.20292908338));
#53555=CARTESIAN_POINT('Ctrl Pts',(3.52119645205,-35.4380584515,-3.20327716833));
#53556=CARTESIAN_POINT('Ctrl Pts',(3.52155459752,-35.4811600245,-3.20258180379));
#53557=CARTESIAN_POINT('Ctrl Pts',(3.49570498282,-35.2664275319,-3.20193555292));
#53558=CARTESIAN_POINT('Ctrl Pts',(3.5049017062,-35.3087336513,-3.20438752525));
#53559=CARTESIAN_POINT('Ctrl Pts',(3.51205619329,-35.3515442739,-3.2057969486));
#53560=CARTESIAN_POINT('Ctrl Pts',(3.51713243885,-35.3946938503,-3.20615423225));
#53561=CARTESIAN_POINT('Ctrl Pts',(3.52011064813,-35.4380129429,-3.20545771792));
#53562=CARTESIAN_POINT('Ctrl Pts',(3.52098739307,-35.4813320354,-3.20371424309));
#53563=CARTESIAN_POINT('Ctrl Pts',(3.49229725928,-35.2657414976,-3.2082566117));
#53564=CARTESIAN_POINT('Ctrl Pts',(3.50211831443,-35.308244275,-3.20970015733));
#53565=CARTESIAN_POINT('Ctrl Pts',(3.50987186481,-35.3512608603,-3.21008384904));
#53566=CARTESIAN_POINT('Ctrl Pts',(3.51551898686,-35.3946227115,-3.20940189333));
#53567=CARTESIAN_POINT('Ctrl Pts',(3.51903723035,-35.4381571989,-3.20765694424));
#53568=CARTESIAN_POINT('Ctrl Pts',(3.52042115146,-35.4816916863,-3.20486003554));
#53569=CARTESIAN_POINT('Ctrl Pts',(3.4889030666,-35.265254082,-3.21461371656));
#53570=CARTESIAN_POINT('Ctrl Pts',(3.49935367791,-35.3079501561,-3.21504791216));
#53571=CARTESIAN_POINT('Ctrl Pts',(3.50770783634,-35.3511703481,-3.21440295273));
#53572=CARTESIAN_POINT('Ctrl Pts',(3.51392345649,-35.3947427765,-3.21267708331));
#53573=CARTESIAN_POINT('Ctrl Pts',(3.51797541562,-35.4384913269,-3.20987727967));
#53574=CARTESIAN_POINT('Ctrl Pts',(3.51985615629,-35.4822398773,-3.20601908088));
#53575=CARTESIAN_POINT('',(3.50597898435511,-35.2696545360883,-3.18321830583732));
#53576=CARTESIAN_POINT('Origin',(3.5116682051481,-35.3848727889406,-3.20631688515481));
#53577=CARTESIAN_POINT('Origin',(2.63323785737633,-35.4813643327716,-2.74332899791331));
#53578=CARTESIAN_POINT('Ctrl Pts',(3.66378622939474,-35.2464640243768,-3.0279781015246));
#53579=CARTESIAN_POINT('Ctrl Pts',(3.66837475167183,-35.2970123124896,-3.04073454824404));
#53580=CARTESIAN_POINT('Ctrl Pts',(3.67167460756035,-35.3484462252211,-3.0504452225707));
#53581=CARTESIAN_POINT('Ctrl Pts',(3.67365999774165,-35.4004772676907,-3.05703724741477));
#53582=CARTESIAN_POINT('Ctrl Pts',(3.67431938153269,-35.4528069345301,-3.06047287388992));
#53583=CARTESIAN_POINT('Ctrl Pts',(3.673656359803,-35.5051366012576,-3.06075050068259));
#53584=CARTESIAN_POINT('Ctrl Pts',(3.64685377738682,-35.2475881828974,-3.03546815079806));
#53585=CARTESIAN_POINT('Ctrl Pts',(3.65197996915299,-35.2977377775771,-3.04779720191966));
#53586=CARTESIAN_POINT('Ctrl Pts',(3.65566459258164,-35.3487504451489,-3.05720437609867));
#53587=CARTESIAN_POINT('Ctrl Pts',(3.65787487045666,-35.4003455971741,-3.06362096615626));
#53588=CARTESIAN_POINT('Ctrl Pts',(3.65859977260828,-35.4522315476326,-3.06701003015053));
#53589=CARTESIAN_POINT('Ctrl Pts',(3.65784552585749,-35.5041174980908,-3.06737014843955));
#53590=CARTESIAN_POINT('Ctrl Pts',(3.63069497520593,-35.2488274318634,-3.04411012182609));
#53591=CARTESIAN_POINT('Ctrl Pts',(3.63621005013032,-35.2985088014843,-3.05599604307844));
#53592=CARTESIAN_POINT('Ctrl Pts',(3.6401348662033,-35.3490281789965,-3.06510435036028));
#53593=CARTESIAN_POINT('Ctrl Pts',(3.64244429896267,-35.4001115250326,-3.0713693085073));
#53594=CARTESIAN_POINT('Ctrl Pts',(3.6431236689932,-35.451477515452,-3.07475727773419));
#53595=CARTESIAN_POINT('Ctrl Pts',(3.64217553898255,-35.5028435058782,-3.07526460898209));
#53596=CARTESIAN_POINT('Ctrl Pts',(3.6149475468118,-35.2501319216701,-3.05405854836525));
#53597=CARTESIAN_POINT('Ctrl Pts',(3.62087332233153,-35.2992445854584,-3.06542135460391));
#53598=CARTESIAN_POINT('Ctrl Pts',(3.6250932299558,-35.3491642058263,-3.07416948701838));
#53599=CARTESIAN_POINT('Ctrl Pts',(3.62757315136577,-35.3996287881775,-3.08023942083983));
#53600=CARTESIAN_POINT('Ctrl Pts',(3.62829959911055,-35.4503649729954,-3.08359895575808));
#53601=CARTESIAN_POINT('Ctrl Pts',(3.62728035817098,-35.5011011577074,-3.0842466362974));
#53602=CARTESIAN_POINT('Ctrl Pts',(3.57804594423897,-35.2537396575121,-3.08151411792311));
#53603=CARTESIAN_POINT('Ctrl Pts',(3.58490210551495,-35.3013209015024,-3.09141036639288));
#53604=CARTESIAN_POINT('Ctrl Pts',(3.58981192437177,-35.3496314438259,-3.09910496604094));
#53605=CARTESIAN_POINT('Ctrl Pts',(3.59274404424921,-35.3984313240945,-3.10455252216444));
#53606=CARTESIAN_POINT('Ctrl Pts',(3.59368370155741,-35.4474771670055,-3.10772506981888));
#53607=CARTESIAN_POINT('Ctrl Pts',(3.59263285291033,-35.4965230101221,-3.10861522294742));
#53608=CARTESIAN_POINT('Ctrl Pts',(3.54614995886284,-35.2585698054349,-3.11565459351817));
#53609=CARTESIAN_POINT('Ctrl Pts',(3.55365282508503,-35.3042784980418,-3.1238029213662));
#53610=CARTESIAN_POINT('Ctrl Pts',(3.55910677430424,-35.3506275899982,-3.13019982938299));
#53611=CARTESIAN_POINT('Ctrl Pts',(3.56247248748482,-35.3974100369749,-3.13480265896626));
#53612=CARTESIAN_POINT('Ctrl Pts',(3.56373415608727,-35.4444073086632,-3.13759135387308));
#53613=CARTESIAN_POINT('Ctrl Pts',(3.56290037565488,-35.4914045803479,-3.1385656230307));
#53614=CARTESIAN_POINT('Ctrl Pts',(3.5297693370109,-35.262096319147,-3.13775667457677));
#53615=CARTESIAN_POINT('Ctrl Pts',(3.53742200429963,-35.3066260775261,-3.14485178755018));
#53616=CARTESIAN_POINT('Ctrl Pts',(3.54299253665026,-35.3517487998208,-3.15044517412045));
#53617=CARTESIAN_POINT('Ctrl Pts',(3.54645603898634,-35.3972616314089,-3.15453043124095));
#53618=CARTESIAN_POINT('Ctrl Pts',(3.54780199054788,-35.4429759293891,-3.15708363433905));
#53619=CARTESIAN_POINT('Ctrl Pts',(3.54701944502996,-35.4886902276847,-3.15808466613649));
#53620=CARTESIAN_POINT('Ctrl Pts',(3.51627715008437,-35.265772097736,-3.16057033053923));
#53621=CARTESIAN_POINT('Ctrl Pts',(3.52379883042827,-35.3089013381962,-3.16688771508641));
#53622=CARTESIAN_POINT('Ctrl Pts',(3.52927202428577,-35.3525623688612,-3.17198724899732));
#53623=CARTESIAN_POINT('Ctrl Pts',(3.53266012631829,-35.3965870683247,-3.17582587319325));
#53624=CARTESIAN_POINT('Ctrl Pts',(3.53394593132937,-35.4407889521592,-3.17839253457853));
#53625=CARTESIAN_POINT('Ctrl Pts',(3.53314312461956,-35.4849908356552,-3.17969330859528));
#53626=CARTESIAN_POINT('Ctrl Pts',(3.50505237127691,-35.269315766807,-3.18490659755473));
#53627=CARTESIAN_POINT('Ctrl Pts',(3.5124462254045,-35.3110230787235,-3.19033652396823));
#53628=CARTESIAN_POINT('Ctrl Pts',(3.51784430886608,-35.35321329042,-3.19477526792434));
#53629=CARTESIAN_POINT('Ctrl Pts',(3.52121894386514,-35.395727447307,-3.19820343835999));
#53630=CARTESIAN_POINT('Ctrl Pts',(3.52255749924592,-35.4384039093696,-3.20060764124573));
#53631=CARTESIAN_POINT('Ctrl Pts',(3.5218618906809,-35.4810803715647,-3.20198185530188));
#53632=CARTESIAN_POINT('Ctrl Pts',(3.66207294829203,-35.247302102094,-3.02895254911367));
#53633=CARTESIAN_POINT('Ctrl Pts',(3.65265573864293,-35.2479321008334,-3.03318696750315));
#53634=CARTESIAN_POINT('Ctrl Pts',(3.64324606816193,-35.2486494149569,-3.03798955551632));
#53635=CARTESIAN_POINT('Ctrl Pts',(3.63389358932175,-35.2494540499443,-3.04342239580713));
#53636=CARTESIAN_POINT('Ctrl Pts',(3.62444446054903,-35.2502670001515,-3.04891137989217));
#53637=CARTESIAN_POINT('Ctrl Pts',(3.61505379466542,-35.251169085322,-3.0550438523311));
#53638=CARTESIAN_POINT('Ctrl Pts',(3.60581140686814,-35.2521603111073,-3.06184608738143));
#53639=CARTESIAN_POINT('Ctrl Pts',(3.59604940078202,-35.2532072648125,-3.06903075236379));
#53640=CARTESIAN_POINT('Ctrl Pts',(3.58645323658232,-35.2543536640781,-3.07696257748029));
#53641=CARTESIAN_POINT('Ctrl Pts',(3.577168615446,-35.2555995155633,-3.08562884702655));
#53642=CARTESIAN_POINT('Ctrl Pts',(3.56445418506134,-35.2573055940071,-3.09749650206843));
#53643=CARTESIAN_POINT('Ctrl Pts',(3.55232717675937,-35.2591981729177,-3.11074138259069));
#53644=CARTESIAN_POINT('Ctrl Pts',(3.54121912889871,-35.2612772693964,-3.12523908272482));
#53645=CARTESIAN_POINT('Ctrl Pts',(3.53419394128748,-35.2625921757604,-3.13440802623778));
#53646=CARTESIAN_POINT('Ctrl Pts',(3.52757805820054,-35.2639816857809,-3.14407554672188));
#53647=CARTESIAN_POINT('Ctrl Pts',(3.52146452079015,-35.2654458037837,-3.1542111523752));
#53648=CARTESIAN_POINT('Ctrl Pts',(3.51586767175993,-35.2667861811912,-3.16349014273109));
#53649=CARTESIAN_POINT('Ctrl Pts',(3.51069302206195,-35.2681890884407,-3.17316034952375));
#53650=CARTESIAN_POINT('Ctrl Pts',(3.50597898250972,-35.2696545288516,-3.18321830602679));
#53651=CARTESIAN_POINT('Origin',(3.28043975923886,-35.505031377995,-2.14129772753315));
#53652=CARTESIAN_POINT('Ctrl Pts',(3.68960640636,-35.2436867043,-3.0159715009));
#53653=CARTESIAN_POINT('Ctrl Pts',(3.68994006064,-35.2950048915,-3.03107790447));
#53654=CARTESIAN_POINT('Ctrl Pts',(3.68889543318,-35.347263528,-3.04301993635));
#53655=CARTESIAN_POINT('Ctrl Pts',(3.68647051515,-35.4001566503,-3.05170748236));
#53656=CARTESIAN_POINT('Ctrl Pts',(3.68267985005,-35.4533670311,-3.05708843877));
#53657=CARTESIAN_POINT('Ctrl Pts',(3.67755401867,-35.5065774118,-3.05915055738));
#53658=CARTESIAN_POINT('Ctrl Pts',(3.68406493808,-35.2441669878,-3.01852789669));
#53659=CARTESIAN_POINT('Ctrl Pts',(3.6852545996,-35.2952993243,-3.03313678947));
#53660=CARTESIAN_POINT('Ctrl Pts',(3.68508444483,-35.3473574121,-3.04461628848));
#53661=CARTESIAN_POINT('Ctrl Pts',(3.68354738519,-35.4000399811,-3.05288030368));
#53662=CARTESIAN_POINT('Ctrl Pts',(3.68065246874,-35.4530348056,-3.05787988529));
#53663=CARTESIAN_POINT('Ctrl Pts',(3.67642456268,-35.5060296301,-3.05960493674));
#53664=CARTESIAN_POINT('Ctrl Pts',(3.67853556896,-35.2447691838,-3.02110736508));
#53665=CARTESIAN_POINT('Ctrl Pts',(3.68058228399,-35.295713802,-3.03522035827));
#53666=CARTESIAN_POINT('Ctrl Pts',(3.68128649848,-35.3475703565,-3.04623632347));
#53667=CARTESIAN_POINT('Ctrl Pts',(3.68063618362,-35.4000419929,-3.05407302366));
#53668=CARTESIAN_POINT('Ctrl Pts',(3.67863507204,-35.4528211843,-3.05868456544));
#53669=CARTESIAN_POINT('Ctrl Pts',(3.67530251301,-35.5056003757,-3.0600629924));
#53670=CARTESIAN_POINT('Ctrl Pts',(3.67302394084,-35.2454929622,-3.02370658462));
#53671=CARTESIAN_POINT('Ctrl Pts',(3.6759278736,-35.2962481955,-3.03732595805));
#53672=CARTESIAN_POINT('Ctrl Pts',(3.67750544789,-35.3479024371,-3.04787800394));
#53673=CARTESIAN_POINT('Ctrl Pts',(3.67773982365,-35.4001629685,-3.05528416988));
#53674=CARTESIAN_POINT('Ctrl Pts',(3.67662956704,-35.4527266586,-3.05950153137));
#53675=CARTESIAN_POINT('Ctrl Pts',(3.67418869929,-35.5052903486,-3.06052426199));
#53676=CARTESIAN_POINT('Ctrl Pts',(3.6675348968,-35.2463373792,-3.02632251085));
#53677=CARTESIAN_POINT('Ctrl Pts',(3.67129543056,-35.2969017565,-3.03945109726));
#53678=CARTESIAN_POINT('Ctrl Pts',(3.67374456646,-35.348353094,-3.04953936585));
#53679=CARTESIAN_POINT('Ctrl Pts',(3.67486076111,-35.4004025315,-3.05651229579));
#53680=CARTESIAN_POINT('Ctrl Pts',(3.67463755638,-35.4527510324,-3.06032984675));
#53681=CARTESIAN_POINT('Ctrl Pts',(3.67308380368,-35.5050995333,-3.0609883158));
#53682=CARTESIAN_POINT('Ctrl Pts',(3.66207264655,-35.2473009405,-3.02895231242));
#53683=CARTESIAN_POINT('Ctrl Pts',(3.66668846955,-35.2976731782,-3.04159341678));
#53684=CARTESIAN_POINT('Ctrl Pts',(3.67000667781,-35.348921195,-3.05121851933));
#53685=CARTESIAN_POINT('Ctrl Pts',(3.67200111268,-35.4007597143,-3.05775598766));
#53686=CARTESIAN_POINT('Ctrl Pts',(3.67266041516,-35.4528934978,-3.0611685886));
#53687=CARTESIAN_POINT('Ctrl Pts',(3.67198840819,-35.5050272814,-3.06145474134));
#53688=CARTESIAN_POINT('Ctrl Pts',(-1.69382496103,-35.2682576589,-5.01043544546));
#53689=CARTESIAN_POINT('Ctrl Pts',(-1.69402179658,-35.3094043143,-5.02023549828));
#53690=CARTESIAN_POINT('Ctrl Pts',(-1.69321049045,-35.351018059,-5.02809467113));
#53691=CARTESIAN_POINT('Ctrl Pts',(-1.69139030338,-35.3929455262,-5.03397642476));
#53692=CARTESIAN_POINT('Ctrl Pts',(-1.68856804502,-35.4350298576,-5.03785875444));
#53693=CARTESIAN_POINT('Ctrl Pts',(-1.6847579226,-35.4771141891,-5.03973467901));
#53694=CARTESIAN_POINT('Ctrl Pts',(-1.68490151218,-35.268974041,-5.01524294734));
#53695=CARTESIAN_POINT('Ctrl Pts',(-1.68651188124,-35.3098358784,-5.02415397172));
#53696=CARTESIAN_POINT('Ctrl Pts',(-1.68714086448,-35.3511508863,-5.03116493545));
#53697=CARTESIAN_POINT('Ctrl Pts',(-1.68678246934,-35.3927702163,-5.03624343644));
#53698=CARTESIAN_POINT('Ctrl Pts',(-1.68543788474,-35.4345417096,-5.03937097175));
#53699=CARTESIAN_POINT('Ctrl Pts',(-1.68311545107,-35.4763132029,-5.04054334111));
#53700=CARTESIAN_POINT('Ctrl Pts',(-1.67612908012,-35.2701100859,-5.02003914153));
#53701=CARTESIAN_POINT('Ctrl Pts',(-1.67913856906,-35.3106802184,-5.02807779826));
#53702=CARTESIAN_POINT('Ctrl Pts',(-1.68118935788,-35.3516915586,-5.03424982493));
#53703=CARTESIAN_POINT('Ctrl Pts',(-1.6822703811,-35.3929991785,-5.03852665843));
#53704=CARTESIAN_POINT('Ctrl Pts',(-1.68237796302,-35.4344548915,-5.04089285688));
#53705=CARTESIAN_POINT('Ctrl Pts',(-1.68151488066,-35.4759106045,-5.04134696784));
#53706=CARTESIAN_POINT('Ctrl Pts',(-1.66745641736,-35.2716459733,-5.02484351574));
#53707=CARTESIAN_POINT('Ctrl Pts',(-1.67185679176,-35.3119189644,-5.03202383893));
#53708=CARTESIAN_POINT('Ctrl Pts',(-1.67531720482,-35.3526230495,-5.03736380107));
#53709=CARTESIAN_POINT('Ctrl Pts',(-1.67782194293,-35.3936164734,-5.04083824001));
#53710=CARTESIAN_POINT('Ctrl Pts',(-1.67936231019,-35.4347546994,-5.04243484007));
#53711=CARTESIAN_POINT('Ctrl Pts',(-1.67993607839,-35.4758929253,-5.04215470289));
#53712=CARTESIAN_POINT('Ctrl Pts',(-1.65900707813,-35.2735686701,-5.02958783575));
#53713=CARTESIAN_POINT('Ctrl Pts',(-1.66477502429,-35.3135351172,-5.03593051298));
#53714=CARTESIAN_POINT('Ctrl Pts',(-1.6696184323,-35.3539241381,-5.04045242297));
#53715=CARTESIAN_POINT('Ctrl Pts',(-1.67351721006,-35.3945968399,-5.04313153636));
#53716=CARTESIAN_POINT('Ctrl Pts',(-1.67645771737,-35.4354113842,-5.0439585342));
#53717=CARTESIAN_POINT('Ctrl Pts',(-1.67843305643,-35.4762259285,-5.04293699751));
#53718=CARTESIAN_POINT('Ctrl Pts',(-1.65073625045,-35.2758278019,-5.0342827697));
#53719=CARTESIAN_POINT('Ctrl Pts',(-1.65785005217,-35.3154860139,-5.03981027692));
#53720=CARTESIAN_POINT('Ctrl Pts',(-1.66405116082,-35.3555599215,-5.04352991245));
#53721=CARTESIAN_POINT('Ctrl Pts',(-1.66931505993,-35.3959128757,-5.04542262153));
#53722=CARTESIAN_POINT('Ctrl Pts',(-1.67362354949,-35.4364053554,-5.04548186008));
#53723=CARTESIAN_POINT('Ctrl Pts',(-1.67696511998,-35.4768978351,-5.04371372921));
#53724=CARTESIAN_POINT('',(-1.69382496553272,-35.2682576607491,-5.01043544611819));
#53725=CARTESIAN_POINT('Origin',(-1.24303989658678,-35.4771141385556,-4.14258040411198));
#53726=CARTESIAN_POINT('',(-1.65073615062032,-35.2758275456167,-5.03428276116393));
#53727=CARTESIAN_POINT('Ctrl Pts',(-1.69382496014738,-35.268257661,-5.01043544642385));
#53728=CARTESIAN_POINT('Ctrl Pts',(-1.68803312612198,-35.2687226336122,
-5.01355579279809));
#53729=CARTESIAN_POINT('Ctrl Pts',(-1.68231297816127,-35.2693997637279,
-5.01667279399805));
#53730=CARTESIAN_POINT('Ctrl Pts',(-1.67666523914987,-35.2702777195431,
-5.0197822570377));
#53731=CARTESIAN_POINT('Ctrl Pts',(-1.67037182346692,-35.2712560474872,
-5.02324720883873));
#53732=CARTESIAN_POINT('Ctrl Pts',(-1.66417391129964,-35.2724846442873,
-5.02670011798684));
#53733=CARTESIAN_POINT('Ctrl Pts',(-1.65809711371162,-35.2739404345783,
-5.03012131671218));
#53734=CARTESIAN_POINT('Ctrl Pts',(-1.65562402628534,-35.2745329006942,
-5.03151364933934));
#53735=CARTESIAN_POINT('Ctrl Pts',(-1.65317074085282,-35.2751628346991,
-5.03290083178419));
#53736=CARTESIAN_POINT('Ctrl Pts',(-1.65073625045,-35.2758278019,-5.0342827697));
#53737=CARTESIAN_POINT('Origin',(-1.20926787984816,-35.4768981557406,-4.15982468247784));
#53738=CARTESIAN_POINT('Ctrl Pts',(-1.65073607085,-35.2758272825,-5.03428274092));
#53739=CARTESIAN_POINT('Ctrl Pts',(-1.65784980534,-35.3154856499,-5.03981034314));
#53740=CARTESIAN_POINT('Ctrl Pts',(-1.66405083454,-35.3555597177,-5.04353006314));
#53741=CARTESIAN_POINT('Ctrl Pts',(-1.66931464207,-35.3959128353,-5.04542284568));
#53742=CARTESIAN_POINT('Ctrl Pts',(-1.67362302807,-35.4364054801,-5.0454821464));
#53743=CARTESIAN_POINT('Ctrl Pts',(-1.67696448333,-35.4768981249,-5.04371406628));
#53744=CARTESIAN_POINT('Ctrl Pts',(-1.61326364266,-35.2619218696,-5.05000316771));
#53745=CARTESIAN_POINT('Ctrl Pts',(-1.62236549352,-35.3070877788,-5.05662956819));
#53746=CARTESIAN_POINT('Ctrl Pts',(-1.63007921825,-35.3528484277,-5.0610482607));
#53747=CARTESIAN_POINT('Ctrl Pts',(-1.63636464034,-35.3990097556,-5.06322951683));
#53748=CARTESIAN_POINT('Ctrl Pts',(-1.64119504878,-35.4453707616,-5.06316361876));
#53749=CARTESIAN_POINT('Ctrl Pts',(-1.64455688984,-35.4917317677,-5.06086202998));
#53750=CARTESIAN_POINT('Ctrl Pts',(-1.57763814761,-35.2502524393,-5.07162003768));
#53751=CARTESIAN_POINT('Ctrl Pts',(-1.58925529962,-35.3001212511,-5.07894359568));
#53752=CARTESIAN_POINT('Ctrl Pts',(-1.59886212553,-35.350806501,-5.08374537669));
#53753=CARTESIAN_POINT('Ctrl Pts',(-1.60640164997,-35.4020401921,-5.08598819927));
#53754=CARTESIAN_POINT('Ctrl Pts',(-1.6118338475,-35.4535491166,-5.08566006898));
#53755=CARTESIAN_POINT('Ctrl Pts',(-1.61513825447,-35.505058041,-5.08277314744));
#53756=CARTESIAN_POINT('Ctrl Pts',(-1.5467652741,-35.2408307961,-5.09796224817));
#53757=CARTESIAN_POINT('Ctrl Pts',(-1.56082810828,-35.2948250485,-5.10559533807));
#53758=CARTESIAN_POINT('Ctrl Pts',(-1.5721279205,-35.3498911181,-5.11056679276));
#53759=CARTESIAN_POINT('Ctrl Pts',(-1.58057518036,-35.4056813318,-5.11281573481));
#53760=CARTESIAN_POINT('Ctrl Pts',(-1.58611547612,-35.4618331019,-5.11233170678));
#53761=CARTESIAN_POINT('Ctrl Pts',(-1.58873141496,-35.5179848719,-5.10914094848));
#53762=CARTESIAN_POINT('Ctrl Pts',(-1.50094788409,-35.2255784603,-5.15114151002));
#53763=CARTESIAN_POINT('Ctrl Pts',(-1.51919307915,-35.2853745424,-5.15844241592));
#53764=CARTESIAN_POINT('Ctrl Pts',(-1.53333303669,-35.34668297,-5.16330955045));
#53765=CARTESIAN_POINT('Ctrl Pts',(-1.54322139667,-35.4090153954,-5.16568966994));
#53766=CARTESIAN_POINT('Ctrl Pts',(-1.54877729981,-35.471860276,-5.16555970229));
#53767=CARTESIAN_POINT('Ctrl Pts',(-1.54998925981,-35.5347051565,-5.16293840519));
#53768=CARTESIAN_POINT('Ctrl Pts',(-1.47301395752,-35.2164048258,-5.21579034781));
#53769=CARTESIAN_POINT('Ctrl Pts',(-1.49420720065,-35.2792319381,-5.22072059065));
#53770=CARTESIAN_POINT('Ctrl Pts',(-1.51037196702,-35.3438574448,-5.22412710654));
#53771=CARTESIAN_POINT('Ctrl Pts',(-1.52131309724,-35.4097044807,-5.22595779822));
#53772=CARTESIAN_POINT('Ctrl Pts',(-1.52692924844,-35.4761620333,-5.22619785569));
#53773=CARTESIAN_POINT('Ctrl Pts',(-1.52721834654,-35.5426195859,-5.22486268019));
#53774=CARTESIAN_POINT('Ctrl Pts',(-1.46470315626,-35.213766631,-5.24531814123));
#53775=CARTESIAN_POINT('Ctrl Pts',(-1.48680690707,-35.277355512,-5.24884399471));
#53776=CARTESIAN_POINT('Ctrl Pts',(-1.50361778858,-35.3428209065,-5.25131648121));
#53777=CARTESIAN_POINT('Ctrl Pts',(-1.51492750077,-35.4095603027,-5.25272449316));
#53778=CARTESIAN_POINT('Ctrl Pts',(-1.52062825527,-35.4769374515,-5.25304460068));
#53779=CARTESIAN_POINT('Ctrl Pts',(-1.52071813077,-35.5443146003,-5.25227472437));
#53780=CARTESIAN_POINT('Ctrl Pts',(-1.46069629729,-35.2129478838,-5.27610920663));
#53781=CARTESIAN_POINT('Ctrl Pts',(-1.48316494179,-35.2768382352,-5.27796326442));
#53782=CARTESIAN_POINT('Ctrl Pts',(-1.50022470946,-35.3426337834,-5.2792979259));
#53783=CARTESIAN_POINT('Ctrl Pts',(-1.51165995618,-35.4097245745,-5.28008044471));
#53784=CARTESIAN_POINT('Ctrl Pts',(-1.51736021529,-35.4774626159,-5.28030986048));
#53785=CARTESIAN_POINT('Ctrl Pts',(-1.51732687674,-35.5452006575,-5.27999548691));
#53786=CARTESIAN_POINT('Ctrl Pts',(-1.46090316329,-35.2135376551,-5.30645216923));
#53787=CARTESIAN_POINT('Ctrl Pts',(-1.48323786433,-35.277208474,-5.30683297122));
#53788=CARTESIAN_POINT('Ctrl Pts',(-1.50020219619,-35.3427631323,-5.30721377032));
#53789=CARTESIAN_POINT('Ctrl Pts',(-1.51158410625,-35.4095977304,-5.30759095434));
#53790=CARTESIAN_POINT('Ctrl Pts',(-1.51727462121,-35.4770723771,-5.30796091202));
#53791=CARTESIAN_POINT('Ctrl Pts',(-1.51727394979,-35.5445470238,-5.30832023528));
#53792=CARTESIAN_POINT('Ctrl Pts',(-1.65073607089,-35.2758272825,-5.03428274092));
#53793=CARTESIAN_POINT('Ctrl Pts',(-1.61326364266,-35.2619218696,-5.05000316771));
#53794=CARTESIAN_POINT('Ctrl Pts',(-1.57763814761,-35.2502524393,-5.07162003768));
#53795=CARTESIAN_POINT('Ctrl Pts',(-1.5467652741,-35.2408307961,-5.09796224817));
#53796=CARTESIAN_POINT('Ctrl Pts',(-1.50094788409,-35.2255784603,-5.15114151002));
#53797=CARTESIAN_POINT('Ctrl Pts',(-1.47301395752,-35.2164048258,-5.21579034781));
#53798=CARTESIAN_POINT('Ctrl Pts',(-1.46470315626,-35.213766631,-5.24531814123));
#53799=CARTESIAN_POINT('Ctrl Pts',(-1.46069629729,-35.2129478838,-5.27610920663));
#53800=CARTESIAN_POINT('Ctrl Pts',(-1.46090316329,-35.2135376551,-5.30645216923));
#53801=CARTESIAN_POINT('Origin',(-0.517273476326547,-35.5445474017573,-5.30645165992553));
#53802=CARTESIAN_POINT('Ctrl Pts',(-3.48890306473,-35.2652540838,-3.21461371005));
#53803=CARTESIAN_POINT('Ctrl Pts',(-3.49935367494,-35.3079501575,-3.21504790568));
#53804=CARTESIAN_POINT('Ctrl Pts',(-3.50770783242,-35.351170349,-3.21440294636));
#53805=CARTESIAN_POINT('Ctrl Pts',(-3.51392345177,-35.3947427768,-3.21267707712));
#53806=CARTESIAN_POINT('Ctrl Pts',(-3.51797541026,-35.4384913267,-3.20987727374));
#53807=CARTESIAN_POINT('Ctrl Pts',(-3.51985615043,-35.4822398766,-3.20601907528));
#53808=CARTESIAN_POINT('Ctrl Pts',(-3.24150677815,-35.2297273503,-3.67797056337));
#53809=CARTESIAN_POINT('Ctrl Pts',(-3.25788366108,-35.2867834422,-3.68259788135));
#53810=CARTESIAN_POINT('Ctrl Pts',(-3.2708619246,-35.3449131549,-3.6851550674));
#53811=CARTESIAN_POINT('Ctrl Pts',(-3.28034612237,-35.4037663878,-3.68562224436));
#53812=CARTESIAN_POINT('Ctrl Pts',(-3.28628025023,-35.4629813934,-3.68400243047));
#53813=CARTESIAN_POINT('Ctrl Pts',(-3.28864951001,-35.5221963991,-3.68032135));
#53814=CARTESIAN_POINT('Ctrl Pts',(-2.93020007641,-35.2159821642,-4.09471223066));
#53815=CARTESIAN_POINT('Ctrl Pts',(-2.94976329618,-35.2791022779,-4.10741039029));
#53816=CARTESIAN_POINT('Ctrl Pts',(-2.96507838407,-35.3440365738,-4.11671739461));
#53817=CARTESIAN_POINT('Ctrl Pts',(-2.97596822876,-35.4101991223,-4.12255014873));
#53818=CARTESIAN_POINT('Ctrl Pts',(-2.98233164479,-35.4769758456,-4.12487890497));
#53819=CARTESIAN_POINT('Ctrl Pts',(-2.984147828,-35.543752569,-4.12372796686));
#53820=CARTESIAN_POINT('Ctrl Pts',(-2.57349039398,-35.21650702,-4.45141980073));
#53821=CARTESIAN_POINT('Ctrl Pts',(-2.58535390407,-35.2792535748,-4.47101557567));
#53822=CARTESIAN_POINT('Ctrl Pts',(-2.59391358392,-35.3437511415,-4.48640413787));
#53823=CARTESIAN_POINT('Ctrl Pts',(-2.59909669842,-35.4094332325,-4.49741590343));
#53824=CARTESIAN_POINT('Ctrl Pts',(-2.60088024578,-35.4757076219,-4.50395318786));
#53825=CARTESIAN_POINT('Ctrl Pts',(-2.59929137485,-35.5419820113,-4.50599426346));
#53826=CARTESIAN_POINT('Ctrl Pts',(-2.15330460094,-35.2313461468,-4.76288665231));
#53827=CARTESIAN_POINT('Ctrl Pts',(-2.15740174514,-35.2874140925,-4.77869293776));
#53828=CARTESIAN_POINT('Ctrl Pts',(-2.15952364918,-35.3444755753,-4.7912469843));
#53829=CARTESIAN_POINT('Ctrl Pts',(-2.15965446887,-35.4022061334,-4.8004623347));
#53830=CARTESIAN_POINT('Ctrl Pts',(-2.15779886139,-35.4602712393,-4.80628788231));
#53831=CARTESIAN_POINT('Ctrl Pts',(-2.15398176798,-35.5183363452,-4.80870937341));
#53832=CARTESIAN_POINT('Ctrl Pts',(-1.69382497102,-35.2682575054,-5.0104353994));
#53833=CARTESIAN_POINT('Ctrl Pts',(-1.69402180198,-35.3094041642,-5.02023545326));
#53834=CARTESIAN_POINT('Ctrl Pts',(-1.69321049227,-35.3510179116,-5.02809462923));
#53835=CARTESIAN_POINT('Ctrl Pts',(-1.69139030263,-35.3929453813,-5.0339763881));
#53836=CARTESIAN_POINT('Ctrl Pts',(-1.68856804274,-35.4350297152,-5.03785872515));
#53837=CARTESIAN_POINT('Ctrl Pts',(-1.68475791979,-35.477114049,-5.03973465917));
#53838=CARTESIAN_POINT('',(-3.48890306745266,-35.2652540841568,-3.21461371228527));
#53839=CARTESIAN_POINT('Origin',(-2.62096730277507,-35.4822399141373,-2.76784133732473));
#53840=CARTESIAN_POINT('Ctrl Pts',(-3.48890306888,-35.2652540838,-3.21461371302));
#53841=CARTESIAN_POINT('Ctrl Pts',(-3.24150677815,-35.2297273503,-3.67797056337));
#53842=CARTESIAN_POINT('Ctrl Pts',(-2.93020007641,-35.2159821642,-4.09471223066));
#53843=CARTESIAN_POINT('Ctrl Pts',(-2.57349039398,-35.21650702,-4.45141980073));
#53844=CARTESIAN_POINT('Ctrl Pts',(-2.15330460094,-35.2313461468,-4.76288665231));
#53845=CARTESIAN_POINT('Ctrl Pts',(-1.69382496468,-35.2682576589,-5.01043545515));
#53846=CARTESIAN_POINT('Ctrl Pts',(-3.68960640636,-35.2436867043,-3.0159715009));
#53847=CARTESIAN_POINT('Ctrl Pts',(-3.68994006064,-35.2950048915,-3.03107790447));
#53848=CARTESIAN_POINT('Ctrl Pts',(-3.68889543318,-35.347263528,-3.04301993635));
#53849=CARTESIAN_POINT('Ctrl Pts',(-3.68647051515,-35.4001566503,-3.05170748236));
#53850=CARTESIAN_POINT('Ctrl Pts',(-3.68267985005,-35.4533670311,-3.05708843877));
#53851=CARTESIAN_POINT('Ctrl Pts',(-3.67755401867,-35.5065774118,-3.05915055738));
#53852=CARTESIAN_POINT('Ctrl Pts',(-3.68406493808,-35.2441669878,-3.01852789669));
#53853=CARTESIAN_POINT('Ctrl Pts',(-3.6852545996,-35.2952993243,-3.03313678947));
#53854=CARTESIAN_POINT('Ctrl Pts',(-3.68508444483,-35.3473574121,-3.04461628848));
#53855=CARTESIAN_POINT('Ctrl Pts',(-3.68354738519,-35.4000399811,-3.05288030368));
#53856=CARTESIAN_POINT('Ctrl Pts',(-3.68065246874,-35.4530348056,-3.05787988529));
#53857=CARTESIAN_POINT('Ctrl Pts',(-3.67642456268,-35.5060296301,-3.05960493674));
#53858=CARTESIAN_POINT('Ctrl Pts',(-3.67853556896,-35.2447691838,-3.02110736508));
#53859=CARTESIAN_POINT('Ctrl Pts',(-3.68058228399,-35.295713802,-3.03522035827));
#53860=CARTESIAN_POINT('Ctrl Pts',(-3.68128649848,-35.3475703565,-3.04623632347));
#53861=CARTESIAN_POINT('Ctrl Pts',(-3.68063618362,-35.4000419929,-3.05407302366));
#53862=CARTESIAN_POINT('Ctrl Pts',(-3.67863507204,-35.4528211843,-3.05868456544));
#53863=CARTESIAN_POINT('Ctrl Pts',(-3.67530251301,-35.5056003757,-3.0600629924));
#53864=CARTESIAN_POINT('Ctrl Pts',(-3.67302394084,-35.2454929622,-3.02370658462));
#53865=CARTESIAN_POINT('Ctrl Pts',(-3.6759278736,-35.2962481955,-3.03732595805));
#53866=CARTESIAN_POINT('Ctrl Pts',(-3.67750544789,-35.3479024371,-3.04787800394));
#53867=CARTESIAN_POINT('Ctrl Pts',(-3.67773982365,-35.4001629685,-3.05528416988));
#53868=CARTESIAN_POINT('Ctrl Pts',(-3.67662956704,-35.4527266586,-3.05950153137));
#53869=CARTESIAN_POINT('Ctrl Pts',(-3.67418869929,-35.5052903486,-3.06052426199));
#53870=CARTESIAN_POINT('Ctrl Pts',(-3.6675348968,-35.2463373792,-3.02632251085));
#53871=CARTESIAN_POINT('Ctrl Pts',(-3.67129543056,-35.2969017565,-3.03945109726));
#53872=CARTESIAN_POINT('Ctrl Pts',(-3.67374456646,-35.348353094,-3.04953936585));
#53873=CARTESIAN_POINT('Ctrl Pts',(-3.67486076111,-35.4004025315,-3.05651229579));
#53874=CARTESIAN_POINT('Ctrl Pts',(-3.67463755638,-35.4527510324,-3.06032984675));
#53875=CARTESIAN_POINT('Ctrl Pts',(-3.67308380368,-35.5050995333,-3.0609883158));
#53876=CARTESIAN_POINT('Ctrl Pts',(-3.66207264655,-35.2473009405,-3.02895231242));
#53877=CARTESIAN_POINT('Ctrl Pts',(-3.66668846955,-35.2976731782,-3.04159341678));
#53878=CARTESIAN_POINT('Ctrl Pts',(-3.67000667781,-35.348921195,-3.05121851933));
#53879=CARTESIAN_POINT('Ctrl Pts',(-3.67200111268,-35.4007597143,-3.05775598766));
#53880=CARTESIAN_POINT('Ctrl Pts',(-3.67266041516,-35.4528934978,-3.0611685886));
#53881=CARTESIAN_POINT('Ctrl Pts',(-3.67198840819,-35.5050272814,-3.06145474134));
#53882=CARTESIAN_POINT('',(-3.68960640636,-35.2436867043,-3.0159715009));
#53883=CARTESIAN_POINT('Origin',(-3.30432478046144,-35.5065775306539,-2.13141045567169));
#53884=CARTESIAN_POINT('Origin',(-3.69828822169992,-35.4059562737349,-3.04854457261671));
#53885=CARTESIAN_POINT('Origin',(-3.28022457192059,-35.5050282606332,-2.14138812518752));
#53886=CARTESIAN_POINT('Ctrl Pts',(-3.66207294828,-35.2473021021,-3.02895254907));
#53887=CARTESIAN_POINT('Ctrl Pts',(-3.66668938645,-35.2976742927,-3.04159327346));
#53888=CARTESIAN_POINT('Ctrl Pts',(-3.67000827764,-35.3489222549,-3.05121799304));
#53889=CARTESIAN_POINT('Ctrl Pts',(-3.67200345992,-35.4007607145,-3.05775507809));
#53890=CARTESIAN_POINT('Ctrl Pts',(-3.6726635701,-35.4528944359,-3.06116729793));
#53891=CARTESIAN_POINT('Ctrl Pts',(-3.67199242621,-35.5050281572,-3.06145307387));
#53892=CARTESIAN_POINT('Ctrl Pts',(-3.64556722008,-35.248406313,-3.03637428958));
#53893=CARTESIAN_POINT('Ctrl Pts',(-3.65069501362,-35.2983832695,-3.04859774823));
#53894=CARTESIAN_POINT('Ctrl Pts',(-3.65437679925,-35.3492138965,-3.0579274977));
#53895=CARTESIAN_POINT('Ctrl Pts',(-3.65658079285,-35.4006204961,-3.06429584207));
#53896=CARTESIAN_POINT('Ctrl Pts',(-3.65729581475,-35.4523147284,-3.06766652406));
#53897=CARTESIAN_POINT('Ctrl Pts',(-3.65652775557,-35.5040089607,-3.06803796128));
#53898=CARTESIAN_POINT('Ctrl Pts',(-3.62977987226,-35.2496170208,-3.04490879463));
#53899=CARTESIAN_POINT('Ctrl Pts',(-3.63528692384,-35.2991304944,-3.05669637995));
#53900=CARTESIAN_POINT('Ctrl Pts',(-3.63920530469,-35.3494729369,-3.06573183442));
#53901=CARTESIAN_POINT('Ctrl Pts',(-3.6415096169,-35.4003733514,-3.07195030901));
#53902=CARTESIAN_POINT('Ctrl Pts',(-3.6421854279,-35.4515533116,-3.07531862585));
#53903=CARTESIAN_POINT('Ctrl Pts',(-3.64123559569,-35.5027332718,-3.07583329833));
#53904=CARTESIAN_POINT('Ctrl Pts',(-3.61439747244,-35.2508930805,-3.05469265108));
#53905=CARTESIAN_POINT('Ctrl Pts',(-3.62030288916,-35.2998487222,-3.06596829565));
#53906=CARTESIAN_POINT('Ctrl Pts',(-3.62450774723,-35.349603179,-3.07465066951));
#53907=CARTESIAN_POINT('Ctrl Pts',(-3.62697838143,-35.3998970016,-3.08067727275));
#53908=CARTESIAN_POINT('Ctrl Pts',(-3.6277014573,-35.4504596751,-3.08401633821));
#53909=CARTESIAN_POINT('Ctrl Pts',(-3.62668459499,-35.5010223485,-3.0846663226));
#53910=CARTESIAN_POINT('Ctrl Pts',(-3.57818606717,-35.254427601,-3.08171182978));
#53911=CARTESIAN_POINT('Ctrl Pts',(-3.58499819528,-35.3018787149,-3.09155249699));
#53912=CARTESIAN_POINT('Ctrl Pts',(-3.58987595331,-35.3500528463,-3.09920396626));
#53913=CARTESIAN_POINT('Ctrl Pts',(-3.59278825537,-35.398712151,-3.1046211988));
#53914=CARTESIAN_POINT('Ctrl Pts',(-3.5937205131,-35.4476152765,-3.10777655729));
#53915=CARTESIAN_POINT('Ctrl Pts',(-3.59267477187,-35.4965184022,-3.10866282874));
#53916=CARTESIAN_POINT('Ctrl Pts',(-3.54680562214,-35.2591381386,-3.11518399273));
#53917=CARTESIAN_POINT('Ctrl Pts',(-3.55425275129,-35.3047560463,-3.12331909977));
#53918=CARTESIAN_POINT('Ctrl Pts',(-3.55966404915,-35.3510104673,-3.12970468618));
#53919=CARTESIAN_POINT('Ctrl Pts',(-3.56300079879,-35.3976954964,-3.13429853608));
#53920=CARTESIAN_POINT('Ctrl Pts',(-3.56424741272,-35.4445940509,-3.13708068529));
#53921=CARTESIAN_POINT('Ctrl Pts',(-3.56341230092,-35.4914926054,-3.13805072514));
#53922=CARTESIAN_POINT('Ctrl Pts',(-3.53059439149,-35.2625776925,-3.1368950068));
#53923=CARTESIAN_POINT('Ctrl Pts',(-3.53819496617,-35.3070386414,-3.14399854711));
#53924=CARTESIAN_POINT('Ctrl Pts',(-3.54372649014,-35.3520895186,-3.14959798998));
#53925=CARTESIAN_POINT('Ctrl Pts',(-3.5471637516,-35.3975290806,-3.15368535098));
#53926=CARTESIAN_POINT('Ctrl Pts',(-3.54849609615,-35.4431689738,-3.15623708405));
#53927=CARTESIAN_POINT('Ctrl Pts',(-3.54771350151,-35.4888088673,-3.15723408602));
#53928=CARTESIAN_POINT('Ctrl Pts',(-3.51717283568,-35.2661737422,-3.15933443135));
#53929=CARTESIAN_POINT('Ctrl Pts',(-3.52465704951,-35.3092672059,-3.16566526845));
#53930=CARTESIAN_POINT('Ctrl Pts',(-3.53010225982,-35.3528915117,-3.17076845393));
#53931=CARTESIAN_POINT('Ctrl Pts',(-3.53347292436,-35.3968779115,-3.17460348458));
#53932=CARTESIAN_POINT('Ctrl Pts',(-3.53475243752,-35.4410413734,-3.17715872601));
#53933=CARTESIAN_POINT('Ctrl Pts',(-3.53395300191,-35.485204835,-3.17843874804));
#53934=CARTESIAN_POINT('Ctrl Pts',(-3.50597877122,-35.2696531524,-3.18321806272));
#53935=CARTESIAN_POINT('Ctrl Pts',(-3.51333812365,-35.3113502754,-3.18868521568));
#53936=CARTESIAN_POINT('Ctrl Pts',(-3.51870904583,-35.3535297557,-3.19315013683));
#53937=CARTESIAN_POINT('Ctrl Pts',(-3.52206358055,-35.3960332589,-3.19659205988));
#53938=CARTESIAN_POINT('Ctrl Pts',(-3.52338894151,-35.4386987766,-3.19899786544));
#53939=CARTESIAN_POINT('Ctrl Pts',(-3.5226878028,-35.4813642944,-3.200362378));
#53940=CARTESIAN_POINT('Origin',(-2.63323785737628,-35.4813643327716,-2.74332899791325));
#53941=CARTESIAN_POINT('Ctrl Pts',(-3.50597880735,-35.2696545374,-3.18321831335));
#53942=CARTESIAN_POINT('Ctrl Pts',(-3.51333803189,-35.3113514663,-3.18868569298));
#53943=CARTESIAN_POINT('Ctrl Pts',(-3.51870881162,-35.353530752,-3.19315085121));
#53944=CARTESIAN_POINT('Ctrl Pts',(-3.52206318971,-35.3960340603,-3.19659302084));
#53945=CARTESIAN_POINT('Ctrl Pts',(-3.52338838043,-35.4386993829,-3.1989990815));
#53946=CARTESIAN_POINT('Ctrl Pts',(-3.52268705855,-35.4813647056,-3.20036385665));
#53947=CARTESIAN_POINT('Ctrl Pts',(-3.50256004198,-35.268393509,-3.18939410052));
#53948=CARTESIAN_POINT('Ctrl Pts',(-3.51052316476,-35.3102955518,-3.1938621313));
#53949=CARTESIAN_POINT('Ctrl Pts',(-3.51648359784,-35.3526863763,-3.19731644996));
#53950=CARTESIAN_POINT('Ctrl Pts',(-3.52041085984,-35.3954055593,-3.19973991273));
#53951=CARTESIAN_POINT('Ctrl Pts',(-3.52228987577,-35.4382889251,-3.2011231722));
#53952=CARTESIAN_POINT('Ctrl Pts',(-3.52212131885,-35.4811722908,-3.20146489487));
#53953=CARTESIAN_POINT('Ctrl Pts',(-3.49913203155,-35.2673150056,-3.1956382498));
#53954=CARTESIAN_POINT('Ctrl Pts',(-3.50770826391,-35.3094204104,-3.19910017162));
#53955=CARTESIAN_POINT('Ctrl Pts',(-3.51426388564,-35.3520219724,-3.20153494382));
#53956=CARTESIAN_POINT('Ctrl Pts',(-3.5187657727,-35.3949568785,-3.20292908338));
#53957=CARTESIAN_POINT('Ctrl Pts',(-3.52119645205,-35.4380584515,-3.20327716833));
#53958=CARTESIAN_POINT('Ctrl Pts',(-3.52155459752,-35.4811600245,-3.20258180379));
#53959=CARTESIAN_POINT('Ctrl Pts',(-3.49570498282,-35.2664275319,-3.20193555292));
#53960=CARTESIAN_POINT('Ctrl Pts',(-3.5049017062,-35.3087336513,-3.20438752525));
#53961=CARTESIAN_POINT('Ctrl Pts',(-3.51205619329,-35.3515442739,-3.2057969486));
#53962=CARTESIAN_POINT('Ctrl Pts',(-3.51713243885,-35.3946938503,-3.20615423225));
#53963=CARTESIAN_POINT('Ctrl Pts',(-3.52011064813,-35.4380129429,-3.20545771792));
#53964=CARTESIAN_POINT('Ctrl Pts',(-3.52098739307,-35.4813320354,-3.20371424309));
#53965=CARTESIAN_POINT('Ctrl Pts',(-3.49229725928,-35.2657414976,-3.2082566117));
#53966=CARTESIAN_POINT('Ctrl Pts',(-3.50211831443,-35.308244275,-3.20970015733));
#53967=CARTESIAN_POINT('Ctrl Pts',(-3.50987186481,-35.3512608603,-3.21008384904));
#53968=CARTESIAN_POINT('Ctrl Pts',(-3.51551898686,-35.3946227115,-3.20940189333));
#53969=CARTESIAN_POINT('Ctrl Pts',(-3.51903723035,-35.4381571989,-3.20765694424));
#53970=CARTESIAN_POINT('Ctrl Pts',(-3.52042115146,-35.4816916863,-3.20486003554));
#53971=CARTESIAN_POINT('Ctrl Pts',(-3.4889030666,-35.265254082,-3.21461371656));
#53972=CARTESIAN_POINT('Ctrl Pts',(-3.49935367791,-35.3079501561,-3.21504791216));
#53973=CARTESIAN_POINT('Ctrl Pts',(-3.50770783634,-35.3511703481,-3.21440295273));
#53974=CARTESIAN_POINT('Ctrl Pts',(-3.51392345649,-35.3947427765,-3.21267708331));
#53975=CARTESIAN_POINT('Ctrl Pts',(-3.51797541562,-35.4384913269,-3.20987727967));
#53976=CARTESIAN_POINT('Ctrl Pts',(-3.51985615629,-35.4822398773,-3.20601908088));
#53977=CARTESIAN_POINT('Origin',(-3.5116682051481,-35.3848727889406,-3.20631688515481));
#53978=CARTESIAN_POINT('Ctrl Pts',(-7.05021190275,-35.3742261151,1.16209541223));
#53979=CARTESIAN_POINT('Ctrl Pts',(-7.05021190275,-35.3742261151,1.16209541223));
#53980=CARTESIAN_POINT('Ctrl Pts',(-7.05021190275,-35.3742261151,1.16209541223));
#53981=CARTESIAN_POINT('Ctrl Pts',(-7.05021190275,-35.3742261151,1.16209541223));
#53982=CARTESIAN_POINT('Ctrl Pts',(-7.05021190275,-35.3742261151,1.16209541223));
#53983=CARTESIAN_POINT('Ctrl Pts',(-7.05021190275,-35.3742261151,1.16209541223));
#53984=CARTESIAN_POINT('Ctrl Pts',(-7.01340171355,-35.3233663073,0.887814197822));
#53985=CARTESIAN_POINT('Ctrl Pts',(-7.01381986471783,-35.3413180972,0.890929938671949));
#53986=CARTESIAN_POINT('Ctrl Pts',(-7.01423801594781,-35.3592698878,0.894045679984952));
#53987=CARTESIAN_POINT('Ctrl Pts',(-7.01465616709811,-35.377221677,0.897161420704254));
#53988=CARTESIAN_POINT('Ctrl Pts',(-7.01507431822199,-35.3951734669,0.900277161226733));
#53989=CARTESIAN_POINT('Ctrl Pts',(-7.01549246939,-35.4131252568,0.903392902078));
#53990=CARTESIAN_POINT('Ctrl Pts',(-6.95185482919,-35.2775995372,0.614848488511));
#53991=CARTESIAN_POINT('Ctrl Pts',(-6.95711039026,-35.3122184667,0.620033495106));
#53992=CARTESIAN_POINT('Ctrl Pts',(-6.96131634916,-35.3468297586,0.625353240693));
#53993=CARTESIAN_POINT('Ctrl Pts',(-6.96447793891,-35.3814361808,0.630808421027));
#53994=CARTESIAN_POINT('Ctrl Pts',(-6.96659784091,-35.4160401708,0.636399696014));
#53995=CARTESIAN_POINT('Ctrl Pts',(-6.96767646618,-35.4506441608,0.642127552041));
#53996=CARTESIAN_POINT('Ctrl Pts',(-6.8673530143,-35.2439788226,0.343363482131));
#53997=CARTESIAN_POINT('Ctrl Pts',(-6.87994051011,-35.2916209137,0.34796525773));
#53998=CARTESIAN_POINT('Ctrl Pts',(-6.88986767191,-35.3397700495,0.353240035009));
#53999=CARTESIAN_POINT('Ctrl Pts',(-6.89711069428,-35.38825575,0.359155938781));
#54000=CARTESIAN_POINT('Ctrl Pts',(-6.90165550114,-35.4369097195,0.365681814414));
#54001=CARTESIAN_POINT('Ctrl Pts',(-6.90349674466,-35.485563689,0.372787607728));
#54002=CARTESIAN_POINT('Ctrl Pts',(-6.64187024435,-35.1886753155,-0.23870995558));
#54003=CARTESIAN_POINT('Ctrl Pts',(-6.66955139679,-35.2585364198,-0.239842936739));
#54004=CARTESIAN_POINT('Ctrl Pts',(-6.691390474,-35.3305802147,-0.238616506959));
#54005=CARTESIAN_POINT('Ctrl Pts',(-6.70712809876,-35.4041022846,-0.23504887133));
#54006=CARTESIAN_POINT('Ctrl Pts',(-6.71661554426,-35.4783635248,-0.229196354076));
#54007=CARTESIAN_POINT('Ctrl Pts',(-6.71982081074,-35.5526247648,-0.221149174844));
#54008=CARTESIAN_POINT('Ctrl Pts',(-6.335633879,-35.1655247078,-0.779903703387));
#54009=CARTESIAN_POINT('Ctrl Pts',(-6.37258533768,-35.2460676029,-0.793096558606));
#54010=CARTESIAN_POINT('Ctrl Pts',(-6.40175618506,-35.3308011559,-0.801727405553));
#54011=CARTESIAN_POINT('Ctrl Pts',(-6.42255691503,-35.4184152395,-0.805611032625));
#54012=CARTESIAN_POINT('Ctrl Pts',(-6.43465051901,-35.5074700242,-0.804704006103));
#54013=CARTESIAN_POINT('Ctrl Pts',(-6.43798249823,-35.5965248091,-0.799107100072));
#54014=CARTESIAN_POINT('Ctrl Pts',(-6.1477485618,-35.1585065417,-1.0593892471));
#54015=CARTESIAN_POINT('Ctrl Pts',(-6.1862455007,-35.2425122041,-1.07972455995));
#54016=CARTESIAN_POINT('Ctrl Pts',(-6.21657209688,-35.331564736,-1.09437680653));
#54017=CARTESIAN_POINT('Ctrl Pts',(-6.23800931387,-35.4241081414,-1.10297704478));
#54018=CARTESIAN_POINT('Ctrl Pts',(-6.25014939755,-35.5183977765,-1.10536973107));
#54019=CARTESIAN_POINT('Ctrl Pts',(-6.25293978467,-35.6126874115,-1.1016283265));
#54020=CARTESIAN_POINT('Ctrl Pts',(-5.64263928747,-35.1503549657,-1.69778761613));
#54021=CARTESIAN_POINT('Ctrl Pts',(-5.6781072677,-35.2388302664,-1.73263418024));
#54022=CARTESIAN_POINT('Ctrl Pts',(-5.70553308479,-35.3334375132,-1.75965360778));
#54023=CARTESIAN_POINT('Ctrl Pts',(-5.72416357539,-35.4323082835,-1.77811755991));
#54024=CARTESIAN_POINT('Ctrl Pts',(-5.7335949111,-35.5333121034,-1.78763419494));
#54025=CARTESIAN_POINT('Ctrl Pts',(-5.73382235555,-35.6343159234,-1.78819570677));
#54026=CARTESIAN_POINT('Ctrl Pts',(-5.01710815157,-35.1629277461,-2.24626629333));
#54027=CARTESIAN_POINT('Ctrl Pts',(-5.03812134505,-35.2465940911,-2.28433468893));
#54028=CARTESIAN_POINT('Ctrl Pts',(-5.05330548672,-35.3352292266,-2.31441076458));
#54029=CARTESIAN_POINT('Ctrl Pts',(-5.06229638123,-35.4272996663,-2.33577662822));
#54030=CARTESIAN_POINT('Ctrl Pts',(-5.06494250992,-35.5210885082,-2.34802021045));
#54031=CARTESIAN_POINT('Ctrl Pts',(-5.06131871348,-35.6148773502,-2.35107992573));
#54032=CARTESIAN_POINT('Ctrl Pts',(-4.60859161999,-35.1762367254,-2.53785301358));
#54033=CARTESIAN_POINT('Ctrl Pts',(-4.61998718798,-35.2544472454,-2.57156731299));
#54034=CARTESIAN_POINT('Ctrl Pts',(-4.62723219199,-35.3360986017,-2.59812098394));
#54035=CARTESIAN_POINT('Ctrl Pts',(-4.63022512886,-35.4200944121,-2.61708014375));
#54036=CARTESIAN_POINT('Ctrl Pts',(-4.62896118843,-35.5052625726,-2.62819842135));
#54037=CARTESIAN_POINT('Ctrl Pts',(-4.62352979415,-35.5904307331,-2.63143094545));
#54038=CARTESIAN_POINT('Ctrl Pts',(-4.16372827527,-35.2025940852,-2.79724907986));
#54039=CARTESIAN_POINT('Ctrl Pts',(-4.16779886982,-35.2702188379,-2.82151459563));
#54040=CARTESIAN_POINT('Ctrl Pts',(-4.16935260067,-35.3397404397,-2.84063625327));
#54041=CARTESIAN_POINT('Ctrl Pts',(-4.16836377754,-35.4105469366,-2.8544077757));
#54042=CARTESIAN_POINT('Ctrl Pts',(-4.16484831327,-35.4819959329,-2.86271080605));
#54043=CARTESIAN_POINT('Ctrl Pts',(-4.15886281142,-35.5534449291,-2.86552034537));
#54044=CARTESIAN_POINT('Ctrl Pts',(-3.68960640598,-35.2436867043,-3.01597150109));
#54045=CARTESIAN_POINT('Ctrl Pts',(-3.68994006034,-35.2950048916,-3.03107790462));
#54046=CARTESIAN_POINT('Ctrl Pts',(-3.68889543294,-35.347263528,-3.04301993645));
#54047=CARTESIAN_POINT('Ctrl Pts',(-3.68647051499,-35.4001566504,-3.05170748242));
#54048=CARTESIAN_POINT('Ctrl Pts',(-3.68267984997,-35.4533670311,-3.0570884388));
#54049=CARTESIAN_POINT('Ctrl Pts',(-3.67755401867,-35.5065774118,-3.05915055738));
#54050=CARTESIAN_POINT('Ctrl Pts',(-7.05021189275609,-35.3742261012918,
1.16209533776304));
#54051=CARTESIAN_POINT('Ctrl Pts',(-7.01340171769854,-35.3233670493629,
0.887814269053016));
#54052=CARTESIAN_POINT('Ctrl Pts',(-6.95185503558031,-35.2776009819157,
0.614848661487126));
#54053=CARTESIAN_POINT('Ctrl Pts',(-6.86735353046522,-35.2439808156064,
0.343363646181602));
#54054=CARTESIAN_POINT('Ctrl Pts',(-6.641871396359,-35.188678241423,-0.23871001639011));
#54055=CARTESIAN_POINT('Ctrl Pts',(-6.33563542689691,-35.1655280817574,
-0.779904256034562));
#54056=CARTESIAN_POINT('Ctrl Pts',(-6.14775017443704,-35.1585100607139,
-1.05939009894544));
#54057=CARTESIAN_POINT('Ctrl Pts',(-5.64264077322358,-35.1503586719484,
-1.69778907585251));
#54058=CARTESIAN_POINT('Ctrl Pts',(-5.01710903181186,-35.1629312508997,
-2.24626788801542));
#54059=CARTESIAN_POINT('Ctrl Pts',(-4.60859209734921,-35.1762400016533,
-2.53785442587224));
#54060=CARTESIAN_POINT('Ctrl Pts',(-4.16372844578607,-35.2025969180128,
-2.79725009634263));
#54061=CARTESIAN_POINT('Ctrl Pts',(-3.68960640636,-35.2436867043,-3.0159715009));
#54062=CARTESIAN_POINT('Ctrl Pts',(-3.67755550257331,-35.3742477797272,
-3.0591534519424));
#54063=CARTESIAN_POINT('Ctrl Pts',(-3.32386409198,-32.4742356128,-2.36922853848));
#54064=CARTESIAN_POINT('Ctrl Pts',(-4.22884692807269,-35.3742477797272,
-2.83737078185739));
#54065=CARTESIAN_POINT('Ctrl Pts',(-3.82968047509,-32.4742356128,-1.81532491987));
#54066=CARTESIAN_POINT('Ctrl Pts',(-4.75872659660362,-35.3742477797272,
-2.56236446563048));
#54067=CARTESIAN_POINT('Ctrl Pts',(-4.31529317605,-32.4742356128,-1.24297128633));
#54068=CARTESIAN_POINT('Ctrl Pts',(-5.25779759486713,-35.3742477797272,
-2.22279170313982));
#54069=CARTESIAN_POINT('Ctrl Pts',(-4.78073424536,-32.4742356128,-0.651925339842));
#54070=CARTESIAN_POINT('Ctrl Pts',(-6.1337700409067,-35.3742477797272,-1.39617908277916));
#54071=CARTESIAN_POINT('Ctrl Pts',(-5.66596200411,-32.4742356128,0.560784091783));
#54072=CARTESIAN_POINT('Ctrl Pts',(-6.70708334214704,-35.3742477797272,
-0.336679612997994));
#54073=CARTESIAN_POINT('Ctrl Pts',(-6.46037298138,-32.4742356128,1.83459706183));
#54074=CARTESIAN_POINT('Ctrl Pts',(-6.90223544201876,-35.3742477797272,
0.234409171633676));
#54075=CARTESIAN_POINT('Ctrl Pts',(-6.83383584614,-32.4742356128,2.48513748583));
#54076=CARTESIAN_POINT('Ctrl Pts',(-7.02153225855751,-35.3742477797272,
0.820419960836672));
#54077=CARTESIAN_POINT('Ctrl Pts',(-7.18368375786,-32.4742356128,3.149547989));
#54078=CARTESIAN_POINT('Ctrl Pts',(-7.07911812989542,-35.3742477797272,
1.41232328791478));
#54079=CARTESIAN_POINT('Ctrl Pts',(-7.50890612221,-32.4742356128,3.82595376918));
#54080=CARTESIAN_POINT('',(-7.50890612221,-32.4742356128,3.82595376918));
#54081=CARTESIAN_POINT('',(-7.07911993306,-35.3742356128,1.41233341424));
#54082=CARTESIAN_POINT('Ctrl Pts',(-7.50890612221,-32.4742356128,3.82595376918));
#54083=CARTESIAN_POINT('Ctrl Pts',(-6.96684733231567,-32.4742356128,2.69856605273344));
#54084=CARTESIAN_POINT('Ctrl Pts',(-6.34321709883092,-32.4742356128,1.612247552867));
#54085=CARTESIAN_POINT('Ctrl Pts',(-4.9426430764693,-32.4742356128,-0.461097896531036));
#54086=CARTESIAN_POINT('Ctrl Pts',(-4.1675411517523,-32.4742356128,-1.44534431497417));
#54087=CARTESIAN_POINT('Ctrl Pts',(-3.32386409198001,-32.4742356128,-2.36922853847999));
#54088=CARTESIAN_POINT('Ctrl Pts',(-7.07911993306,-35.3742356128,1.41233341424));
#54089=CARTESIAN_POINT('Ctrl Pts',(-7.50890612221,-32.4742356128,3.82595376918));
#54090=CARTESIAN_POINT('Ctrl Pts',(-7.09439816601,-35.3742356128,1.56936058085));
#54091=CARTESIAN_POINT('Ctrl Pts',(-7.59518497882,-32.4742356128,4.00539873882));
#54092=CARTESIAN_POINT('Ctrl Pts',(-7.10532841684,-35.3742356128,1.72680313633));
#54093=CARTESIAN_POINT('Ctrl Pts',(-7.6797307274,-32.4742356128,4.18568800425));
#54094=CARTESIAN_POINT('Ctrl Pts',(-7.08904842402,-35.3742356128,1.89842406838));
#54095=CARTESIAN_POINT('Ctrl Pts',(-7.76642508589,-32.4742356128,4.37540694872));
#54096=CARTESIAN_POINT('Ctrl Pts',(-7.1390862001,-35.3742356128,2.05065495714));
#54097=CARTESIAN_POINT('Ctrl Pts',(-7.84739395748,-32.4742356128,4.5573230698));
#54098=CARTESIAN_POINT('Ctrl Pts',(-7.21384189759,-35.3742356128,2.18958432614));
#54099=CARTESIAN_POINT('Ctrl Pts',(-7.92659403983,-32.4742356128,4.74000601033));
#54100=CARTESIAN_POINT('Ctrl Pts',(-7.92659403983,-32.4742356128,4.74000601033));
#54101=CARTESIAN_POINT('Ctrl Pts',(-7.85943746154874,-32.4742356128,4.58510262093531));
#54102=CARTESIAN_POINT('Ctrl Pts',(-7.79122837535821,-32.4742356128,4.43204332182943));
#54103=CARTESIAN_POINT('Ctrl Pts',(-7.65314301021617,-32.4742356128,4.12986259705412));
#54104=CARTESIAN_POINT('Ctrl Pts',(-7.58206613716612,-32.4742356128,3.97811383687775));
#54105=CARTESIAN_POINT('Ctrl Pts',(-7.50890612221,-32.4742356128,3.82595376918));
#54106=CARTESIAN_POINT('',(-7.21702818953265,-35.2986940617107,2.22615323676817));
#54107=CARTESIAN_POINT('Ctrl Pts',(-7.21702817531,-35.2986941477,2.22615317529));
#54108=CARTESIAN_POINT('Ctrl Pts',(-7.20692741189441,-35.3061131910589,
2.20294516691052));
#54109=CARTESIAN_POINT('Ctrl Pts',(-7.19719329525834,-35.3141912841077,
2.17900438661006));
#54110=CARTESIAN_POINT('Ctrl Pts',(-7.18796980246911,-35.3226070668248,
2.15465538142052));
#54111=CARTESIAN_POINT('Ctrl Pts',(-7.18234237094649,-35.3277416987947,
2.1397995819442));
#54112=CARTESIAN_POINT('Ctrl Pts',(-7.17690465211826,-35.3330009806929,
2.12479257546628));
#54113=CARTESIAN_POINT('Ctrl Pts',(-7.17168536591732,-35.3383049690758,
2.10971258769397));
#54114=CARTESIAN_POINT('Ctrl Pts',(-7.16774304131616,-35.342311272444,2.0983221016215));
#54115=CARTESIAN_POINT('Ctrl Pts',(-7.16392050826559,-35.3463755747386,
2.08687105022291));
#54116=CARTESIAN_POINT('Ctrl Pts',(-7.160224977354,-35.3504229454298,2.07538760256753));
#54117=CARTESIAN_POINT('Ctrl Pts',(-7.15647459950107,-35.3545303848657,
2.06373372419597));
#54118=CARTESIAN_POINT('Ctrl Pts',(-7.15285530677851,-35.3586203097449,
2.05204630782424));
#54119=CARTESIAN_POINT('Ctrl Pts',(-7.14937553131797,-35.3626673165653,
2.0403417618537));
#54120=CARTESIAN_POINT('Ctrl Pts',(-7.14731388684394,-35.3650650256538,
2.0334072303603));
#54121=CARTESIAN_POINT('Ctrl Pts',(-7.14530121097212,-35.3674486946293,
2.02646644336296));
#54122=CARTESIAN_POINT('Ctrl Pts',(-7.14333877168014,-35.3698214557652,
2.01952124225387));
#54123=CARTESIAN_POINT('Ctrl Pts',(-7.14233333890139,-35.3710371121333,
2.01596294983756));
#54124=CARTESIAN_POINT('Ctrl Pts',(-7.14133929086512,-35.3722572507634,
2.01239698022069));
#54125=CARTESIAN_POINT('Ctrl Pts',(-7.14035958693292,-35.3734664689908,
2.00883384018666));
#54126=CARTESIAN_POINT('Ctrl Pts',(-7.14015072156521,-35.3737242650467,
2.00807420604724));
#54127=CARTESIAN_POINT('Ctrl Pts',(-7.13994249884667,-35.3739817495794,
2.00731466330883));
#54128=CARTESIAN_POINT('Ctrl Pts',(-7.13973493084178,-35.3742390721046,
2.00655525500559));
#54129=CARTESIAN_POINT('Ctrl Pts',(-7.23545016824,-35.2863172732,2.26690461571));
#54130=CARTESIAN_POINT('Ctrl Pts',(-7.23162479878,-35.288610995,2.25877896783));
#54131=CARTESIAN_POINT('Ctrl Pts',(-7.22786970762,-35.291024056,2.2506285999));
#54132=CARTESIAN_POINT('Ctrl Pts',(-7.22418450574,-35.2935251725,2.24246594859));
#54133=CARTESIAN_POINT('Ctrl Pts',(-7.22057030307,-35.2960900286,2.23430349206));
#54134=CARTESIAN_POINT('Ctrl Pts',(-7.2170282235,-35.2986939836,2.22615333516));
#54135=CARTESIAN_POINT('Ctrl Pts',(-7.21702817531,-35.2986941477,2.22615317529));
#54136=CARTESIAN_POINT('Ctrl Pts',(-7.21896716995,-35.3316547085,2.21752764579));
#54137=CARTESIAN_POINT('Ctrl Pts',(-7.21961961863,-35.364857528,2.20953864245));
#54138=CARTESIAN_POINT('Ctrl Pts',(-7.218980814,-35.3982226387,2.20220709377));
#54139=CARTESIAN_POINT('Ctrl Pts',(-7.21705230964,-35.4316688958,2.19555083028));
#54140=CARTESIAN_POINT('Ctrl Pts',(-7.21384189759,-35.4651151528,2.18958432614));
#54141=CARTESIAN_POINT('Ctrl Pts',(-7.18673962782,-35.3208994409,2.15657660598));
#54142=CARTESIAN_POINT('Ctrl Pts',(-7.18679863605,-35.3444227249,2.15079574742));
#54143=CARTESIAN_POINT('Ctrl Pts',(-7.18629633971,-35.3679639778,2.14519357364));
#54144=CARTESIAN_POINT('Ctrl Pts',(-7.18523498451,-35.3915169062,2.13977082956));
#54145=CARTESIAN_POINT('Ctrl Pts',(-7.18361579364,-35.4150756718,2.13452906411));
#54146=CARTESIAN_POINT('Ctrl Pts',(-7.18143896677,-35.4386344375,2.12947072768));
#54147=CARTESIAN_POINT('Ctrl Pts',(-7.16019775778,-35.3488473737,2.08142068745));
#54148=CARTESIAN_POINT('Ctrl Pts',(-7.15961328066171,-35.3598678430844,
2.07926829342153));
#54149=CARTESIAN_POINT('Ctrl Pts',(-7.15902631490073,-35.370880846883,2.07710680880288));
#54150=CARTESIAN_POINT('Ctrl Pts',(-7.15843669056073,-35.3818889651522,
2.07493560863704));
#54151=CARTESIAN_POINT('Ctrl Pts',(-7.15784419952897,-35.3928946462221,
2.07275392853839));
#54152=CARTESIAN_POINT('Ctrl Pts',(-7.15724858875,-35.4039003382,2.07056083977));
#54153=CARTESIAN_POINT('Ctrl Pts',(-7.13973478936,-35.3742392475,2.00655473738));
#54154=CARTESIAN_POINT('Ctrl Pts',(-7.13973478936,-35.3742392475,2.00655473738));
#54155=CARTESIAN_POINT('Ctrl Pts',(-7.13973478936,-35.3742392475,2.00655473738));
#54156=CARTESIAN_POINT('Ctrl Pts',(-7.13973478936,-35.3742392475,2.00655473738));
#54157=CARTESIAN_POINT('Ctrl Pts',(-7.13973478936,-35.3742392475,2.00655473738));
#54158=CARTESIAN_POINT('Ctrl Pts',(-7.13973478936,-35.3742392475,2.00655473738));
#54159=CARTESIAN_POINT('Origin',(-6.33322471801445,-35.4651138830689,2.6634130643161));
#54160=CARTESIAN_POINT('Ctrl Pts',(-7.23545146011,-35.2863120169,2.26690923839));
#54161=CARTESIAN_POINT('Ctrl Pts',(-7.2384543,-35.3245396537,2.25650943661));
#54162=CARTESIAN_POINT('Ctrl Pts',(-7.23974953205,-35.3631494767,2.24702142178));
#54163=CARTESIAN_POINT('Ctrl Pts',(-7.23932727374,-35.4020157716,2.23847939875));
#54164=CARTESIAN_POINT('Ctrl Pts',(-7.23718891826,-35.4410103045,2.23091155076));
#54165=CARTESIAN_POINT('Ctrl Pts',(-7.23334710717,-35.4800048374,2.2243394865));
#54166=CARTESIAN_POINT('Ctrl Pts',(-7.23162479878,-35.288610995,2.25877896783));
#54167=CARTESIAN_POINT('Ctrl Pts',(-7.23442685161,-35.3258445567,2.2487681051));
#54168=CARTESIAN_POINT('Ctrl Pts',(-7.23560643854,-35.3634294381,2.2396106895));
#54169=CARTESIAN_POINT('Ctrl Pts',(-7.2351548746,-35.4012499853,2.23133779585));
#54170=CARTESIAN_POINT('Ctrl Pts',(-7.2330735745,-35.4391883682,2.22397519179));
#54171=CARTESIAN_POINT('Ctrl Pts',(-7.22937402512,-35.477126751,2.21754286118));
#54172=CARTESIAN_POINT('Ctrl Pts',(-7.22786970762,-35.291024056,2.2506285999));
#54173=CARTESIAN_POINT('Ctrl Pts',(-7.23046153941,-35.32723074,2.24098939513));
#54174=CARTESIAN_POINT('Ctrl Pts',(-7.23151609908,-35.3637591309,2.23214656382));
#54175=CARTESIAN_POINT('Ctrl Pts',(-7.23102584019,-35.4005032431,2.22412829997));
#54176=CARTESIAN_POINT('Ctrl Pts',(-7.22899220964,-35.437355218,2.21695813089));
#54177=CARTESIAN_POINT('Ctrl Pts',(-7.22542564343,-35.4742071929,2.21065452768));
#54178=CARTESIAN_POINT('Ctrl Pts',(-7.22418450574,-35.2935251725,2.24246594859));
#54179=CARTESIAN_POINT('Ctrl Pts',(-7.22656046023,-35.328675405,2.23318153594));
#54180=CARTESIAN_POINT('Ctrl Pts',(-7.22748386956,-35.3641192075,2.22463810729));
#54181=CARTESIAN_POINT('Ctrl Pts',(-7.22694822371,-35.3997598036,2.21686121842));
#54182=CARTESIAN_POINT('Ctrl Pts',(-7.22495501199,-35.4354987894,2.20987233634));
#54183=CARTESIAN_POINT('Ctrl Pts',(-7.22151371785,-35.4712377752,2.20368850558));
#54184=CARTESIAN_POINT('Ctrl Pts',(-7.22057030307,-35.2960900286,2.23430349206));
#54185=CARTESIAN_POINT('Ctrl Pts',(-7.22272782881,-35.3301573964,2.22535702652));
#54186=CARTESIAN_POINT('Ctrl Pts',(-7.22351653394,-35.364491827,2.21709818648));
#54187=CARTESIAN_POINT('Ctrl Pts',(-7.22293085753,-35.3990052196,2.20955010655));
#54188=CARTESIAN_POINT('Ctrl Pts',(-7.22097232999,-35.4336080936,2.20273236154));
#54189=CARTESIAN_POINT('Ctrl Pts',(-7.21764954964,-35.4682109676,2.19666066586));
#54190=CARTESIAN_POINT('Ctrl Pts',(-7.21702826363,-35.2986939836,2.22615331206));
#54191=CARTESIAN_POINT('Ctrl Pts',(-7.21896725362,-35.3316545144,2.21752775213));
#54192=CARTESIAN_POINT('Ctrl Pts',(-7.21961969567,-35.3648573041,2.20953871906));
#54193=CARTESIAN_POINT('Ctrl Pts',(-7.21898088241,-35.3982223851,2.20220714146));
#54194=CARTESIAN_POINT('Ctrl Pts',(-7.21705236747,-35.4316686126,2.19555084997));
#54195=CARTESIAN_POINT('Ctrl Pts',(-7.2138419429,-35.46511484,2.18958431883));
#54196=CARTESIAN_POINT('Origin',(-6.37002476138651,-35.4800021287416,2.72899290183013));
#54197=CARTESIAN_POINT('Ctrl Pts',(-8.60091079918,-35.1203221982,2.60032832802));
#54198=CARTESIAN_POINT('Ctrl Pts',(-8.55250196755,-35.2208633974,2.5457337616));
#54199=CARTESIAN_POINT('Ctrl Pts',(-8.51670667214,-35.3325773527,2.50053052804));
#54200=CARTESIAN_POINT('Ctrl Pts',(-8.49508712358,-35.4522342996,2.46647854203));
#54201=CARTESIAN_POINT('Ctrl Pts',(-8.48835988758,-35.5758682873,2.44470643423));
#54202=CARTESIAN_POINT('Ctrl Pts',(-8.49626487495,-35.6995022751,2.43550520334));
#54203=CARTESIAN_POINT('Ctrl Pts',(-8.56160117875,-35.1140346808,2.66060541831));
#54204=CARTESIAN_POINT('Ctrl Pts',(-8.51158038352,-35.2164638336,2.60178050099));
#54205=CARTESIAN_POINT('Ctrl Pts',(-8.47440952478,-35.3311106273,2.55334779448));
#54206=CARTESIAN_POINT('Ctrl Pts',(-8.45180416694,-35.454476252,2.51731779839));
#54207=CARTESIAN_POINT('Ctrl Pts',(-8.44456120074,-35.5822080931,2.49495976327));
#54208=CARTESIAN_POINT('Ctrl Pts',(-8.45240512852,-35.7099399342,2.48655698047));
#54209=CARTESIAN_POINT('Ctrl Pts',(-8.51829161967,-35.1086508497,2.71924356476));
#54210=CARTESIAN_POINT('Ctrl Pts',(-8.4676782837,-35.2126508331,2.65547482048));
#54211=CARTESIAN_POINT('Ctrl Pts',(-8.42997337302,-35.3299187074,2.6031885652));
#54212=CARTESIAN_POINT('Ctrl Pts',(-8.40701812301,-35.4566921944,2.56468900549));
#54213=CARTESIAN_POINT('Ctrl Pts',(-8.39967272263,-35.5882267707,2.5414121675));
#54214=CARTESIAN_POINT('Ctrl Pts',(-8.40764108873,-35.7197613468,2.53363446576));
#54215=CARTESIAN_POINT('Ctrl Pts',(-8.47165311425,-35.1035435988,2.77475885702));
#54216=CARTESIAN_POINT('Ctrl Pts',(-8.42103112523,-35.2090000749,2.7055559059));
#54217=CARTESIAN_POINT('Ctrl Pts',(-8.38318247508,-35.3288584812,2.64914965253));
#54218=CARTESIAN_POINT('Ctrl Pts',(-8.36006509714,-35.4590804193,2.60819117966));
#54219=CARTESIAN_POINT('Ctrl Pts',(-8.35259991719,-35.5944943118,2.58430328363));
#54220=CARTESIAN_POINT('Ctrl Pts',(-8.36047222003,-35.7299082045,2.5777319381));
#54221=CARTESIAN_POINT('Ctrl Pts',(-8.35159188251,-35.0922845623,2.89275323394));
#54222=CARTESIAN_POINT('Ctrl Pts',(-8.3050322624,-35.2005432762,2.80975608337));
#54223=CARTESIAN_POINT('Ctrl Pts',(-8.26959869952,-35.3257180408,2.7430273545));
#54224=CARTESIAN_POINT('Ctrl Pts',(-8.2473160419,-35.4631716043,2.69610840641));
#54225=CARTESIAN_POINT('Ctrl Pts',(-8.23918506507,-35.6067794199,2.67107903223));
#54226=CARTESIAN_POINT('Ctrl Pts',(-8.24494252704,-35.7503872354,2.66806485365));
#54227=CARTESIAN_POINT('Ctrl Pts',(-8.20219946581,-35.0869079403,2.96964215712));
#54228=CARTESIAN_POINT('Ctrl Pts',(-8.17044511261,-35.196070615,2.87494321335));
#54229=CARTESIAN_POINT('Ctrl Pts',(-8.14524485361,-35.3234854768,2.79971065515));
#54230=CARTESIAN_POINT('Ctrl Pts',(-8.12806473503,-35.4642227883,2.74824760952));
#54231=CARTESIAN_POINT('Ctrl Pts',(-8.11972374517,-35.6116396625,2.72298240153));
#54232=CARTESIAN_POINT('Ctrl Pts',(-8.12018530542,-35.7590565367,2.723855906));
#54233=CARTESIAN_POINT('Ctrl Pts',(-8.10597427981,-35.0887550559,2.98941073315));
#54234=CARTESIAN_POINT('Ctrl Pts',(-8.08828816032,-35.1976252196,2.89277147723));
#54235=CARTESIAN_POINT('Ctrl Pts',(-8.07262669454,-35.3241767484,2.81647388405));
#54236=CARTESIAN_POINT('Ctrl Pts',(-8.05970660483,-35.4635970156,2.76481016119));
#54237=CARTESIAN_POINT('Ctrl Pts',(-8.05010223161,-35.6094680649,2.74015988873));
#54238=CARTESIAN_POINT('Ctrl Pts',(-8.0441099093,-35.7553391142,2.74240669266));
#54239=CARTESIAN_POINT('Ctrl Pts',(-7.82075728158,-35.1140008873,2.95981413055));
#54240=CARTESIAN_POINT('Ctrl Pts',(-7.83753302833,-35.2174511648,2.88177682176));
#54241=CARTESIAN_POINT('Ctrl Pts',(-7.84624727736,-35.3324220766,2.81978760483));
#54242=CARTESIAN_POINT('Ctrl Pts',(-7.84611816579,-35.4555224941,2.77624706117));
#54243=CARTESIAN_POINT('Ctrl Pts',(-7.83704746541,-35.5826911821,2.75255272839));
#54244=CARTESIAN_POINT('Ctrl Pts',(-7.81966214074,-35.7098598702,2.74888110871));
#54245=CARTESIAN_POINT('Ctrl Pts',(-7.56538653659,-35.1573736159,2.76989788484));
#54246=CARTESIAN_POINT('Ctrl Pts',(-7.58792144694,-35.2456787757,2.72783328434));
#54247=CARTESIAN_POINT('Ctrl Pts',(-7.60265321273,-35.3389337113,2.69350582125));
#54248=CARTESIAN_POINT('Ctrl Pts',(-7.60913119693,-35.4355529064,2.66745188002));
#54249=CARTESIAN_POINT('Ctrl Pts',(-7.60718914349,-35.5338539365,2.65003275892));
#54250=CARTESIAN_POINT('Ctrl Pts',(-7.59696106493,-35.6321549665,2.64143245401));
#54251=CARTESIAN_POINT('Ctrl Pts',(-7.43180190579,-35.1865123729,2.62065670169));
#54252=CARTESIAN_POINT('Ctrl Pts',(-7.44817986306,-35.2646063876,2.59073345827));
#54253=CARTESIAN_POINT('Ctrl Pts',(-7.45830517498,-35.3457624596,2.56600593478));
#54254=CARTESIAN_POINT('Ctrl Pts',(-7.46204607379,-35.4290060284,2.5468488602));
#54255=CARTESIAN_POINT('Ctrl Pts',(-7.45940380717,-35.5132946093,2.53351481199));
#54256=CARTESIAN_POINT('Ctrl Pts',(-7.45050807009,-35.5975831903,2.52611015512));
#54257=CARTESIAN_POINT('Ctrl Pts',(-7.32065041948,-35.231204862,2.4495725015));
#54258=CARTESIAN_POINT('Ctrl Pts',(-7.32870713782,-35.2926200315,2.43080253154));
#54259=CARTESIAN_POINT('Ctrl Pts',(-7.33308472128,-35.3551340146,2.41429805269));
#54260=CARTESIAN_POINT('Ctrl Pts',(-7.33374284515,-35.4183882264,2.40016471574));
#54261=CARTESIAN_POINT('Ctrl Pts',(-7.33068095224,-35.4820120082,2.3884845177));
#54262=CARTESIAN_POINT('Ctrl Pts',(-7.3239386903,-35.5456357901,2.37931366962));
#54263=CARTESIAN_POINT('Ctrl Pts',(-7.23545016815,-35.2863172732,2.26690461593));
#54264=CARTESIAN_POINT('Ctrl Pts',(-7.23845227406,-35.3245433701,2.25650461508));
#54265=CARTESIAN_POINT('Ctrl Pts',(-7.23974688842,-35.3631516089,2.24701631825));
#54266=CARTESIAN_POINT('Ctrl Pts',(-7.23932413184,-35.4020162898,2.23847392839));
#54267=CARTESIAN_POINT('Ctrl Pts',(-7.23718539906,-35.4410091937,2.23090562784));
#54268=CARTESIAN_POINT('Ctrl Pts',(-7.23334333153,-35.4800020975,2.22433302544));
#54269=CARTESIAN_POINT('Origin',(-9.25479694586426,-35.6995103355176,3.08717878194488));
#54270=CARTESIAN_POINT('Ctrl Pts',(-8.82321783753,-35.1473399652,2.21902634713));
#54271=CARTESIAN_POINT('Ctrl Pts',(-8.78215068074,-35.2382758927,2.18429700681));
#54272=CARTESIAN_POINT('Ctrl Pts',(-8.75159630524,-35.3362200688,2.15548691366));
#54273=CARTESIAN_POINT('Ctrl Pts',(-8.73251216058,-35.4390587483,2.13340513227));
#54274=CARTESIAN_POINT('Ctrl Pts',(-8.72535205902,-35.5443464741,2.11857675734));
#54275=CARTESIAN_POINT('Ctrl Pts',(-8.73000528472,-35.6496341999,2.11117245845));
#54276=CARTESIAN_POINT('Ctrl Pts',(-8.7950132494,-35.1439026605,2.27318832802));
#54277=CARTESIAN_POINT('Ctrl Pts',(-8.75278762749,-35.2361296908,2.23654747651));
#54278=CARTESIAN_POINT('Ctrl Pts',(-8.72137526051,-35.3357860213,2.20615712169));
#54279=CARTESIAN_POINT('Ctrl Pts',(-8.70180041036,-35.4406403454,2.18290446914));
#54280=CARTESIAN_POINT('Ctrl Pts',(-8.69454777529,-35.548095721,2.16736469093));
#54281=CARTESIAN_POINT('Ctrl Pts',(-8.69949502688,-35.6555510966,2.15972094562));
#54282=CARTESIAN_POINT('Ctrl Pts',(-8.76584958693,-35.140386513,2.32745356943));
#54283=CARTESIAN_POINT('Ctrl Pts',(-8.72246681666,-35.2339199765,2.28869203429));
#54284=CARTESIAN_POINT('Ctrl Pts',(-8.69020329348,-35.3353435452,2.25654623894));
#54285=CARTESIAN_POINT('Ctrl Pts',(-8.67015581074,-35.4422984936,2.23199348318));
#54286=CARTESIAN_POINT('Ctrl Pts',(-8.66284221447,-35.5520214947,2.21566670729));
#54287=CARTESIAN_POINT('Ctrl Pts',(-8.66812648429,-35.6617444959,2.20776307897));
#54288=CARTESIAN_POINT('Ctrl Pts',(-8.7356657971,-35.1367480171,2.38172554964));
#54289=CARTESIAN_POINT('Ctrl Pts',(-8.69113780582,-35.2316121539,2.34057114953));
#54290=CARTESIAN_POINT('Ctrl Pts',(-8.65803763705,-35.3348781572,2.30644499517));
#54291=CARTESIAN_POINT('Ctrl Pts',(-8.63754180367,-35.4440469154,2.28042962134));
#54292=CARTESIAN_POINT('Ctrl Pts',(-8.63020353714,-35.5561701517,2.26322602866));
#54293=CARTESIAN_POINT('Ctrl Pts',(-8.63587110442,-35.668293388,2.25504712403));
#54294=CARTESIAN_POINT('Ctrl Pts',(-8.69114735744,-35.1314764865,2.45847308227));
#54295=CARTESIAN_POINT('Ctrl Pts',(-8.64510845073,-35.2282535188,2.41340322951));
#54296=CARTESIAN_POINT('Ctrl Pts',(-8.61094346222,-35.3342411346,2.37601936382));
#54297=CARTESIAN_POINT('Ctrl Pts',(-8.58994905716,-35.4467225347,2.34758564448));
#54298=CARTESIAN_POINT('Ctrl Pts',(-8.58273119234,-35.5624541016,2.32891916373));
#54299=CARTESIAN_POINT('Ctrl Pts',(-8.58910725848,-35.6781856686,2.32025995821));
#54300=CARTESIAN_POINT('Ctrl Pts',(-8.64411242258,-35.1256902423,2.53413655954));
#54301=CARTESIAN_POINT('Ctrl Pts',(-8.59671994041,-35.2244531785,2.48429647903));
#54302=CARTESIAN_POINT('Ctrl Pts',(-8.56161211733,-35.333412859,2.44298795985));
#54303=CARTESIAN_POINT('Ctrl Pts',(-8.54022333506,-35.4495924912,2.41171677405));
#54304=CARTESIAN_POINT('Ctrl Pts',(-8.53321738738,-35.5693865938,2.39145291764));
#54305=CARTESIAN_POINT('Ctrl Pts',(-8.54037362589,-35.6891806965,2.38246370607));
#54306=CARTESIAN_POINT('Ctrl Pts',(-8.62993676763,-35.1239763388,2.55637951988));
#54307=CARTESIAN_POINT('Ctrl Pts',(-8.58219189761,-35.2233231665,2.50503392418));
#54308=CARTESIAN_POINT('Ctrl Pts',(-8.54685013234,-35.3331714269,2.46248222847));
#54309=CARTESIAN_POINT('Ctrl Pts',(-8.52538633662,-35.4504650834,2.43030855578));
#54310=CARTESIAN_POINT('Ctrl Pts',(-8.51848133158,-35.5714859455,2.4095318701));
#54311=CARTESIAN_POINT('Ctrl Pts',(-8.52590127043,-35.6925068075,2.40042817508));
#54312=CARTESIAN_POINT('Ctrl Pts',(-8.61560772534,-35.1221440943,2.57842131078));
#54313=CARTESIAN_POINT('Ctrl Pts',(-8.56749228928,-35.2220926432,2.52550930797));
#54314=CARTESIAN_POINT('Ctrl Pts',(-8.53188890827,-35.3328708509,2.48168265536));
#54315=CARTESIAN_POINT('Ctrl Pts',(-8.5103168202,-35.4513369446,2.44860878814));
#54316=CARTESIAN_POINT('Ctrl Pts',(-8.50347493534,-35.5736522798,2.42735915225));
#54317=CARTESIAN_POINT('Ctrl Pts',(-8.51111753906,-35.695967615,2.41821700034));
#54318=CARTESIAN_POINT('Ctrl Pts',(-8.60091081429,-35.1203221009,2.60032838611));
#54319=CARTESIAN_POINT('Ctrl Pts',(-8.55250194661,-35.2208633123,2.54573382886));
#54320=CARTESIAN_POINT('Ctrl Pts',(-8.51670661225,-35.3325772847,2.50053061213));
#54321=CARTESIAN_POINT('Ctrl Pts',(-8.49508702343,-35.4522342523,2.46647865078));
#54322=CARTESIAN_POINT('Ctrl Pts',(-8.4883597474,-35.5758682626,2.44470657499));
#54323=CARTESIAN_POINT('Ctrl Pts',(-8.49626469614,-35.699502273,2.4355053823));
#54324=CARTESIAN_POINT('Origin',(-9.57674350374405,-35.6496306966926,2.64320593658555));
#54325=CARTESIAN_POINT('Ctrl Pts',(-8.84972761074,-35.1509187546,2.16704276679));
#54326=CARTESIAN_POINT('Ctrl Pts',(-8.80995141052,-35.2405485577,2.13393459289));
#54327=CARTESIAN_POINT('Ctrl Pts',(-8.78039709025,-35.3367789605,2.10641485522));
#54328=CARTESIAN_POINT('Ctrl Pts',(-8.7619545083,-35.4376105338,2.08522367244));
#54329=CARTESIAN_POINT('Ctrl Pts',(-8.75504416849,-35.5407442468,2.0708442184));
#54330=CARTESIAN_POINT('Ctrl Pts',(-8.75956299023,-35.6438779598,2.0634404101));
#54331=CARTESIAN_POINT('Ctrl Pts',(-8.84456885861,-35.1501669799,2.17736664036));
#54332=CARTESIAN_POINT('Ctrl Pts',(-8.80450316343,-35.2400691335,2.14397755154));
#54333=CARTESIAN_POINT('Ctrl Pts',(-8.77471769299,-35.3366533562,2.11624485706));
#54334=CARTESIAN_POINT('Ctrl Pts',(-8.75611631291,-35.437897274,2.0949212219));
#54335=CARTESIAN_POINT('Ctrl Pts',(-8.74912677261,-35.5414726393,2.08049700356));
#54336=CARTESIAN_POINT('Ctrl Pts',(-8.75364509765,-35.6450480046,2.07313650893));
#54337=CARTESIAN_POINT('Ctrl Pts',(-8.83934134903,-35.1494257084,2.1877279664));
#54338=CARTESIAN_POINT('Ctrl Pts',(-8.79900028815,-35.2395949404,2.15403728116));
#54339=CARTESIAN_POINT('Ctrl Pts',(-8.76899769743,-35.3365278505,2.12607022447));
#54340=CARTESIAN_POINT('Ctrl Pts',(-8.75025126803,-35.4381791278,2.10459258862));
#54341=CARTESIAN_POINT('Ctrl Pts',(-8.74319574656,-35.5421912387,2.09010248095));
#54342=CARTESIAN_POINT('Ctrl Pts',(-8.74772599292,-35.6462033496,2.08276502103));
#54343=CARTESIAN_POINT('Ctrl Pts',(-8.83403961773,-35.1487041475,2.19812825065));
#54344=CARTESIAN_POINT('Ctrl Pts',(-8.79343976066,-35.2391345884,2.16411346789));
#54345=CARTESIAN_POINT('Ctrl Pts',(-8.76323651939,-35.3364102747,2.1358885387));
#54346=CARTESIAN_POINT('Ctrl Pts',(-8.74436113276,-35.4384630225,2.11423302609));
#54347=CARTESIAN_POINT('Ctrl Pts',(-8.73725504684,-35.5429059973,2.0996533862));
#54348=CARTESIAN_POINT('Ctrl Pts',(-8.74181161845,-35.6473489721,2.09231606717));
#54349=CARTESIAN_POINT('Ctrl Pts',(-8.82866432718,-35.1480081194,2.20856250217));
#54350=CARTESIAN_POINT('Ctrl Pts',(-8.78782272692,-35.2386939519,2.17420118315));
#54351=CARTESIAN_POINT('Ctrl Pts',(-8.75743582295,-35.3363065177,2.14569487681));
#54352=CARTESIAN_POINT('Ctrl Pts',(-8.73844810187,-35.4387548314,2.12383756828));
#54353=CARTESIAN_POINT('Ctrl Pts',(-8.73130736324,-35.5436227636,2.10914471028));
#54354=CARTESIAN_POINT('Ctrl Pts',(-8.73590510583,-35.6484906957,2.1017846051));
#54355=CARTESIAN_POINT('Ctrl Pts',(-8.82321744436,-35.1473421125,2.21902489656));
#54356=CARTESIAN_POINT('Ctrl Pts',(-8.78215104537,-35.2382777414,2.18429511356));
#54357=CARTESIAN_POINT('Ctrl Pts',(-8.75159740651,-35.3362215383,2.15548447298));
#54358=CARTESIAN_POINT('Ctrl Pts',(-8.73251395256,-35.4390597803,2.13340204369));
#54359=CARTESIAN_POINT('Ctrl Pts',(-8.72535447592,-35.5443470397,2.11857293178));
#54360=CARTESIAN_POINT('Ctrl Pts',(-8.73000824887,-35.6496342991,2.1111678244));
#54361=CARTESIAN_POINT('Origin',(-9.61320752990433,-35.6438714700362,2.58431858586112));
#54362=CARTESIAN_POINT('Ctrl Pts',(-8.84973117353,-35.1509193731,2.1670354781));
#54363=CARTESIAN_POINT('Ctrl Pts',(-8.80995437067,-35.2405490067,2.13392896451));
#54364=CARTESIAN_POINT('Ctrl Pts',(-8.78039938016,-35.3367791654,2.10641082417));
#54365=CARTESIAN_POINT('Ctrl Pts',(-8.76195606614,-35.4376104406,2.08522113231));
#54366=CARTESIAN_POINT('Ctrl Pts',(-8.75504494547,-35.5407438285,2.07084302459));
#54367=CARTESIAN_POINT('Ctrl Pts',(-8.75956295656,-35.6438772164,2.06344039042));
#54368=CARTESIAN_POINT('Ctrl Pts',(-8.91091202313,-35.1598372898,2.04459467569));
#54369=CARTESIAN_POINT('Ctrl Pts',(-8.87455647002,-35.246237181,2.01484191076));
#54370=CARTESIAN_POINT('Ctrl Pts',(-8.84773035639,-35.3382711138,1.98987130618));
#54371=CARTESIAN_POINT('Ctrl Pts',(-8.83115765576,-35.4342118768,1.97027362582));
#54372=CARTESIAN_POINT('Ctrl Pts',(-8.82517322934,-35.532107067,1.95644630565));
#54373=CARTESIAN_POINT('Ctrl Pts',(-8.82968488575,-35.6300022572,1.94854820039));
#54374=CARTESIAN_POINT('Ctrl Pts',(-8.96795816735,-35.1710296589,1.91634945111));
#54375=CARTESIAN_POINT('Ctrl Pts',(-8.93494048323,-35.2532459987,1.89161496085));
#54376=CARTESIAN_POINT('Ctrl Pts',(-8.91060835461,-35.3400086156,1.87063336475));
#54377=CARTESIAN_POINT('Ctrl Pts',(-8.89552405555,-35.4299031373,1.85381398232));
#54378=CARTESIAN_POINT('Ctrl Pts',(-8.88994864311,-35.5213641494,1.84144178963));
#54379=CARTESIAN_POINT('Ctrl Pts',(-8.89381707546,-35.6128251616,1.83365112687));
#54380=CARTESIAN_POINT('Ctrl Pts',(-9.01653709076,-35.1835781664,1.78332507658));
#54381=CARTESIAN_POINT('Ctrl Pts',(-8.98711360766,-35.260897748,1.76325201128));
#54382=CARTESIAN_POINT('Ctrl Pts',(-8.96538998881,-35.341846639,1.74604152846));
#54383=CARTESIAN_POINT('Ctrl Pts',(-8.95179602076,-35.4252853121,1.73198094156));
#54384=CARTESIAN_POINT('Ctrl Pts',(-8.94653331601,-35.5099692034,1.72127486801));
#54385=CARTESIAN_POINT('Ctrl Pts',(-8.9495584777,-35.5946530947,1.71402843838));
#54386=CARTESIAN_POINT('Ctrl Pts',(-9.1140028877,-35.2108461818,1.46157810716));
#54387=CARTESIAN_POINT('Ctrl Pts',(-9.09197113076,-35.2771127336,1.45066936239));
#54388=CARTESIAN_POINT('Ctrl Pts',(-9.07556758896,-35.3453927996,1.44108450365));
#54389=CARTESIAN_POINT('Ctrl Pts',(-9.06500040952,-35.4150382685,1.43291495679));
#54390=CARTESIAN_POINT('Ctrl Pts',(-9.06037122564,-35.4853665076,1.42623124853));
#54391=CARTESIAN_POINT('Ctrl Pts',(-9.06167021042,-35.5556947466,1.4210802448));
#54392=CARTESIAN_POINT('Ctrl Pts',(-9.17852891179,-35.2281865303,1.13254165139));
#54393=CARTESIAN_POINT('Ctrl Pts',(-9.16069403398,-35.2869558429,1.12639249526));
#54394=CARTESIAN_POINT('Ctrl Pts',(-9.14729128577,-35.3471459486,1.12104732689));
#54395=CARTESIAN_POINT('Ctrl Pts',(-9.13845933491,-35.4082985485,1.1165532711));
#54396=CARTESIAN_POINT('Ctrl Pts',(-9.13426752236,-35.4699324162,1.11294417189));
#54397=CARTESIAN_POINT('Ctrl Pts',(-9.13471251897,-35.531566284,1.1102388653));
#54398=CARTESIAN_POINT('Ctrl Pts',(-9.20897519651,-35.2324135956,0.943972367435));
#54399=CARTESIAN_POINT('Ctrl Pts',(-9.19209813045,-35.2892087111,0.939475719579));
#54400=CARTESIAN_POINT('Ctrl Pts',(-9.17938477515,-35.3472963111,0.935686471687));
#54401=CARTESIAN_POINT('Ctrl Pts',(-9.1709591607,-35.4062580486,0.93263706468));
#54402=CARTESIAN_POINT('Ctrl Pts',(-9.16688368582,-35.4656570006,0.930349922162));
#54403=CARTESIAN_POINT('Ctrl Pts',(-9.1671566108,-35.5250559527,0.928836133483));
#54404=CARTESIAN_POINT('Ctrl Pts',(-9.23916608575,-35.2348774759,0.761379139513));
#54405=CARTESIAN_POINT('Ctrl Pts',(-9.22290027765,-35.2906450094,0.757499573794));
#54406=CARTESIAN_POINT('Ctrl Pts',(-9.21063507987,-35.3476242625,0.754282164424));
#54407=CARTESIAN_POINT('Ctrl Pts',(-9.20248495391,-35.4054228352,0.75175437252));
#54408=CARTESIAN_POINT('Ctrl Pts',(-9.19850755669,-35.4636310173,0.749934120027));
#54409=CARTESIAN_POINT('Ctrl Pts',(-9.19870123297,-35.5218391995,0.748829315604));
#54410=CARTESIAN_POINT('Ctrl Pts',(-9.26569123725,-35.2394333704,0.579580156823));
#54411=CARTESIAN_POINT('Ctrl Pts',(-9.25048972376,-35.2934591001,0.575764245003));
#54412=CARTESIAN_POINT('Ctrl Pts',(-9.23904456924,-35.3485824305,0.57252390595));
#54413=CARTESIAN_POINT('Ctrl Pts',(-9.2314560575,-35.4044472049,0.569884306758));
#54414=CARTESIAN_POINT('Ctrl Pts',(-9.22777454338,-35.4606827234,0.567862962924));
#54415=CARTESIAN_POINT('Ctrl Pts',(-9.22799848318,-35.5169182418,0.566469053265));
#54416=CARTESIAN_POINT('Origin',(-10.2153564537533,-35.5169155168785,0.724979907680837));
#54417=CARTESIAN_POINT('Ctrl Pts',(-9.26569107955,-35.2394341184,0.579579770152));
#54418=CARTESIAN_POINT('Ctrl Pts',(-9.25048970237,-35.2934597015,0.575763550708));
#54419=CARTESIAN_POINT('Ctrl Pts',(-9.23904466522,-35.3485828761,0.57252289393));
#54420=CARTESIAN_POINT('Ctrl Pts',(-9.23145625045,-35.4044474883,0.569882968796));
#54421=CARTESIAN_POINT('Ctrl Pts',(-9.22777481195,-35.4606828414,0.567861292872));
#54422=CARTESIAN_POINT('Ctrl Pts',(-9.22799880569,-35.5169181946,0.566467047136));
#54423=CARTESIAN_POINT('Ctrl Pts',(-9.26734254057,-35.2397154298,0.568265288566));
#54424=CARTESIAN_POINT('Ctrl Pts',(-9.25220700276,-35.2936330337,0.564453943744));
#54425=CARTESIAN_POINT('Ctrl Pts',(-9.24081265384,-35.3486411511,0.561212799914));
#54426=CARTESIAN_POINT('Ctrl Pts',(-9.23325890658,-35.4043858824,0.558566884261));
#54427=CARTESIAN_POINT('Ctrl Pts',(-9.22959566517,-35.4604989426,0.556533678149));
#54428=CARTESIAN_POINT('Ctrl Pts',(-9.22982138229,-35.5166120028,0.55512243494));
#54429=CARTESIAN_POINT('Ctrl Pts',(-9.26898307793,-35.2399973473,0.556947742073));
#54430=CARTESIAN_POINT('Ctrl Pts',(-9.25391368938,-35.2938057049,0.55314265644));
#54431=CARTESIAN_POINT('Ctrl Pts',(-9.24257020144,-35.3486974567,0.549902346095));
#54432=CARTESIAN_POINT('Ctrl Pts',(-9.23505116442,-35.4043209585,0.547251660046));
#54433=CARTESIAN_POINT('Ctrl Pts',(-9.23140601814,-35.4603103757,0.54520808798));
#54434=CARTESIAN_POINT('Ctrl Pts',(-9.23163322063,-35.516299793,0.543780919912));
#54435=CARTESIAN_POINT('Ctrl Pts',(-9.2706134925,-35.2402652369,0.545649357377));
#54436=CARTESIAN_POINT('Ctrl Pts',(-9.25560999309,-35.2939662109,0.541842800001));
#54437=CARTESIAN_POINT('Ctrl Pts',(-9.24431742891,-35.3487436319,0.53859575027));
#54438=CARTESIAN_POINT('Ctrl Pts',(-9.23683343793,-35.4042480754,0.535933346844));
#54439=CARTESIAN_POINT('Ctrl Pts',(-9.23320713925,-35.460116063,0.533872309581));
#54440=CARTESIAN_POINT('Ctrl Pts',(-9.23343691736,-35.5159840505,0.532422414623));
#54441=CARTESIAN_POINT('Ctrl Pts',(-9.2722446143,-35.2405353461,0.534265835364));
#54442=CARTESIAN_POINT('Ctrl Pts',(-9.25730181761,-35.294127701,0.530496224362));
#54443=CARTESIAN_POINT('Ctrl Pts',(-9.24605472348,-35.3487894773,0.527280786202));
#54444=CARTESIAN_POINT('Ctrl Pts',(-9.2386001998,-35.4041734976,0.524643949807));
#54445=CARTESIAN_POINT('Ctrl Pts',(-9.23498684878,-35.4599186602,0.522602910424));
#54446=CARTESIAN_POINT('Ctrl Pts',(-9.23521314025,-35.5156638228,0.521166956934));
#54447=CARTESIAN_POINT('Ctrl Pts',(-9.27386188355,-35.2408046483,0.522899878387));
#54448=CARTESIAN_POINT('Ctrl Pts',(-9.25898070438,-35.2942887003,0.519158423034));
#54449=CARTESIAN_POINT('Ctrl Pts',(-9.24778011027,-35.34883522,0.515965854318));
#54450=CARTESIAN_POINT('Ctrl Pts',(-9.24035614735,-35.4040992464,0.513346314134));
#54451=CARTESIAN_POINT('Ctrl Pts',(-9.23675700648,-35.4597220466,0.511316806589));
#54452=CARTESIAN_POINT('Ctrl Pts',(-9.23698117862,-35.5153448469,0.509886547139));
#54453=CARTESIAN_POINT('Origin',(-10.224921002496,-35.5153449894579,0.664731520865732));
#54454=CARTESIAN_POINT('Ctrl Pts',(-9.01911953995,-35.2680044421,-3.13244837682));
#54455=CARTESIAN_POINT('Ctrl Pts',(-9.01128290018,-35.3096899679,-3.12777753845));
#54456=CARTESIAN_POINT('Ctrl Pts',(-9.00550173203,-35.3518572367,-3.12395745117));
#54457=CARTESIAN_POINT('Ctrl Pts',(-9.00180577632,-35.3943481132,-3.12100583911));
#54458=CARTESIAN_POINT('Ctrl Pts',(-9.00020910686,-35.4370007968,-3.11893394172));
#54459=CARTESIAN_POINT('Ctrl Pts',(-9.00070981215,-35.4796534803,-3.1177462595));
#54460=CARTESIAN_POINT('Ctrl Pts',(-9.17544595344,-35.2835018925,-2.74597776201));
#54461=CARTESIAN_POINT('Ctrl Pts',(-9.16933554333,-35.3193494556,-2.74372235315));
#54462=CARTESIAN_POINT('Ctrl Pts',(-9.16476148349,-35.3554672008,-2.74189804713));
#54463=CARTESIAN_POINT('Ctrl Pts',(-9.1617381998,-35.3917657165,-2.74050818076));
#54464=CARTESIAN_POINT('Ctrl Pts',(-9.1602730438,-35.428154617,-2.73955472374));
#54465=CARTESIAN_POINT('Ctrl Pts',(-9.16036621938,-35.4645435174,-2.73903830807));
#54466=CARTESIAN_POINT('Ctrl Pts',(-9.29269126807,-35.2907452551,-2.34477529883));
#54467=CARTESIAN_POINT('Ctrl Pts',(-9.28707239127,-35.3238061129,-2.34352966982));
#54468=CARTESIAN_POINT('Ctrl Pts',(-9.282834933,-35.3571174391,-2.34257541991));
#54469=CARTESIAN_POINT('Ctrl Pts',(-9.27999356004,-35.3905967652,-2.34191674071));
#54470=CARTESIAN_POINT('Ctrl Pts',(-9.27855558309,-35.424160093,-2.3415559411));
#54471=CARTESIAN_POINT('Ctrl Pts',(-9.27852082014,-35.4577234207,-2.34149337034));
#54472=CARTESIAN_POINT('Ctrl Pts',(-9.36191429928,-35.2893802972,-1.92981468559));
#54473=CARTESIAN_POINT('Ctrl Pts',(-9.3560452611,-35.3232454878,-1.92921642136));
#54474=CARTESIAN_POINT('Ctrl Pts',(-9.35161541947,-35.3573586818,-1.92882344418));
#54475=CARTESIAN_POINT('Ctrl Pts',(-9.34863880943,-35.3916379824,-1.92863719423));
#54476=CARTESIAN_POINT('Ctrl Pts',(-9.3471225791,-35.4260003368,-1.92865812789));
#54477=CARTESIAN_POINT('Ctrl Pts',(-9.3470668903,-35.4603626911,-1.92888572013));
#54478=CARTESIAN_POINT('Ctrl Pts',(-9.4171903904,-35.2789856765,-1.18748239275));
#54479=CARTESIAN_POINT('Ctrl Pts',(-9.40981639515,-35.3169659165,-1.18801696878));
#54480=CARTESIAN_POINT('Ctrl Pts',(-9.40425718706,-35.3552891517,-1.18859518921));
#54481=CARTESIAN_POINT('Ctrl Pts',(-9.40053397643,-35.3938423214,-1.18921641071));
#54482=CARTESIAN_POINT('Ctrl Pts',(-9.39865750897,-35.4325104595,-1.18987939995));
#54483=CARTESIAN_POINT('Ctrl Pts',(-9.39862789646,-35.4711785976,-1.19058233503));
#54484=CARTESIAN_POINT('Ctrl Pts',(-9.38314539193,-35.2631816303,-0.439456405049));
#54485=CARTESIAN_POINT('Ctrl Pts',(-9.37293597078,-35.3077684071,-0.441248963721));
#54486=CARTESIAN_POINT('Ctrl Pts',(-9.36525594777,-35.3529358557,-0.442871125473));
#54487=CARTESIAN_POINT('Ctrl Pts',(-9.36014835673,-35.3984936385,-0.444315444411));
#54488=CARTESIAN_POINT('Ctrl Pts',(-9.35763482817,-35.4442465927,-0.44557584201));
#54489=CARTESIAN_POINT('Ctrl Pts',(-9.3577150604,-35.489999547,-0.446647757649));
#54490=CARTESIAN_POINT('Ctrl Pts',(-9.3558891039,-35.2557890156,-0.116721794816));
#54491=CARTESIAN_POINT('Ctrl Pts',(-9.34426128655,-35.3033050214,-0.118995176137));
#54492=CARTESIAN_POINT('Ctrl Pts',(-9.33551278911,-35.3515333802,-0.120988679218));
#54493=CARTESIAN_POINT('Ctrl Pts',(-9.3296998933,-35.4002411909,-0.122691582222));
#54494=CARTESIAN_POINT('Ctrl Pts',(-9.32685085926,-35.4491887348,-0.124095735733));
#54495=CARTESIAN_POINT('Ctrl Pts',(-9.32696513263,-35.4981362787,-0.12519578818));
#54496=CARTESIAN_POINT('Ctrl Pts',(-9.3192256268,-35.2483585547,0.204089324846));
#54497=CARTESIAN_POINT('Ctrl Pts',(-9.30607279618,-35.2988047548,0.201137625763));
#54498=CARTESIAN_POINT('Ctrl Pts',(-9.29617649939,-35.3501183672,0.198586534665));
#54499=CARTESIAN_POINT('Ctrl Pts',(-9.28960975953,-35.4020166188,0.196452114669));
#54500=CARTESIAN_POINT('Ctrl Pts',(-9.28640921473,-35.4542072015,0.194746107875));
#54501=CARTESIAN_POINT('Ctrl Pts',(-9.28657394094,-35.5063977842,0.193475565417));
#54502=CARTESIAN_POINT('Ctrl Pts',(-9.27386188307,-35.2408046524,0.522899877563));
#54503=CARTESIAN_POINT('Ctrl Pts',(-9.25898070398,-35.2942887044,0.519158422332));
#54504=CARTESIAN_POINT('Ctrl Pts',(-9.24778010992,-35.3488352241,0.515965853737));
#54505=CARTESIAN_POINT('Ctrl Pts',(-9.24035614705,-35.4040992505,0.513346313675));
#54506=CARTESIAN_POINT('Ctrl Pts',(-9.2367570062,-35.4597220507,0.511316806249));
#54507=CARTESIAN_POINT('Ctrl Pts',(-9.23698117834,-35.5153448509,0.509886546917));
#54508=CARTESIAN_POINT('Origin',(-9.92303703930928,-35.4797547933065,-3.50659112139201));
#54509=CARTESIAN_POINT('Ctrl Pts',(-8.93444595596,-35.2748053687,-3.31652394249));
#54510=CARTESIAN_POINT('Ctrl Pts',(-8.92616317166,-35.3147866052,-3.31461891577));
#54511=CARTESIAN_POINT('Ctrl Pts',(-8.91971750036,-35.3551912403,-3.31361234962));
#54512=CARTESIAN_POINT('Ctrl Pts',(-8.91513778092,-35.3958801128,-3.31351087925));
#54513=CARTESIAN_POINT('Ctrl Pts',(-8.91244000919,-35.4367111064,-3.31431485906));
#54514=CARTESIAN_POINT('Ctrl Pts',(-8.91162700591,-35.4775421,-3.31601835533));
#54515=CARTESIAN_POINT('Ctrl Pts',(-8.94734368663,-35.2728133782,-3.29109023634));
#54516=CARTESIAN_POINT('Ctrl Pts',(-8.93895107582,-35.3135017401,-3.28875572575));
#54517=CARTESIAN_POINT('Ctrl Pts',(-8.93246763725,-35.3546364096,-3.28733586636));
#54518=CARTESIAN_POINT('Ctrl Pts',(-8.9279236303,-35.3960707679,-3.28683902656));
#54519=CARTESIAN_POINT('Ctrl Pts',(-8.92533550226,-35.4376549725,-3.28726695529));
#54520=CARTESIAN_POINT('Ctrl Pts',(-8.92470553582,-35.4792391771,-3.28861474271));
#54521=CARTESIAN_POINT('Ctrl Pts',(-8.95983458954,-35.2711079221,-3.26569669172));
#54522=CARTESIAN_POINT('Ctrl Pts',(-8.95141175919,-35.3123562177,-3.2628807422));
#54523=CARTESIAN_POINT('Ctrl Pts',(-8.94495906105,-35.354070024,-3.26098724776));
#54524=CARTESIAN_POINT('Ctrl Pts',(-8.94050773142,-35.3960964758,-3.260026589));
#54525=CARTESIAN_POINT('Ctrl Pts',(-8.93807435022,-35.4382792543,-3.26000227455));
#54526=CARTESIAN_POINT('Ctrl Pts',(-8.93766047318,-35.4804620328,-3.26091086944));
#54527=CARTESIAN_POINT('Ctrl Pts',(-8.97214212604,-35.2697920542,-3.23978066277));
#54528=CARTESIAN_POINT('Ctrl Pts',(-8.9637190734,-35.311417995,-3.23656869462));
#54529=CARTESIAN_POINT('Ctrl Pts',(-8.95731138416,-35.3535230656,-3.23427864864));
#54530=CARTESIAN_POINT('Ctrl Pts',(-8.95295080025,-35.3959499382,-3.2329226531));
#54531=CARTESIAN_POINT('Ctrl Pts',(-8.95065387904,-35.4385377451,-3.23250578662));
#54532=CARTESIAN_POINT('Ctrl Pts',(-8.95042158697,-35.481125552,-3.23302610121));
#54533=CARTESIAN_POINT('Ctrl Pts',(-8.98911618271,-35.268630653,-3.20263013659));
#54534=CARTESIAN_POINT('Ctrl Pts',(-8.98077765617,-35.3105436223,-3.19892614932));
#54535=CARTESIAN_POINT('Ctrl Pts',(-8.97449392264,-35.3529460311,-3.19613159274));
#54536=CARTESIAN_POINT('Ctrl Pts',(-8.97029699893,-35.3956772608,-3.19426066196));
#54537=CARTESIAN_POINT('Ctrl Pts',(-8.96820302947,-35.4385728912,-3.19332056844));
#54538=CARTESIAN_POINT('Ctrl Pts',(-8.96821193143,-35.4814685217,-3.19331131722));
#54539=CARTESIAN_POINT('Ctrl Pts',(-9.00517206358,-35.2680735988,-3.16566118546));
#54540=CARTESIAN_POINT('Ctrl Pts',(-8.99706509175,-35.3099657558,-3.16142494219));
#54541=CARTESIAN_POINT('Ctrl Pts',(-8.99102314624,-35.3523468191,-3.15807110791));
#54542=CARTESIAN_POINT('Ctrl Pts',(-8.98707727301,-35.395056319,-3.15561591639));
#54543=CARTESIAN_POINT('Ctrl Pts',(-8.9852426452,-35.4379300459,-3.15406880151));
#54544=CARTESIAN_POINT('Ctrl Pts',(-8.98551821082,-35.4808037728,-3.15343220651));
#54545=CARTESIAN_POINT('Ctrl Pts',(-9.00990494748,-35.2680166859,-3.15455724964));
#54546=CARTESIAN_POINT('Ctrl Pts',(-9.00187362208,-35.3098646744,-3.1501873274));
#54547=CARTESIAN_POINT('Ctrl Pts',(-8.99590638677,-35.3522000159,-3.14669037035));
#54548=CARTESIAN_POINT('Ctrl Pts',(-8.99203402793,-35.3948627823,-3.14408308561));
#54549=CARTESIAN_POINT('Ctrl Pts',(-8.9902713955,-35.4376892422,-3.1423755103));
#54550=CARTESIAN_POINT('Ctrl Pts',(-8.9906170886,-35.480515702,-3.141570683));
#54551=CARTESIAN_POINT('Ctrl Pts',(-9.01453522232,-35.2679213672,-3.1435714055));
#54552=CARTESIAN_POINT('Ctrl Pts',(-9.00660223792,-35.3097130029,-3.13902110731));
#54553=CARTESIAN_POINT('Ctrl Pts',(-9.00073178209,-35.3519900952,-3.13533334259));
#54554=CARTESIAN_POINT('Ctrl Pts',(-8.99695406159,-35.3945932824,-3.13252547117));
#54555=CARTESIAN_POINT('Ctrl Pts',(-8.99528353801,-35.4373595352,-3.13060822223));
#54556=CARTESIAN_POINT('Ctrl Pts',(-8.99571858313,-35.480125788,-3.12958551692));
#54557=CARTESIAN_POINT('Ctrl Pts',(-9.01911869111,-35.2680072167,-3.13244884091));
#54558=CARTESIAN_POINT('Ctrl Pts',(-9.01128168784,-35.3096922673,-3.12777947274));
#54559=CARTESIAN_POINT('Ctrl Pts',(-9.00550009533,-35.3518590427,-3.12396085378));
#54560=CARTESIAN_POINT('Ctrl Pts',(-9.00180365501,-35.3943494134,-3.12101070215));
#54561=CARTESIAN_POINT('Ctrl Pts',(-9.00020644216,-35.4370015851,-3.1189402514));
#54562=CARTESIAN_POINT('Ctrl Pts',(-9.0007065476,-35.4796537567,-3.11775399652));
#54563=CARTESIAN_POINT('Origin',(-9.81411538991078,-35.4775422485357,-3.74673324846717));
#54564=CARTESIAN_POINT('Ctrl Pts',(-2.02882252548,-35.2583787857,-8.24404394735));
#54565=CARTESIAN_POINT('Ctrl Pts',(-2.02793435434,-35.304849438,-8.23266211897));
#54566=CARTESIAN_POINT('Ctrl Pts',(-2.0275994353,-35.3519981482,-8.22400554803));
#54567=CARTESIAN_POINT('Ctrl Pts',(-2.02782201048,-35.3996032301,-8.21812855721));
#54568=CARTESIAN_POINT('Ctrl Pts',(-2.02860101303,-35.4474365049,-8.21505931587));
#54569=CARTESIAN_POINT('Ctrl Pts',(-2.02993009745,-35.4952697797,-8.21479904026));
#54570=CARTESIAN_POINT('Ctrl Pts',(-2.7603704221,-35.2788135941,-8.09044877058));
#54571=CARTESIAN_POINT('Ctrl Pts',(-2.75916038902,-35.3170950643,-8.08332087145));
#54572=CARTESIAN_POINT('Ctrl Pts',(-2.75848926909,-35.3556762451,-8.07788965412));
#54573=CARTESIAN_POINT('Ctrl Pts',(-2.75836124945,-35.3944575182,-8.07416878882));
#54574=CARTESIAN_POINT('Ctrl Pts',(-2.75877734505,-35.4333388354,-8.07216551353));
#54575=CARTESIAN_POINT('Ctrl Pts',(-2.75973535856,-35.4722201525,-8.07188072536));
#54576=CARTESIAN_POINT('Ctrl Pts',(-3.46770746463,-35.2977417588,-7.8780751558));
#54577=CARTESIAN_POINT('Ctrl Pts',(-3.46660967304,-35.3282659767,-7.87385395784));
#54578=CARTESIAN_POINT('Ctrl Pts',(-3.46593509074,-35.3589261674,-7.87061653092));
#54579=CARTESIAN_POINT('Ctrl Pts',(-3.4656850911,-35.3896774143,-7.8683685806));
#54580=CARTESIAN_POINT('Ctrl Pts',(-3.46586006339,-35.420474191,-7.86711317222));
#54581=CARTESIAN_POINT('Ctrl Pts',(-3.46645942733,-35.4512709677,-7.86685062308));
#54582=CARTESIAN_POINT('Ctrl Pts',(-4.1448564034,-35.31305193,-7.60417987874));
#54583=CARTESIAN_POINT('Ctrl Pts',(-4.14387911843,-35.3375078051,-7.60136146782));
#54584=CARTESIAN_POINT('Ctrl Pts',(-4.14322007764,-35.3620512903,-7.59920530757));
#54585=CARTESIAN_POINT('Ctrl Pts',(-4.14288053918,-35.3866532884,-7.59771461525));
#54586=CARTESIAN_POINT('Ctrl Pts',(-4.14286096901,-35.4112845426,-7.59689108063));
#54587=CARTESIAN_POINT('Ctrl Pts',(-4.14316103429,-35.4359157968,-7.59673486922));
#54588=CARTESIAN_POINT('Ctrl Pts',(-5.21843923371,-35.3262967395,-7.044990155));
#54589=CARTESIAN_POINT('Ctrl Pts',(-5.21754878579,-35.3454147425,-7.04339100369));
#54590=CARTESIAN_POINT('Ctrl Pts',(-5.21690210383,-35.3645740899,-7.04217483695));
#54591=CARTESIAN_POINT('Ctrl Pts',(-5.21649981226,-35.3837610519,-7.04134271025));
#54592=CARTESIAN_POINT('Ctrl Pts',(-5.21634220772,-35.4029618215,-7.04089517538));
#54593=CARTESIAN_POINT('Ctrl Pts',(-5.21642926006,-35.422162591,-7.04083226933));
#54594=CARTESIAN_POINT('Ctrl Pts',(-6.21090480851,-35.3291957718,-6.34191684905));
#54595=CARTESIAN_POINT('Ctrl Pts',(-6.20990218356,-35.347292328,-6.34059495831));
#54596=CARTESIAN_POINT('Ctrl Pts',(-6.20914711064,-35.3654273382,-6.33960321184));
#54597=CARTESIAN_POINT('Ctrl Pts',(-6.20864031997,-35.3835880114,-6.33894257829));
#54598=CARTESIAN_POINT('Ctrl Pts',(-6.20838217516,-35.401761516,-6.33861353938));
#54599=CARTESIAN_POINT('Ctrl Pts',(-6.20837267016,-35.4199350207,-6.33861609384));
#54600=CARTESIAN_POINT('Ctrl Pts',(-6.59524089295,-35.3292320711,-6.04038307893));
#54601=CARTESIAN_POINT('Ctrl Pts',(-6.59420777333,-35.3473355691,-6.03905690773));
#54602=CARTESIAN_POINT('Ctrl Pts',(-6.59343802139,-35.3654739877,-6.03805312954));
#54603=CARTESIAN_POINT('Ctrl Pts',(-6.59293154067,-35.3836356047,-6.03737283826));
#54604=CARTESIAN_POINT('Ctrl Pts',(-6.59268825297,-35.4018088233,-6.03701670404));
#54605=CARTESIAN_POINT('Ctrl Pts',(-6.59270812441,-35.4199820418,-6.03698498184));
#54606=CARTESIAN_POINT('Ctrl Pts',(-7.36674622516,-35.3292429118,-5.37908303219));
#54607=CARTESIAN_POINT('Ctrl Pts',(-7.36563384979,-35.3471062503,-5.37795639383));
#54608=CARTESIAN_POINT('Ctrl Pts',(-7.36479211144,-35.3650081661,-5.37711871787));
#54609=CARTESIAN_POINT('Ctrl Pts',(-7.36422260417,-35.3829359555,-5.37657056503));
#54610=CARTESIAN_POINT('Ctrl Pts',(-7.36392615799,-35.4008766793,-5.37631208835));
#54611=CARTESIAN_POINT('Ctrl Pts',(-7.36390280813,-35.4188174032,-5.37634302053));
#54612=CARTESIAN_POINT('Ctrl Pts',(-8.06644392307,-35.3242511579,-4.63577831824));
#54613=CARTESIAN_POINT('Ctrl Pts',(-8.06481498329,-35.3443613723,-4.63450682037));
#54614=CARTESIAN_POINT('Ctrl Pts',(-8.06356784153,-35.3645192368,-4.63357464248));
#54615=CARTESIAN_POINT('Ctrl Pts',(-8.06270291188,-35.3847087915,-4.63298305339));
#54616=CARTESIAN_POINT('Ctrl Pts',(-8.06222041463,-35.4049141939,-4.63273277941));
#54617=CARTESIAN_POINT('Ctrl Pts',(-8.06212040397,-35.4251195963,-4.63282401372));
#54618=CARTESIAN_POINT('Ctrl Pts',(-8.40676939645,-35.318254221,-4.22563363488));
#54619=CARTESIAN_POINT('Ctrl Pts',(-8.40459143683,-35.3405015468,-4.22453866256));
#54620=CARTESIAN_POINT('Ctrl Pts',(-8.40288571682,-35.3628356427,-4.22380563891));
#54621=CARTESIAN_POINT('Ctrl Pts',(-8.40165936546,-35.3852283571,-4.22343491308));
#54622=CARTESIAN_POINT('Ctrl Pts',(-8.40091620766,-35.4076503711,-4.22342586623));
#54623=CARTESIAN_POINT('Ctrl Pts',(-8.40065659496,-35.4300723851,-4.22377686476));
#54624=CARTESIAN_POINT('Ctrl Pts',(-8.6986202738,-35.3007569312,-3.78649453504));
#54625=CARTESIAN_POINT('Ctrl Pts',(-8.69512018043,-35.3302263046,-3.78463499808));
#54626=CARTESIAN_POINT('Ctrl Pts',(-8.69237513121,-35.3597713122,-3.78337739168));
#54627=CARTESIAN_POINT('Ctrl Pts',(-8.69038139929,-35.3893659949,-3.78272454109));
#54628=CARTESIAN_POINT('Ctrl Pts',(-8.68913711634,-35.4189855209,-3.78267851397));
#54629=CARTESIAN_POINT('Ctrl Pts',(-8.68864247336,-35.4486050468,-3.78324063488));
#54630=CARTESIAN_POINT('Ctrl Pts',(-8.93444618031,-35.2748044449,-3.31652377072));
#54631=CARTESIAN_POINT('Ctrl Pts',(-8.92616350743,-35.3147858017,-3.31461838858));
#54632=CARTESIAN_POINT('Ctrl Pts',(-8.91971795914,-35.3551905608,-3.31361146728));
#54633=CARTESIAN_POINT('Ctrl Pts',(-8.91513837409,-35.3958795596,-3.31350964329));
#54634=CARTESIAN_POINT('Ctrl Pts',(-8.91244074774,-35.4367106808,-3.31431327227));
#54635=CARTESIAN_POINT('Ctrl Pts',(-8.91162790031,-35.4775418019,-3.31601642165));
#54636=CARTESIAN_POINT('Origin',(-2.2221106022258,-35.495269847715,-9.19615921132892));
#54637=CARTESIAN_POINT('Ctrl Pts',(-1.88395974093662,-35.2523605115009,
-8.27259966015858));
#54638=CARTESIAN_POINT('Ctrl Pts',(-1.88009563783341,-35.2998111449227,
-8.26124833618188));
#54639=CARTESIAN_POINT('Ctrl Pts',(-1.8767191336114,-35.3479866024315,-8.25276092720707));
#54640=CARTESIAN_POINT('Ctrl Pts',(-1.87384951644931,-35.3966500949375,
-8.24719410915978));
#54641=CARTESIAN_POINT('Ctrl Pts',(-1.87150117757236,-35.4455575723249,
-8.24457579968163));
#54642=CARTESIAN_POINT('Ctrl Pts',(-1.86968318420237,-35.4944649688017,
-8.24490433018094));
#54643=CARTESIAN_POINT('Ctrl Pts',(-1.91300759658597,-35.2527339398473,
-8.26755957224482));
#54644=CARTESIAN_POINT('Ctrl Pts',(-1.9097199029017,-35.3003685469398,-8.25602454207901));
#54645=CARTESIAN_POINT('Ctrl Pts',(-1.90694145962302,-35.3487360921407,
-8.24737013222748));
#54646=CARTESIAN_POINT('Ctrl Pts',(-1.90468881485147,-35.3975971714161,
-8.24165434232319));
#54647=CARTESIAN_POINT('Ctrl Pts',(-1.90297337398542,-35.4467049836923,
-8.23890603779062));
#54648=CARTESIAN_POINT('Ctrl Pts',(-1.90180104448326,-35.4958127139372,
-8.23912408927851));
#54649=CARTESIAN_POINT('Ctrl Pts',(-1.94218018572405,-35.2535044474158,
-8.2621591143811));
#54650=CARTESIAN_POINT('Ctrl Pts',(-1.93948439180326,-35.3011355726151,
-8.25052643519998));
#54651=CARTESIAN_POINT('Ctrl Pts',(-1.93731618833942,-35.3494991334594,
-8.24176908020048));
#54652=CARTESIAN_POINT('Ctrl Pts',(-1.9356894040532,-35.3983557916441,-8.23594548297372));
#54653=CARTESIAN_POINT('Ctrl Pts',(-1.93461165570096,-35.4474591093103,
-8.23308511017217));
#54654=CARTESIAN_POINT('Ctrl Pts',(-1.93408585739421,-35.4965623450722,
-8.23318738466497));
#54655=CARTESIAN_POINT('Ctrl Pts',(-1.9724911224602,-35.2538279318595,-8.25640089670514));
#54656=CARTESIAN_POINT('Ctrl Pts',(-1.96989995083931,-35.3014474096544,
-8.2447738198874));
#54657=CARTESIAN_POINT('Ctrl Pts',(-1.96784715401122,-35.3497975316059,
-8.23601549714894));
#54658=CARTESIAN_POINT('Ctrl Pts',(-1.96632241972348,-35.3986473889607,
-8.23018671944173));
#54659=CARTESIAN_POINT('Ctrl Pts',(-1.96537905911117,-35.4477354015217,
-8.22731155195785));
#54660=CARTESIAN_POINT('Ctrl Pts',(-1.9649957888598,-35.4968233351047,-8.22739248875143));
#54661=CARTESIAN_POINT('Ctrl Pts',(-2.00036048734845,-35.2563328498845,
-8.25033564485486));
#54662=CARTESIAN_POINT('Ctrl Pts',(-1.9989276215456,-35.3033816639248,-8.23877146644499));
#54663=CARTESIAN_POINT('Ctrl Pts',(-1.9980459932212,-35.3511346917004,-8.2300037370207));
#54664=CARTESIAN_POINT('Ctrl Pts',(-1.99772296424743,-35.3993616720185,
-8.22408907865538));
#54665=CARTESIAN_POINT('Ctrl Pts',(-1.99795923658066,-35.4478257884428,
-8.2210566696507));
#54666=CARTESIAN_POINT('Ctrl Pts',(-1.99875127112907,-35.4962898261243,
-8.22090710192112));
#54667=CARTESIAN_POINT('Ctrl Pts',(-2.02950436722481,-35.2581725723914,
-8.2439568163922));
#54668=CARTESIAN_POINT('Ctrl Pts',(-2.02862442295225,-35.3046828131338,
-8.23255380319936));
#54669=CARTESIAN_POINT('Ctrl Pts',(-2.0282990861559,-35.3518728653025,-8.22388078348058));
#54670=CARTESIAN_POINT('Ctrl Pts',(-2.02853256285331,-35.3995204524209,
-8.2179922787766));
#54671=CARTESIAN_POINT('Ctrl Pts',(-2.0293237410715,-35.4473967740714,-8.2149165636107));
#54672=CARTESIAN_POINT('Ctrl Pts',(-2.03066619547392,-35.4952730196676,
-8.2146548655385));
#54673=CARTESIAN_POINT('Origin',(-2.04762566711772,-35.4944692176037,-9.22894616712353));
#54674=CARTESIAN_POINT('Ctrl Pts',(-1.46090085849,-35.2135310847,-7.94951679032));
#54675=CARTESIAN_POINT('Ctrl Pts',(-1.48323559961,-35.2772019758,-7.94951679554));
#54676=CARTESIAN_POINT('Ctrl Pts',(-1.50020012625,-35.3427566518,-7.94951680076));
#54677=CARTESIAN_POINT('Ctrl Pts',(-1.51158239151,-35.4095912303,-7.94951680594));
#54678=CARTESIAN_POINT('Ctrl Pts',(-1.51727342189,-35.4770658384,-7.94951681101));
#54679=CARTESIAN_POINT('Ctrl Pts',(-1.5172734197,-35.5445404466,-7.94951681593));
#54680=CARTESIAN_POINT('Ctrl Pts',(-1.46090084734,-35.2135310529,-7.95714134841));
#54681=CARTESIAN_POINT('Ctrl Pts',(-1.48323559207,-35.2772019436,-7.95594579353));
#54682=CARTESIAN_POINT('Ctrl Pts',(-1.50020012179,-35.3427566195,-7.95475023866));
#54683=CARTESIAN_POINT('Ctrl Pts',(-1.51158238894,-35.4095911981,-7.95356602458));
#54684=CARTESIAN_POINT('Ctrl Pts',(-1.51727341997,-35.4770658064,-7.95240448782));
#54685=CARTESIAN_POINT('Ctrl Pts',(-1.51727341782,-35.5445404148,-7.95127632944));
#54686=CARTESIAN_POINT('Ctrl Pts',(-1.46095673562,-35.2136903768,-7.96472994159));
#54687=CARTESIAN_POINT('Ctrl Pts',(-1.48329083274,-35.277359414,-7.96234446573));
#54688=CARTESIAN_POINT('Ctrl Pts',(-1.50025081243,-35.3429136053,-7.95995898987));
#54689=CARTESIAN_POINT('Ctrl Pts',(-1.51162447777,-35.4097486473,-7.95759614371));
#54690=CARTESIAN_POINT('Ctrl Pts',(-1.51730285882,-35.477224193,-7.95527854376));
#54691=CARTESIAN_POINT('Ctrl Pts',(-1.51728631578,-35.5446997387,-7.9530275433));
#54692=CARTESIAN_POINT('Ctrl Pts',(-1.46106747229,-35.2140060602,-7.97227569366));
#54693=CARTESIAN_POINT('Ctrl Pts',(-1.48340028139,-35.277671426,-7.9687069317));
#54694=CARTESIAN_POINT('Ctrl Pts',(-1.50035124089,-35.3432246581,-7.96513816975));
#54695=CARTESIAN_POINT('Ctrl Pts',(-1.51170786352,-35.4100606172,-7.96160330128));
#54696=CARTESIAN_POINT('Ctrl Pts',(-1.51736118389,-35.4775380197,-7.95813620969));
#54697=CARTESIAN_POINT('Ctrl Pts',(-1.51731187088,-35.5450154221,-7.95476887067));
#54698=CARTESIAN_POINT('Ctrl Pts',(-1.4612316362,-35.2144740518,-7.97977268509));
#54699=CARTESIAN_POINT('Ctrl Pts',(-1.48356253349,-35.2781339746,-7.97502812195));
#54700=CARTESIAN_POINT('Ctrl Pts',(-1.50050012169,-35.3436857837,-7.9702835588));
#54701=CARTESIAN_POINT('Ctrl Pts',(-1.51183147778,-35.4105231034,-7.96558416229));
#54702=CARTESIAN_POINT('Ctrl Pts',(-1.51744764399,-35.4780032585,-7.96097508922));
#54703=CARTESIAN_POINT('Ctrl Pts',(-1.51734975497,-35.5454834136,-7.95649894554));
#54704=CARTESIAN_POINT('Ctrl Pts',(-1.461447583,-35.2150896638,-7.9872159128));
#54705=CARTESIAN_POINT('Ctrl Pts',(-1.48377596485,-35.2787424258,-7.98130374694));
#54706=CARTESIAN_POINT('Ctrl Pts',(-1.50069596198,-35.3442923623,-7.97539158107));
#54707=CARTESIAN_POINT('Ctrl Pts',(-1.51199407822,-35.4111314721,-7.96953589364));
#54708=CARTESIAN_POINT('Ctrl Pts',(-1.51756136975,-35.4786152489,-7.963793149));
#54709=CARTESIAN_POINT('Ctrl Pts',(-1.5173995886,-35.5460990256,-7.95821661336));
#54710=CARTESIAN_POINT('Origin',(-0.517271904869316,-35.5445407938528,-7.94950153701101));
#54711=CARTESIAN_POINT('Origin',(-0.517817922218787,-35.5460995791193,-7.98721621984755));
#54712=CARTESIAN_POINT('Ctrl Pts',(-1.46144763142,-35.2150898018,-7.98721591698));
#54713=CARTESIAN_POINT('Ctrl Pts',(-1.48377600029,-35.278742568,-7.9813037531));
#54714=CARTESIAN_POINT('Ctrl Pts',(-1.50069598676,-35.344292508,-7.97539158967));
#54715=CARTESIAN_POINT('Ctrl Pts',(-1.51199409489,-35.4111316208,-7.96953590506));
#54716=CARTESIAN_POINT('Ctrl Pts',(-1.51756138096,-35.4786154003,-7.96379316359));
#54717=CARTESIAN_POINT('Ctrl Pts',(-1.51739959704,-35.5460991799,-7.95821663141));
#54718=CARTESIAN_POINT('Ctrl Pts',(-1.45535023282,-35.1977075828,-8.04883580535));
#54719=CARTESIAN_POINT('Ctrl Pts',(-1.48166949688,-35.2678829449,-8.03945279279));
#54720=CARTESIAN_POINT('Ctrl Pts',(-1.50141667723,-35.3406016986,-8.03107453153));
#54721=CARTESIAN_POINT('Ctrl Pts',(-1.51429114701,-35.4150544061,-8.02380364128));
#54722=CARTESIAN_POINT('Ctrl Pts',(-1.52014358616,-35.4903742161,-8.01772327965));
#54723=CARTESIAN_POINT('Ctrl Pts',(-1.51898580713,-35.5656940262,-8.01289172937));
#54724=CARTESIAN_POINT('Ctrl Pts',(-1.46435245205,-35.1856198088,-8.11169781125));
#54725=CARTESIAN_POINT('Ctrl Pts',(-1.49329848629,-35.2601192136,-8.09750578865));
#54726=CARTESIAN_POINT('Ctrl Pts',(-1.51493019199,-35.3378102208,-8.08590190484));
#54727=CARTESIAN_POINT('Ctrl Pts',(-1.52885470957,-35.4176855473,-8.07706315905));
#54728=CARTESIAN_POINT('Ctrl Pts',(-1.53488112404,-35.4986532993,-8.07110658123));
#54729=CARTESIAN_POINT('Ctrl Pts',(-1.53303520019,-35.5796210507,-8.06808053282));
#54730=CARTESIAN_POINT('Ctrl Pts',(-1.49172176542,-35.1799552596,-8.17111299923));
#54731=CARTESIAN_POINT('Ctrl Pts',(-1.51992397896,-35.2563325377,-8.15127801209));
#54732=CARTESIAN_POINT('Ctrl Pts',(-1.54120100093,-35.3362785459,-8.13597848758));
#54733=CARTESIAN_POINT('Ctrl Pts',(-1.5551380035,-35.4186751656,-8.12550808337));
#54734=CARTESIAN_POINT('Ctrl Pts',(-1.56152781403,-35.5022972201,-8.12002297191));
#54735=CARTESIAN_POINT('Ctrl Pts',(-1.5603885908,-35.5859192753,-8.11952822853));
#54736=CARTESIAN_POINT('Ctrl Pts',(-1.57027832078,-35.1818573291,-8.25620202557));
#54737=CARTESIAN_POINT('Ctrl Pts',(-1.59174100272,-35.2575761439,-8.2305972979));
#54738=CARTESIAN_POINT('Ctrl Pts',(-1.60864769834,-35.3366611931,-8.21163579835));
#54739=CARTESIAN_POINT('Ctrl Pts',(-1.62070812016,-35.4180526309,-8.19967893383));
#54740=CARTESIAN_POINT('Ctrl Pts',(-1.62775389781,-35.5005977196,-8.19489712008));
#54741=CARTESIAN_POINT('Ctrl Pts',(-1.62975211946,-35.5831428078,-8.19725603749));
#54742=CARTESIAN_POINT('Ctrl Pts',(-1.67937525828,-35.2054111593,-8.29244102122));
#54743=CARTESIAN_POINT('Ctrl Pts',(-1.69139601914,-35.2726177891,-8.26960761361));
#54744=CARTESIAN_POINT('Ctrl Pts',(-1.70188615133,-35.3420423454,-8.25274940255));
#54745=CARTESIAN_POINT('Ctrl Pts',(-1.7107273602,-35.4129758871,-8.24210785095));
#54746=CARTESIAN_POINT('Ctrl Pts',(-1.71782785643,-35.4846639068,-8.23779633493));
#54747=CARTESIAN_POINT('Ctrl Pts',(-1.72312748813,-35.5563519268,-8.23979333534));
#54748=CARTESIAN_POINT('Ctrl Pts',(-1.73126212215,-35.2199435259,-8.29740056817));
#54749=CARTESIAN_POINT('Ctrl Pts',(-1.73944999004,-35.2817848557,-8.27769690404));
#54750=CARTESIAN_POINT('Ctrl Pts',(-1.74724337723,-35.3452273068,-8.26303381776));
#54751=CARTESIAN_POINT('Ctrl Pts',(-1.75458028421,-35.4097526752,-8.25356881995));
#54752=CARTESIAN_POINT('Ctrl Pts',(-1.76140026731,-35.4748200605,-8.24938018459));
#54753=CARTESIAN_POINT('Ctrl Pts',(-1.7676477796,-35.5398874456,-8.25046377193));
#54754=CARTESIAN_POINT('Ctrl Pts',(-1.78213085799,-35.2383375006,-8.29255588031));
#54755=CARTESIAN_POINT('Ctrl Pts',(-1.7878752107,-35.2931533399,-8.27665796781));
#54756=CARTESIAN_POINT('Ctrl Pts',(-1.79382722081,-35.3490506456,-8.26463904937));
#54757=CARTESIAN_POINT('Ctrl Pts',(-1.79995135062,-35.4056781551,-8.25659979182));
#54758=CARTESIAN_POINT('Ctrl Pts',(-1.80620870196,-35.4626704426,-8.2525916122));
#54759=CARTESIAN_POINT('Ctrl Pts',(-1.81255794182,-35.5196627301,-8.25261467335));
#54760=CARTESIAN_POINT('Ctrl Pts',(-1.83110005152,-35.2589529157,-8.27964657201));
#54761=CARTESIAN_POINT('Ctrl Pts',(-1.83516520879,-35.3056415029,-8.26740924886));
#54762=CARTESIAN_POINT('Ctrl Pts',(-1.83967790698,-35.3530283973,-8.25798482029));
#54763=CARTESIAN_POINT('Ctrl Pts',(-1.84461828078,-35.4008854025,-8.25143312625));
#54764=CARTESIAN_POINT('Ctrl Pts',(-1.84996206575,-35.4489774707,-8.24778634512));
#54765=CARTESIAN_POINT('Ctrl Pts',(-1.85568130399,-35.4970695389,-8.24704805785));
#54766=CARTESIAN_POINT('Origin',(-1.98370762109533,-35.4970695944798,-9.23881946100821));
#54767=CARTESIAN_POINT('Ctrl Pts',(-1.8311006173,-35.2589545751,-8.27964607156));
#54768=CARTESIAN_POINT('Ctrl Pts',(-1.83516599722,-35.30564267,-8.26740892391));
#54769=CARTESIAN_POINT('Ctrl Pts',(-1.83967892993,-35.3530290502,-8.25798461135));
#54770=CARTESIAN_POINT('Ctrl Pts',(-1.84461954945,-35.4008855262,-8.25143297176));
#54771=CARTESIAN_POINT('Ctrl Pts',(-1.84996359063,-35.4489770577,-8.24778618257));
#54772=CARTESIAN_POINT('Ctrl Pts',(-1.85568309486,-35.4970685893,-8.24704782502));
#54773=CARTESIAN_POINT('Ctrl Pts',(-1.8411549102,-35.2563947443,-8.27868180069));
#54774=CARTESIAN_POINT('Ctrl Pts',(-1.84372513023,-35.3033039498,-8.26655797443));
#54775=CARTESIAN_POINT('Ctrl Pts',(-1.84674896075,-35.3509164835,-8.25725221826));
#54776=CARTESIAN_POINT('Ctrl Pts',(-1.85021379554,-35.3990025183,-8.25082395949));
#54777=CARTESIAN_POINT('Ctrl Pts',(-1.85410255764,-35.447325312,-8.24730484866));
#54778=CARTESIAN_POINT('Ctrl Pts',(-1.85839419939,-35.4956481058,-8.24669783586));
#54779=CARTESIAN_POINT('Ctrl Pts',(-1.8515433823,-35.25441601,-8.27750101411));
#54780=CARTESIAN_POINT('Ctrl Pts',(-1.85257607592,-35.3015060532,-8.26552228872));
#54781=CARTESIAN_POINT('Ctrl Pts',(-1.85406935318,-35.3493041477,-8.25636790881));
#54782=CARTESIAN_POINT('Ctrl Pts',(-1.85601808078,-35.3975789365,-8.25009675826));
#54783=CARTESIAN_POINT('Ctrl Pts',(-1.8584126658,-35.4460920799,-8.24673979731));
#54784=CARTESIAN_POINT('Ctrl Pts',(-1.86123915467,-35.4946052233,-8.24629917315));
#54785=CARTESIAN_POINT('Ctrl Pts',(-1.86227923956,-35.2530824801,-8.2760758565));
#54786=CARTESIAN_POINT('Ctrl Pts',(-1.86172760863,-35.3003142451,-8.26427721621));
#54787=CARTESIAN_POINT('Ctrl Pts',(-1.86164442165,-35.3482586468,-8.25531090742));
#54788=CARTESIAN_POINT('Ctrl Pts',(-1.86203232275,-35.3966828431,-8.24923515298));
#54789=CARTESIAN_POINT('Ctrl Pts',(-1.86288941138,-35.4453469517,-8.24608002563));
#54790=CARTESIAN_POINT('Ctrl Pts',(-1.86420909862,-35.4940110603,-8.24584666363));
#54791=CARTESIAN_POINT('Ctrl Pts',(-1.8733302454,-35.2524719557,-8.27438297071));
#54792=CARTESIAN_POINT('Ctrl Pts',(-1.87114978057,-35.2998071163,-8.26280107324));
#54793=CARTESIAN_POINT('Ctrl Pts',(-1.86944655662,-35.34785966,-8.25406232754));
#54794=CARTESIAN_POINT('Ctrl Pts',(-1.8682313281,-35.3963952193,-8.24822411924));
#54795=CARTESIAN_POINT('Ctrl Pts',(-1.8675100956,-35.4451722935,-8.24531550566));
#54796=CARTESIAN_POINT('Ctrl Pts',(-1.86728392959,-35.4939493677,-8.24533636007));
#54797=CARTESIAN_POINT('Ctrl Pts',(-1.88461561635,-35.2526204897,-8.27242216736));
#54798=CARTESIAN_POINT('Ctrl Pts',(-1.88077145213,-35.3000228694,-8.26109202298));
#54799=CARTESIAN_POINT('Ctrl Pts',(-1.87741430691,-35.3481478104,-8.25261964893));
#54800=CARTESIAN_POINT('Ctrl Pts',(-1.87456332753,-35.3967592797,-8.24706149184));
#54801=CARTESIAN_POINT('Ctrl Pts',(-1.87223278053,-35.4456140212,-8.24444536521));
#54802=CARTESIAN_POINT('Ctrl Pts',(-1.87043162953,-35.4944687629,-8.2447696254));
#54803=CARTESIAN_POINT('Origin',(-0.517276095271889,-35.5445396177181,-6.5565839998119));
#54804=CARTESIAN_POINT('Origin',(-4.19954447987E-15,-32.5742356128,1.22464679915E-17));
#54805=CARTESIAN_POINT('',(9.27193478991,-32.4742356128,12.7934055377));
#54806=CARTESIAN_POINT('Origin',(9.27193478991,-32.5742356128,12.7934055377));
#54807=CARTESIAN_POINT('',(-8.84971102033,-32.4742356128,13.0890265053));
#54808=CARTESIAN_POINT('Origin',(9.55224857921E-16,-32.4742356128,-1.40227797601E-15));
#54809=CARTESIAN_POINT('Origin',(-8.84971102033,-32.5742356128,13.0890265053));
#54810=CARTESIAN_POINT('Origin',(9.15456852675,-32.5742356128,12.6314636954));
#54811=CARTESIAN_POINT('',(9.29417531907,-32.4742356128,12.4882507647));
#54812=CARTESIAN_POINT('Origin',(9.29417531907,-32.5742356128,12.4882507647));
#54813=CARTESIAN_POINT('Origin',(9.15456852675,-32.4742356128,12.6314636954));
#54814=CARTESIAN_POINT('Origin',(-0.316839226711,-32.5742356128,3.11924403781));
#54815=CARTESIAN_POINT('',(8.12053083925,-32.4742356128,11.3441589548));
#54816=CARTESIAN_POINT('Origin',(8.12053083925,-32.5742356128,11.3441589548));
#54817=CARTESIAN_POINT('',(8.70735307916,-32.4742356128,11.9162048597));
#54818=CARTESIAN_POINT('Origin',(8.39974442389,-32.5742356128,11.0577330933));
#54819=CARTESIAN_POINT('',(8.11331856237,-32.4742356128,10.7785195086));
#54820=CARTESIAN_POINT('Origin',(8.11331856237,-32.5742356128,10.7785195086));
#54821=CARTESIAN_POINT('Origin',(8.39974442389,-32.4742356128,11.0577330933));
#54822=CARTESIAN_POINT('Origin',(8.43647932171,-32.5742356128,10.447011287));
#54823=CARTESIAN_POINT('',(11.1212648448,-32.4742356128,7.69287592692));
#54824=CARTESIAN_POINT('Origin',(11.1212648448,-32.5742356128,7.69287592692));
#54825=CARTESIAN_POINT('',(9.6172917036,-32.4742356128,9.23569771778));
#54826=CARTESIAN_POINT('Origin',(11.4076907064,-32.5742356128,7.97208951156));
#54827=CARTESIAN_POINT('',(11.686904291,-32.4742356128,7.68566365004));
#54828=CARTESIAN_POINT('Origin',(11.686904291,-32.5742356128,7.68566365004));
#54829=CARTESIAN_POINT('Origin',(11.4076907064,-32.4742356128,7.97208951156));
#54830=CARTESIAN_POINT('Origin',(0.45986885604,-32.5742356128,-3.25867214427));
#54831=CARTESIAN_POINT('',(12.8348977878,-32.4742356128,8.80475037519));
#54832=CARTESIAN_POINT('Origin',(12.8348977878,-32.5742356128,8.80475037519));
#54833=CARTESIAN_POINT('',(12.2609010394,-32.4742356128,8.24520701262));
#54834=CARTESIAN_POINT('Origin',(12.9745045801,-32.5742356128,8.66153744443));
#54835=CARTESIAN_POINT('',(13.1408443824,-32.4742356128,8.77258279628));
#54836=CARTESIAN_POINT('Origin',(13.1408443824,-32.5742356128,8.77258279628));
#54837=CARTESIAN_POINT('Origin',(12.9745045801,-32.4742356128,8.66153744443));
#54838=CARTESIAN_POINT('Origin',(6.68547290961E-14,-32.5742356128,3.37630264166E-14));
#54839=CARTESIAN_POINT('',(14.1086187499,-32.4742356128,7.11244521731));
#54840=CARTESIAN_POINT('Origin',(14.1086187499,-32.5742356128,7.11244521731));
#54841=CARTESIAN_POINT('Origin',(-1.78359931397E-15,-32.4742356128,7.01138988003E-16));
#54842=CARTESIAN_POINT('Origin',(13.7514385284,-32.5742356128,6.93238331308));
#54843=CARTESIAN_POINT('',(14.1514385284,-32.4742356128,6.93238331308));
#54844=CARTESIAN_POINT('Origin',(14.1514385284,-32.5742356128,6.93238331308));
#54845=CARTESIAN_POINT('Origin',(13.7514385284,-32.4742356128,6.93238331308));
#54846=CARTESIAN_POINT('Origin',(14.1514385284,-32.5742356128,5.21140063714E-15));
#54847=CARTESIAN_POINT('',(14.1514385284,-32.4742356128,-6.93238331308));
#54848=CARTESIAN_POINT('Origin',(14.1514385284,-32.5742356128,-6.93238331308));
#54849=CARTESIAN_POINT('',(14.1514385284,-32.4742356128,6.2172489379E-15));
#54850=CARTESIAN_POINT('Origin',(13.7514385284,-32.5742356128,-6.93238331308));
#54851=CARTESIAN_POINT('',(14.1086187499,-32.4742356128,-7.11244521731));
#54852=CARTESIAN_POINT('Origin',(14.1086187499,-32.5742356128,-7.11244521731));
#54853=CARTESIAN_POINT('Origin',(13.7514385284,-32.4742356128,-6.93238331308));
#54854=CARTESIAN_POINT('Origin',(1.12952603833E-15,-32.5742356128,1.22464679915E-17));
#54855=CARTESIAN_POINT('',(13.1408443824,-32.4742356128,-8.77258279628));
#54856=CARTESIAN_POINT('Origin',(13.1408443824,-32.5742356128,-8.77258279628));
#54857=CARTESIAN_POINT('Origin',(-1.78359931397E-15,-32.4742356128,7.01138988003E-16));
#54858=CARTESIAN_POINT('Origin',(12.9745045801,-32.5742356128,-8.66153744443));
#54859=CARTESIAN_POINT('',(12.8348977878,-32.4742356128,-8.80475037519));
#54860=CARTESIAN_POINT('Origin',(12.8348977878,-32.5742356128,-8.80475037519));
#54861=CARTESIAN_POINT('Origin',(12.9745045801,-32.4742356128,-8.66153744443));
#54862=CARTESIAN_POINT('Origin',(0.45986885604,-32.5742356128,3.25867214427));
#54863=CARTESIAN_POINT('',(11.686904291,-32.4742356128,-7.68566365004));
#54864=CARTESIAN_POINT('Origin',(11.686904291,-32.5742356128,-7.68566365004));
#54865=CARTESIAN_POINT('',(12.2609010394,-32.4742356128,-8.24520701262));
#54866=CARTESIAN_POINT('Origin',(11.4076907064,-32.5742356128,-7.97208951156));
#54867=CARTESIAN_POINT('',(11.1212648448,-32.4742356128,-7.69287592692));
#54868=CARTESIAN_POINT('Origin',(11.1212648448,-32.5742356128,-7.69287592692));
#54869=CARTESIAN_POINT('Origin',(11.4076907064,-32.4742356128,-7.97208951156));
#54870=CARTESIAN_POINT('Origin',(8.43647932171,-32.5742356128,-10.447011287));
#54871=CARTESIAN_POINT('',(8.11331856237,-32.4742356128,-10.7785195086));
#54872=CARTESIAN_POINT('Origin',(8.11331856237,-32.5742356128,-10.7785195086));
#54873=CARTESIAN_POINT('',(9.6172917036,-32.4742356128,-9.23569771778));
#54874=CARTESIAN_POINT('Origin',(8.39974442389,-32.5742356128,-11.0577330933));
#54875=CARTESIAN_POINT('',(8.12053083925,-32.4742356128,-11.3441589548));
#54876=CARTESIAN_POINT('Origin',(8.12053083925,-32.5742356128,-11.3441589548));
#54877=CARTESIAN_POINT('Origin',(8.39974442389,-32.4742356128,-11.0577330933));
#54878=CARTESIAN_POINT('Origin',(-0.316839226711,-32.5742356128,-3.11924403781));
#54879=CARTESIAN_POINT('',(9.29417531907,-32.4742356128,-12.4882507647));
#54880=CARTESIAN_POINT('Origin',(9.29417531907,-32.5742356128,-12.4882507647));
#54881=CARTESIAN_POINT('',(8.70735307916,-32.4742356128,-11.9162048597));
#54882=CARTESIAN_POINT('Origin',(9.15456852675,-32.5742356128,-12.6314636954));
#54883=CARTESIAN_POINT('',(9.27193478991,-32.4742356128,-12.7934055377));
#54884=CARTESIAN_POINT('Origin',(9.27193478991,-32.5742356128,-12.7934055377));
#54885=CARTESIAN_POINT('Origin',(9.15456852675,-32.4742356128,-12.6314636954));
#54886=CARTESIAN_POINT('Origin',(1.12952603833E-15,-32.5742356128,-1.76411037141E-15));
#54887=CARTESIAN_POINT('',(-9.27193478991,-32.4742356128,-12.7934055377));
#54888=CARTESIAN_POINT('Origin',(-9.27193478991,-32.5742356128,-12.7934055377));
#54889=CARTESIAN_POINT('Origin',(-1.78359931397E-15,-32.4742356128,7.01138988003E-16));
#54890=CARTESIAN_POINT('Origin',(-9.15456852675,-32.5742356128,-12.6314636954));
#54891=CARTESIAN_POINT('',(-9.29417531907,-32.4742356128,-12.4882507647));
#54892=CARTESIAN_POINT('Origin',(-9.29417531907,-32.5742356128,-12.4882507647));
#54893=CARTESIAN_POINT('Origin',(-9.15456852675,-32.4742356128,-12.6314636954));
#54894=CARTESIAN_POINT('Origin',(0.316839226711,-32.5742356128,-3.11924403781));
#54895=CARTESIAN_POINT('',(-8.12053083925,-32.4742356128,-11.3441589548));
#54896=CARTESIAN_POINT('Origin',(-8.12053083925,-32.5742356128,-11.3441589548));
#54897=CARTESIAN_POINT('',(-8.70735307916,-32.4742356128,-11.9162048597));
#54898=CARTESIAN_POINT('Origin',(-8.39974442389,-32.5742356128,-11.0577330933));
#54899=CARTESIAN_POINT('',(-8.11331856237,-32.4742356128,-10.7785195086));
#54900=CARTESIAN_POINT('Origin',(-8.11331856237,-32.5742356128,-10.7785195086));
#54901=CARTESIAN_POINT('Origin',(-8.39974442389,-32.4742356128,-11.0577330933));
#54902=CARTESIAN_POINT('Origin',(-8.43647932171,-32.5742356128,-10.447011287));
#54903=CARTESIAN_POINT('',(-11.1212648448,-32.4742356128,-7.69287592692));
#54904=CARTESIAN_POINT('Origin',(-11.1212648448,-32.5742356128,-7.69287592692));
#54905=CARTESIAN_POINT('',(-9.6172917036,-32.4742356128,-9.23569771778));
#54906=CARTESIAN_POINT('Origin',(-11.4076907064,-32.5742356128,-7.97208951156));
#54907=CARTESIAN_POINT('',(-11.686904291,-32.4742356128,-7.68566365004));
#54908=CARTESIAN_POINT('Origin',(-11.686904291,-32.5742356128,-7.68566365004));
#54909=CARTESIAN_POINT('Origin',(-11.4076907064,-32.4742356128,-7.97208951156));
#54910=CARTESIAN_POINT('Origin',(-0.45986885604,-32.5742356128,3.25867214427));
#54911=CARTESIAN_POINT('',(-12.8348977878,-32.4742356128,-8.80475037519));
#54912=CARTESIAN_POINT('Origin',(-12.8348977878,-32.5742356128,-8.80475037519));
#54913=CARTESIAN_POINT('',(-12.2609010394,-32.4742356128,-8.24520701262));
#54914=CARTESIAN_POINT('Origin',(-12.9745045801,-32.5742356128,-8.66153744443));
#54915=CARTESIAN_POINT('',(-13.1408443824,-32.4742356128,-8.77258279628));
#54916=CARTESIAN_POINT('Origin',(-13.1408443824,-32.5742356128,-8.77258279628));
#54917=CARTESIAN_POINT('Origin',(-12.9745045801,-32.4742356128,-8.66153744443));
#54918=CARTESIAN_POINT('Origin',(1.12952603833E-15,-32.5742356128,1.22464679915E-17));
#54919=CARTESIAN_POINT('',(-14.1086187499,-32.4742356128,-7.11244521731));
#54920=CARTESIAN_POINT('Origin',(-14.1086187499,-32.5742356128,-7.11244521731));
#54921=CARTESIAN_POINT('Origin',(9.55224857921E-16,-32.4742356128,-1.40227797601E-15));
#54922=CARTESIAN_POINT('Origin',(-13.7514385284,-32.5742356128,-6.93238331308));
#54923=CARTESIAN_POINT('',(-14.1514385284,-32.4742356128,-6.93238331308));
#54924=CARTESIAN_POINT('Origin',(-14.1514385284,-32.5742356128,-6.93238331308));
#54925=CARTESIAN_POINT('Origin',(-13.7514385284,-32.4742356128,-6.93238331308));
#54926=CARTESIAN_POINT('Origin',(-14.1514385284,-32.5742356128,-5.18690770115E-15));
#54927=CARTESIAN_POINT('',(-14.1514385284,-32.4742356128,6.93238331308));
#54928=CARTESIAN_POINT('Origin',(-14.1514385284,-32.5742356128,6.93238331308));
#54929=CARTESIAN_POINT('',(-14.1514385284,-32.4742356128,-2.6645352591E-15));
#54930=CARTESIAN_POINT('Origin',(-13.7514385284,-32.5742356128,6.93238331308));
#54931=CARTESIAN_POINT('',(-14.1086187499,-32.4742356128,7.11244521731));
#54932=CARTESIAN_POINT('Origin',(-14.1086187499,-32.5742356128,7.11244521731));
#54933=CARTESIAN_POINT('Origin',(-13.7514385284,-32.4742356128,6.93238331308));
#54934=CARTESIAN_POINT('Origin',(6.95023748177E-12,-32.5742356128,-3.88843287498E-12));
#54935=CARTESIAN_POINT('',(-13.4206904888,-32.4742356128,8.33816927169));
#54936=CARTESIAN_POINT('Origin',(-13.4206904888,-32.5742356128,8.33816927169));
#54937=CARTESIAN_POINT('Origin',(9.55224857921E-16,-32.4742356128,-1.40227797601E-15));
#54938=CARTESIAN_POINT('Origin',(-13.2508083307,-32.5742356128,8.23262282521));
#54939=CARTESIAN_POINT('',(-13.1112015384,-32.4742356128,8.37583575597));
#54940=CARTESIAN_POINT('Origin',(-13.1112015384,-32.5742356128,8.37583575597));
#54941=CARTESIAN_POINT('Origin',(-13.2508083307,-32.4742356128,8.23262282521));
#54942=CARTESIAN_POINT('Origin',(-0.818017619209,-32.5742356128,-3.60780262944));
#54943=CARTESIAN_POINT('',(-12.0359212718,-32.4742356128,7.32763132313));
#54944=CARTESIAN_POINT('Origin',(-12.0359212718,-32.5742356128,7.32763132313));
#54945=CARTESIAN_POINT('',(-12.5735614051,-32.4742356128,7.85173353955));
#54946=CARTESIAN_POINT('Origin',(-11.7567076872,-32.5742356128,7.61405718465));
#54947=CARTESIAN_POINT('',(-11.4702818256,-32.4742356128,7.33484360001));
#54948=CARTESIAN_POINT('Origin',(-11.4702818256,-32.5742356128,7.33484360001));
#54949=CARTESIAN_POINT('Origin',(-11.7567076872,-32.4742356128,7.61405718465));
#54950=CARTESIAN_POINT('Origin',(-8.43647932171,-32.5742356128,10.447011287));
#54951=CARTESIAN_POINT('',(-7.76430158156,-32.4742356128,11.1365518355));
#54952=CARTESIAN_POINT('Origin',(-7.76430158156,-32.5742356128,11.1365518355));
#54953=CARTESIAN_POINT('',(-9.6172917036,-32.4742356128,9.23569771778));
#54954=CARTESIAN_POINT('Origin',(-8.73768936184,-32.5742356128,12.9233426255));
#54955=CARTESIAN_POINT('',(-8.87729615416,-32.4742356128,12.7801296947));
#54956=CARTESIAN_POINT('Origin',(-8.73768936184,-32.4742356128,12.9233426255));
#54957=CARTESIAN_POINT('Origin',(-8.87729615416,-32.5742356128,12.7801296947));
#54958=CARTESIAN_POINT('Origin',(-8.05072744309,-32.5742356128,11.4157654202));
#54959=CARTESIAN_POINT('',(-7.77151385845,-32.4742356128,11.7021912817));
#54960=CARTESIAN_POINT('Origin',(-7.77151385845,-32.5742356128,11.7021912817));
#54961=CARTESIAN_POINT('Origin',(-8.05072744309,-32.4742356128,11.4157654202));
#54962=CARTESIAN_POINT('Origin',(0.67498798988,-32.5742356128,3.46837452298));
#54963=CARTESIAN_POINT('',(-8.3244050063,-32.4742356128,12.2411604882));
#54964=CARTESIAN_POINT('Origin',(-6.22337865086E-16,-32.4742356128,0.));
#54965=CARTESIAN_POINT('',(12.4493324411,-32.4742356128,6.47376294621));
#54966=CARTESIAN_POINT('',(12.3114960897,-32.4742356128,6.33939734959));
#54967=CARTESIAN_POINT('',(10.328184518,-32.4742356128,6.50080898452));
#54968=CARTESIAN_POINT('Origin',(11.4022814987,-32.4742356128,7.54785992694));
#54969=CARTESIAN_POINT('',(6.90141785854,-32.4742356128,10.0160913585));
#54970=CARTESIAN_POINT('',(8.61480118826,-32.4742356128,8.25845017153));
#54971=CARTESIAN_POINT('',(6.92846389685,-32.4742356128,12.1372392817));
#54972=CARTESIAN_POINT('Origin',(7.97551483927,-32.4742356128,11.0631423009));
#54973=CARTESIAN_POINT('',(7.24427528424,-32.4742356128,12.4450984571));
#54974=CARTESIAN_POINT('',(6.79621292104,-32.4742356128,12.0083184194));
#54975=CARTESIAN_POINT('',(-6.7887641255,-32.4742356128,12.6993181568));
#54976=CARTESIAN_POINT('Origin',(-6.22337865086E-16,-32.4742356128,-9.86076131526E-32));
#54977=CARTESIAN_POINT('',(-6.57944691605,-32.4742356128,12.4952716086));
#54978=CARTESIAN_POINT('',(-6.14705703041,-32.4742356128,12.0737694115));
#54979=CARTESIAN_POINT('',(-6.55240087774,-32.4742356128,10.3741236854));
#54980=CARTESIAN_POINT('Origin',(-7.62649785846,-32.4742356128,11.4211746278));
#54981=CARTESIAN_POINT('',(-10.6782005908,-32.4742356128,6.14175175838));
#54982=CARTESIAN_POINT('',(-8.61480118826,-32.4742356128,8.25845017153));
#54983=CARTESIAN_POINT('Origin',(-11.7522975715,-32.4742356128,7.18880270079));
#54984=CARTESIAN_POINT('',(-10.328184518,-32.4742356128,-6.50080898452));
#54985=CARTESIAN_POINT('Origin',(-11.4022814987,-32.4742356128,-7.54785992694));
#54986=CARTESIAN_POINT('',(-6.90141785854,-32.4742356128,-10.0160913585));
#54987=CARTESIAN_POINT('',(-8.61480118826,-32.4742356128,-8.25845017153));
#54988=CARTESIAN_POINT('',(-6.92846389685,-32.4742356128,-12.1372392817));
#54989=CARTESIAN_POINT('Origin',(-7.97551483927,-32.4742356128,-11.0631423009));
#54990=CARTESIAN_POINT('',(-7.24427528424,-32.4742356128,-12.4450984571));
#54991=CARTESIAN_POINT('',(-6.79621292104,-32.4742356128,-12.0083184194));
#54992=CARTESIAN_POINT('',(7.24427528424,-32.4742356128,-12.4450984571));
#54993=CARTESIAN_POINT('Origin',(-6.22337865086E-16,-32.4742356128,-9.86076131526E-32));
#54994=CARTESIAN_POINT('',(6.92846389685,-32.4742356128,-12.1372392817));
#54995=CARTESIAN_POINT('',(6.79621292104,-32.4742356128,-12.0083184194));
#54996=CARTESIAN_POINT('',(6.90141785854,-32.4742356128,-10.0160913585));
#54997=CARTESIAN_POINT('Origin',(7.97551483927,-32.4742356128,-11.0631423009));
#54998=CARTESIAN_POINT('',(10.328184518,-32.4742356128,-6.50080898452));
#54999=CARTESIAN_POINT('',(8.61480118826,-32.4742356128,-8.25845017153));
#55000=CARTESIAN_POINT('Origin',(11.4022814987,-32.4742356128,-7.54785992694));
#55001=CARTESIAN_POINT('Origin',(-1.09995011675E-15,-34.4242356128,2.38806125834E-16));
#55002=CARTESIAN_POINT('',(7.24427528424,-32.8742356128,-12.4450984571));
#55003=CARTESIAN_POINT('',(7.24427528424,-33.6742356128,-12.4450984571));
#55004=CARTESIAN_POINT('',(-7.24427528424,-32.8742356128,-12.4450984571));
#55005=CARTESIAN_POINT('',(-7.24427528424,-33.6742356128,-12.4450984571));
#55006=CARTESIAN_POINT('Origin',(5.26886406864393E-14,-32.8742356128,2.66453525910038E-14));
#55007=CARTESIAN_POINT('Origin',(12.4493324411,-32.4742356128,6.47376294621));
#55008=CARTESIAN_POINT('',(12.4493324411,-32.8742356128,6.47376294621));
#55009=CARTESIAN_POINT('',(12.4493324411,-32.8742356128,6.47376294621));
#55010=CARTESIAN_POINT('',(12.4493324411,-32.6742356128,6.47376294621));
#55011=CARTESIAN_POINT('Origin',(6.92846389685,-32.4742356128,-12.1372392817));
#55012=CARTESIAN_POINT('',(6.92846389685,-32.8742356128,-12.1372392817));
#55013=CARTESIAN_POINT('',(6.92846389685,-32.8742356128,-12.1372392817));
#55014=CARTESIAN_POINT('',(6.92846389685,-32.6742356128,-12.1372392817));
#55015=CARTESIAN_POINT('Origin',(7.97551483927,-32.6742356128,-11.0631423009));
#55016=CARTESIAN_POINT('',(6.90141785854,-32.8742356128,-10.0160913585));
#55017=CARTESIAN_POINT('Origin',(7.97551483927,-32.8742356128,-11.0631423009));
#55018=CARTESIAN_POINT('',(6.90141785854,-33.6742356128,-10.0160913585));
#55019=CARTESIAN_POINT('Origin',(10.328184518,-32.4742356128,-6.50080898452));
#55020=CARTESIAN_POINT('',(10.328184518,-32.8742356128,-6.50080898452));
#55021=CARTESIAN_POINT('',(10.328184518,-32.8742356128,-6.50080898452));
#55022=CARTESIAN_POINT('',(10.328184518,-32.6742356128,-6.50080898452));
#55023=CARTESIAN_POINT('Origin',(11.4022814987,-32.6742356128,-7.54785992694));
#55024=CARTESIAN_POINT('Origin',(11.4022814987,-32.8742356128,-7.54785992694));
#55025=CARTESIAN_POINT('Origin',(10.328184518,-32.4742356128,6.50080898452));
#55026=CARTESIAN_POINT('',(10.328184518,-32.8742356128,6.50080898452));
#55027=CARTESIAN_POINT('',(10.328184518,-32.6742356128,6.50080898452));
#55028=CARTESIAN_POINT('',(6.90141785854,-32.8742356128,10.0160913585));
#55029=CARTESIAN_POINT('',(10.328184518,-32.8742356128,6.50080898452));
#55030=CARTESIAN_POINT('',(6.90141785854,-32.6742356128,10.0160913585));
#55031=CARTESIAN_POINT('Origin',(11.4022814987,-32.6742356128,7.54785992694));
#55032=CARTESIAN_POINT('Origin',(11.4022814987,-32.8742356128,7.54785992694));
#55033=CARTESIAN_POINT('Origin',(7.97551483927,-32.6742356128,11.0631423009));
#55034=CARTESIAN_POINT('',(6.92846389685,-32.8742356128,12.1372392817));
#55035=CARTESIAN_POINT('Origin',(7.97551483927,-32.8742356128,11.0631423009));
#55036=CARTESIAN_POINT('',(6.92846389685,-33.6742356128,12.1372392817));
#55037=CARTESIAN_POINT('Origin',(6.92846389685,-32.4742356128,12.1372392817));
#55038=CARTESIAN_POINT('',(7.24427528424,-32.8742356128,12.4450984571));
#55039=CARTESIAN_POINT('',(6.92846389685,-32.8742356128,12.1372392817));
#55040=CARTESIAN_POINT('',(7.24427528424,-33.6742356128,12.4450984571));
#55041=CARTESIAN_POINT('Origin',(-1.09995011675E-15,-34.4242356128,2.38806125834E-16));
#55042=CARTESIAN_POINT('',(-6.7887641255,-32.8742356128,12.6993181568));
#55043=CARTESIAN_POINT('Origin',(5.21804821573824E-14,-32.8742356128,8.88178419700125E-15));
#55044=CARTESIAN_POINT('',(-6.7887641255,-33.6742356128,12.6993181568));
#55045=CARTESIAN_POINT('Origin',(-6.92846389685,-32.4742356128,-12.1372392817));
#55046=CARTESIAN_POINT('',(-6.92846389685,-32.8742356128,-12.1372392817));
#55047=CARTESIAN_POINT('',(-6.92846389685,-32.6742356128,-12.1372392817));
#55048=CARTESIAN_POINT('',(-6.92846389685,-32.8742356128,-12.1372392817));
#55049=CARTESIAN_POINT('Origin',(-7.97551483927,-32.6742356128,-11.0631423009));
#55050=CARTESIAN_POINT('',(-6.90141785854,-32.8742356128,-10.0160913585));
#55051=CARTESIAN_POINT('Origin',(-7.97551483927,-32.8742356128,-11.0631423009));
#55052=CARTESIAN_POINT('',(-6.90141785854,-33.6742356128,-10.0160913585));
#55053=CARTESIAN_POINT('Origin',(-10.328184518,-32.4742356128,-6.50080898452));
#55054=CARTESIAN_POINT('',(-10.328184518,-32.8742356128,-6.50080898452));
#55055=CARTESIAN_POINT('',(-10.328184518,-32.6742356128,-6.50080898452));
#55056=CARTESIAN_POINT('',(-10.328184518,-32.8742356128,-6.50080898452));
#55057=CARTESIAN_POINT('Origin',(-11.7522975715,-32.6742356128,7.18880270079));
#55058=CARTESIAN_POINT('',(-10.6782005908,-32.8742356128,6.14175175838));
#55059=CARTESIAN_POINT('Origin',(-11.7522975715,-32.8742356128,7.18880270079));
#55060=CARTESIAN_POINT('',(-10.6782005908,-33.6742356128,6.14175175838));
#55061=CARTESIAN_POINT('Origin',(-10.328184518,-32.4742356128,6.50080898452));
#55062=CARTESIAN_POINT('',(-6.55240087774,-32.8742356128,10.3741236854));
#55063=CARTESIAN_POINT('',(-6.55240087774,-32.6742356128,10.3741236854));
#55064=CARTESIAN_POINT('',(-10.6782005908,-32.8742356128,6.14175175838));
#55065=CARTESIAN_POINT('Origin',(-7.62649785846,-32.6742356128,11.4211746278));
#55066=CARTESIAN_POINT('',(-6.57944691605,-32.8742356128,12.4952716086));
#55067=CARTESIAN_POINT('Origin',(-7.62649785846,-32.8742356128,11.4211746278));
#55068=CARTESIAN_POINT('',(-6.57944691605,-32.6742356128,12.4952716086));
#55069=CARTESIAN_POINT('Origin',(-6.57944691605,-32.4742356128,12.4952716086));
#55070=CARTESIAN_POINT('',(-6.57944691605,-32.8742356128,12.4952716086));
#55071=CARTESIAN_POINT('Ctrl Pts',(1.68475792039,-35.3742356128,-5.03973467448));
#55072=CARTESIAN_POINT('Ctrl Pts',(0.682166339124,-32.4742356128,-4.8790713724));
#55073=CARTESIAN_POINT('Ctrl Pts',(2.15538022242,-35.3742356128,-4.8080213959));
#55074=CARTESIAN_POINT('Ctrl Pts',(1.20736921572,-32.4742356128,-4.44659694115));
#55075=CARTESIAN_POINT('Ctrl Pts',(2.59973387128,-35.3742356128,-4.50528924317));
#55076=CARTESIAN_POINT('Ctrl Pts',(1.71079094607,-32.4742356128,-4.00290111016));
#55077=CARTESIAN_POINT('Ctrl Pts',(2.98121657961,-35.3742356128,-4.12686323533));
#55078=CARTESIAN_POINT('Ctrl Pts',(2.19825830329,-32.4742356128,-3.54512092123));
#55079=CARTESIAN_POINT('Ctrl Pts',(3.28679922947,-35.3742356128,-3.68411804659));
#55080=CARTESIAN_POINT('Ctrl Pts',(2.67474264449,-32.4742356128,-3.06699209341));
#55081=CARTESIAN_POINT('Ctrl Pts',(3.51985615629,-35.3742356128,-3.20601908088));
#55082=CARTESIAN_POINT('Ctrl Pts',(3.1350457731,-32.4742356128,-2.57376246377));
#55083=CARTESIAN_POINT('',(0.682166339124,-32.4742356128,-4.8790713724));
#55084=CARTESIAN_POINT('',(1.65073607089,-35.2758272825,-5.03428274092));
#55085=CARTESIAN_POINT('',(3.1350457731,-32.4742356128,-2.57376246377));
#55086=CARTESIAN_POINT('Ctrl Pts',(3.1350457731,-32.4742356128,-2.57376246377));
#55087=CARTESIAN_POINT('Ctrl Pts',(3.04574386842478,-32.4742356128,-2.66945233123215));
#55088=CARTESIAN_POINT('Ctrl Pts',(2.95565520899676,-32.4742356128,-2.76451972688002));
#55089=CARTESIAN_POINT('Ctrl Pts',(2.86486097840212,-32.4742356128,-2.85887905523607));
#55090=CARTESIAN_POINT('Ctrl Pts',(2.76926551199805,-32.4742356128,-2.95822814321991));
#55091=CARTESIAN_POINT('Ctrl Pts',(2.67288792014402,-32.4742356128,-3.05679239893703));
#55092=CARTESIAN_POINT('Ctrl Pts',(2.57578459070286,-32.4742356128,-3.15451622941541));
#55093=CARTESIAN_POINT('Ctrl Pts',(2.47439813201672,-32.4742356128001,-3.25655055880935));
#55094=CARTESIAN_POINT('Ctrl Pts',(2.37222039913981,-32.4742356128001,-3.35766900818225));
#55095=CARTESIAN_POINT('Ctrl Pts',(2.2692753175773,-32.4742356128001,-3.45785202544386));
#55096=CARTESIAN_POINT('Ctrl Pts',(2.16032661276555,-32.4742356128001,-3.56387758595748));
#55097=CARTESIAN_POINT('Ctrl Pts',(2.05051830060976,-32.4742356128001,-3.66885589509191));
#55098=CARTESIAN_POINT('Ctrl Pts',(1.93983639318639,-32.4742356128001,-3.77280566427766));
#55099=CARTESIAN_POINT('Ctrl Pts',(1.81352928403153,-32.4742356128001,-3.89143024483304));
#55100=CARTESIAN_POINT('Ctrl Pts',(1.68608466211416,-32.4742356128001,-4.00871596374921));
#55101=CARTESIAN_POINT('Ctrl Pts',(1.55742711564637,-32.4742356128001,-4.1247361422481));
#55102=CARTESIAN_POINT('Ctrl Pts',(1.40954803390843,-32.4742356128001,-4.25808982363347));
#55103=CARTESIAN_POINT('Ctrl Pts',(1.26006594487636,-32.4742356128001,-4.38977385603739));
#55104=CARTESIAN_POINT('Ctrl Pts',(1.10880104134623,-32.4742356128001,-4.51993332529904));
#55105=CARTESIAN_POINT('Ctrl Pts',(0.968189500144993,-32.4742356128001,
-4.64092585659807));
#55106=CARTESIAN_POINT('Ctrl Pts',(0.826035174351419,-32.4742356128001,
-4.760603642191));
#55107=CARTESIAN_POINT('Ctrl Pts',(0.682166339124,-32.4742356128,-4.8790713724));
#55108=CARTESIAN_POINT('',(3.50597895501,-35.2696545374,-3.18321836469));
#55109=CARTESIAN_POINT('Ctrl Pts',(1.51727342606,-35.3742356128,-5.3088808072));
#55110=CARTESIAN_POINT('Ctrl Pts',(0.5,-32.4742356128,-5.26505293156));
#55111=CARTESIAN_POINT('Ctrl Pts',(1.51727346704,-35.3742356128,-5.24111839755));
#55112=CARTESIAN_POINT('Ctrl Pts',(0.49999996933,-32.4742356128,-5.17707576222));
#55113=CARTESIAN_POINT('Ctrl Pts',(1.53640667867,-35.3742356128,-5.1734830193));
#55114=CARTESIAN_POINT('Ctrl Pts',(0.519349085752,-32.4742356128,-5.08894068096));
#55115=CARTESIAN_POINT('Ctrl Pts',(1.57167084987,-35.3742356128,-5.11676901693));
#55116=CARTESIAN_POINT('Ctrl Pts',(0.558553592228,-32.4742356128,-5.00590412413));
#55117=CARTESIAN_POINT('Ctrl Pts',(1.62392373781,-35.3742356128,-5.06968674937));
#55118=CARTESIAN_POINT('Ctrl Pts',(0.614278309582,-32.4742356128,-4.93497322721));
#55119=CARTESIAN_POINT('Ctrl Pts',(1.68475792039,-35.3742356128,-5.03973467448));
#55120=CARTESIAN_POINT('Ctrl Pts',(0.682166339124,-32.4742356128,-4.8790713724));
#55121=CARTESIAN_POINT('',(0.5,-32.4742356128,-5.26505293156));
#55122=CARTESIAN_POINT('',(1.46090316329,-35.2135376551,-5.30645216923));
#55123=CARTESIAN_POINT('Ctrl Pts',(0.5,-32.4742356128,-5.26505293156));
#55124=CARTESIAN_POINT('Ctrl Pts',(0.499999987183553,-32.4742356128,-5.22828883820323));
#55125=CARTESIAN_POINT('Ctrl Pts',(0.504054600653073,-32.4742356128085,
-5.19170069064497));
#55126=CARTESIAN_POINT('Ctrl Pts',(0.520156709880915,-32.4742356128085,
-5.1199141043431));
#55127=CARTESIAN_POINT('Ctrl Pts',(0.532168073174417,-32.4742356128085,
-5.08496970255448));
#55128=CARTESIAN_POINT('Ctrl Pts',(0.56359844412932,-32.4742356128085,-5.0183737839542));
#55129=CARTESIAN_POINT('Ctrl Pts',(0.582941481982889,-32.4742356128085,
-4.98688524144264));
#55130=CARTESIAN_POINT('Ctrl Pts',(0.628123824966223,-32.4742356128085,
-4.9288235651309));
#55131=CARTESIAN_POINT('Ctrl Pts',(0.653788606277979,-32.4742356128,-4.90243878948513));
#55132=CARTESIAN_POINT('Ctrl Pts',(0.682166339124,-32.4742356128,-4.8790713724));
#55133=CARTESIAN_POINT('Origin',(1.51727342606,-35.3742356128,-6.62635333853281));
#55134=CARTESIAN_POINT('',(0.5,-32.4742356128,-8.63648038577));
#55135=CARTESIAN_POINT('',(1.46144758302801,-35.2150896637902,-7.9872159496586));
#55136=CARTESIAN_POINT('',(0.5,-32.4742356128,-5.26505293156));
#55137=CARTESIAN_POINT('Ctrl Pts',(2.06618662358,-35.3742356128,-8.20763292551));
#55138=CARTESIAN_POINT('Ctrl Pts',(1.13092983125,-32.4742356128,-9.11903336658));
#55139=CARTESIAN_POINT('Ctrl Pts',(2.02728693019,-35.3742356128,-8.21539237438));
#55140=CARTESIAN_POINT('Ctrl Pts',(1.08254865919,-32.4742356128,-9.13216050293));
#55141=CARTESIAN_POINT('Ctrl Pts',(1.98835267261,-35.3742356128,-8.22296816028));
#55142=CARTESIAN_POINT('Ctrl Pts',(1.03251986746,-32.4742356128,-9.13922496193));
#55143=CARTESIAN_POINT('Ctrl Pts',(1.94830447917,-35.3742356128,-8.23056358523));
#55144=CARTESIAN_POINT('Ctrl Pts',(0.980045978296,-32.4742356128,-9.13989363405));
#55145=CARTESIAN_POINT('Ctrl Pts',(1.90939289225,-35.3742356128,-8.23775490438));
#55146=CARTESIAN_POINT('Ctrl Pts',(0.929775106566,-32.4742356128,-9.13406227499));
#55147=CARTESIAN_POINT('Ctrl Pts',(1.87043161103,-35.3742356128,-8.24476960824));
#55148=CARTESIAN_POINT('Ctrl Pts',(0.881024471639,-32.4742356128,-9.12211895883));
#55149=CARTESIAN_POINT('',(1.13092983125,-32.4742356128,-9.11903336658));
#55150=CARTESIAN_POINT('',(2.02882173043,-35.2583763205,-8.24404472212));
#55151=CARTESIAN_POINT('',(0.881024471639,-32.4742356128,-9.12211895883));
#55152=CARTESIAN_POINT('Ctrl Pts',(0.881024471639,-32.4742356128,-9.12211895883));
#55153=CARTESIAN_POINT('Ctrl Pts',(0.922203022128766,-32.4742356128,-9.13220720584968));
#55154=CARTESIAN_POINT('Ctrl Pts',(0.964264761466657,-32.4742356129145,
-9.13687601608875));
#55155=CARTESIAN_POINT('Ctrl Pts',(1.04807643550279,-32.4742356129145,-9.13584111848088));
#55156=CARTESIAN_POINT('Ctrl Pts',(1.09001173360473,-32.4742356128,-9.13013556654957));
#55157=CARTESIAN_POINT('Ctrl Pts',(1.13092983125,-32.4742356128,-9.11903336658));
#55158=CARTESIAN_POINT('',(1.83110005118,-35.2589529157,-8.27964657357));
#55159=CARTESIAN_POINT('Ctrl Pts',(1.87043161103,-35.3742356128,-8.24476960824));
#55160=CARTESIAN_POINT('Ctrl Pts',(0.881024471639,-32.4742356128,-9.12211895883));
#55161=CARTESIAN_POINT('Ctrl Pts',(1.76698369017,-35.3742356128,-8.26339468616));
#55162=CARTESIAN_POINT('Ctrl Pts',(0.751586859387,-32.4742356128,-9.0904082994));
#55163=CARTESIAN_POINT('Ctrl Pts',(1.65525765665,-35.3742356128,-8.23673498884));
#55164=CARTESIAN_POINT('Ctrl Pts',(0.632864708596,-32.4742356128,-9.01561057704));
#55165=CARTESIAN_POINT('Ctrl Pts',(1.56310817921,-35.3742356128,-8.15928174403));
#55166=CARTESIAN_POINT('Ctrl Pts',(0.544519454171,-32.4742356128,-8.90337130527));
#55167=CARTESIAN_POINT('Ctrl Pts',(1.51727343488,-35.3742356128,-8.05439924541));
#55168=CARTESIAN_POINT('Ctrl Pts',(0.500000005883,-32.4742356128,-8.76992589769));
#55169=CARTESIAN_POINT('Ctrl Pts',(1.51727342606,-35.3742356128,-7.9495168227));
#55170=CARTESIAN_POINT('Ctrl Pts',(0.5,-32.4742356128,-8.63648038577));
#55171=CARTESIAN_POINT('Ctrl Pts',(0.881024471639,-32.4742356128,-9.12211895883));
#55172=CARTESIAN_POINT('Ctrl Pts',(0.827016089126107,-32.4742356128,-9.10888755418313));
#55173=CARTESIAN_POINT('Ctrl Pts',(0.775540637915395,-32.4742356128,-9.08673032516009));
#55174=CARTESIAN_POINT('Ctrl Pts',(0.682134270020786,-32.4742356128,-9.02649837726588));
#55175=CARTESIAN_POINT('Ctrl Pts',(0.640813901103346,-32.4742356141908,
-8.98885840070038));
#55176=CARTESIAN_POINT('Ctrl Pts',(0.57228055336198,-32.4742356141908,-8.901510263898));
#55177=CARTESIAN_POINT('Ctrl Pts',(0.545563385694432,-32.4742356128,-8.85244719394298));
#55178=CARTESIAN_POINT('Ctrl Pts',(0.509276617611064,-32.4742356128,-8.74739553291418));
#55179=CARTESIAN_POINT('Ctrl Pts',(0.500000002452142,-32.4742356128,-8.69210290609089));
#55180=CARTESIAN_POINT('Ctrl Pts',(0.5,-32.4742356128,-8.63648038577));
#55181=CARTESIAN_POINT('Ctrl Pts',(8.90408048591,-35.3742356128,-3.33175685019));
#55182=CARTESIAN_POINT('Ctrl Pts',(9.78972512979,-32.4742356128,-2.88747118331));
#55183=CARTESIAN_POINT('Ctrl Pts',(8.6873937464,-35.3742356128,-3.78156218415));
#55184=CARTESIAN_POINT('Ctrl Pts',(9.44154892618,-32.4742356128,-3.40960230403));
#55185=CARTESIAN_POINT('Ctrl Pts',(8.41228804471,-35.3742356128,-4.20311089247));
#55186=CARTESIAN_POINT('Ctrl Pts',(9.06633060557,-32.4742356128,-3.9138589137));
#55187=CARTESIAN_POINT('Ctrl Pts',(8.09063109224,-35.3742356128,-4.59678365893));
#55188=CARTESIAN_POINT('Ctrl Pts',(8.6592141531,-32.4742356128,-4.40538764451));
#55189=CARTESIAN_POINT('Ctrl Pts',(7.360622472,-35.3742356128,-5.38465519647));
#55190=CARTESIAN_POINT('Ctrl Pts',(7.74414150515,-32.4742356128,-5.40001779324));
#55191=CARTESIAN_POINT('Ctrl Pts',(6.54392160985,-35.3742356128,-6.08248533528));
#55192=CARTESIAN_POINT('Ctrl Pts',(6.72376489891,-32.4742356128,-6.28784412471));
#55193=CARTESIAN_POINT('Ctrl Pts',(6.08996440487,-35.3742356128,-6.43395446983));
#55194=CARTESIAN_POINT('Ctrl Pts',(6.15045388192,-32.4742356128,-6.72961730824));
#55195=CARTESIAN_POINT('Ctrl Pts',(5.07098217764,-35.3742356128,-7.12903795521));
#55196=CARTESIAN_POINT('Ctrl Pts',(4.8659622122,-32.4742356128,-7.60280558321));
#55197=CARTESIAN_POINT('Ctrl Pts',(3.96068628695,-35.3742356128,-7.66774624913));
#55198=CARTESIAN_POINT('Ctrl Pts',(3.47975995949,-32.4742356128,-8.30623076748));
#55199=CARTESIAN_POINT('Ctrl Pts',(3.34362139801,-35.3742356128,-7.90067576649));
#55200=CARTESIAN_POINT('Ctrl Pts',(2.71614717835,-32.4742356128,-8.63027694049));
#55201=CARTESIAN_POINT('Ctrl Pts',(2.70966555084,-35.3742356128,-8.07927608136));
#55202=CARTESIAN_POINT('Ctrl Pts',(1.93124535238,-32.4742356128,-8.90188586102));
#55203=CARTESIAN_POINT('Ctrl Pts',(2.06618662358,-35.3742356128,-8.20763292551));
#55204=CARTESIAN_POINT('Ctrl Pts',(1.13092983125,-32.4742356128,-9.11903336658));
#55205=CARTESIAN_POINT('',(9.78972512979,-32.4742356128,-2.88747118331));
#55206=CARTESIAN_POINT('',(8.93444623808,-35.2748044449,-3.31652380097));
#55207=CARTESIAN_POINT('Ctrl Pts',(1.13092983125,-32.4742356128,-9.11903336658));
#55208=CARTESIAN_POINT('Ctrl Pts',(1.35748096440087,-32.4742356128002,-9.05756384343984));
#55209=CARTESIAN_POINT('Ctrl Pts',(1.58257164660585,-32.4742356128003,-8.99085150410091));
#55210=CARTESIAN_POINT('Ctrl Pts',(1.80593829563056,-32.4742356128004,-8.91898444731663));
#55211=CARTESIAN_POINT('Ctrl Pts',(2.06358605409587,-32.4742356128005,-8.83608762199012));
#55212=CARTESIAN_POINT('Ctrl Pts',(2.31894092044636,-32.4742356128005,-8.74633156326516));
#55213=CARTESIAN_POINT('Ctrl Pts',(2.57167018297851,-32.4742356128005,-8.6498360378973));
#55214=CARTESIAN_POINT('Ctrl Pts',(2.87961762633398,-32.4742356128005,-8.53225744792893));
#55215=CARTESIAN_POINT('Ctrl Pts',(3.18367140744747,-32.4742356128005,-8.40466930268279));
#55216=CARTESIAN_POINT('Ctrl Pts',(3.48328763307677,-32.4742356128004,-8.26730091093105));
#55217=CARTESIAN_POINT('Ctrl Pts',(3.71568832582298,-32.4742356128003,-8.16074957400834));
#55218=CARTESIAN_POINT('Ctrl Pts',(3.94542176433015,-32.4742356128003,-8.0483135945673));
#55219=CARTESIAN_POINT('Ctrl Pts',(4.17221459820387,-32.4742356128002,-7.93012756314153));
#55220=CARTESIAN_POINT('Ctrl Pts',(4.3691051862723,-32.4742356128002,-7.82752415706631));
#55221=CARTESIAN_POINT('Ctrl Pts',(4.56378009094538,-32.4742356128001,-7.72058696590365));
#55222=CARTESIAN_POINT('Ctrl Pts',(4.75602733655703,-32.4742356128001,-7.60942955096299));
#55223=CARTESIAN_POINT('Ctrl Pts',(4.81482808842437,-32.4742356128001,-7.57543093863777));
#55224=CARTESIAN_POINT('Ctrl Pts',(4.87340144129883,-32.4742356128001,-7.54103772494405));
#55225=CARTESIAN_POINT('Ctrl Pts',(4.93174048144869,-32.4742356128001,-7.50625373162201));
#55226=CARTESIAN_POINT('Ctrl Pts',(5.17371609272893,-32.4742356128,-7.36197850828535));
#55227=CARTESIAN_POINT('Ctrl Pts',(5.41165903155182,-32.4742356128,-7.21097959772054));
#55228=CARTESIAN_POINT('Ctrl Pts',(5.64521361977431,-32.4742356128,-7.0534854983882));
#55229=CARTESIAN_POINT('Ctrl Pts',(5.92854786582719,-32.4742356128,-6.86242321940786));
#55230=CARTESIAN_POINT('Ctrl Pts',(6.20541886627958,-32.4742356128,-6.66180293529635));
#55231=CARTESIAN_POINT('Ctrl Pts',(6.47520523011177,-32.4742356128,-6.45207607376425));
#55232=CARTESIAN_POINT('Ctrl Pts',(6.7042174903774,-32.4742356128001,-6.27404623594872));
#55233=CARTESIAN_POINT('Ctrl Pts',(6.92812568553406,-32.4742356128001,-6.08945471655604));
#55234=CARTESIAN_POINT('Ctrl Pts',(7.14656401932481,-32.4742356128001,-5.89860434351618));
#55235=CARTESIAN_POINT('Ctrl Pts',(7.30145174556248,-32.4742356128002,-5.76327836927544));
#55236=CARTESIAN_POINT('Ctrl Pts',(7.4535896236381,-32.4742356128002,-5.62480608682023));
#55237=CARTESIAN_POINT('Ctrl Pts',(7.60284952378423,-32.4742356128003,-5.48330473081067));
#55238=CARTESIAN_POINT('Ctrl Pts',(7.66409102798865,-32.4742356128003,-5.42524656595522));
#55239=CARTESIAN_POINT('Ctrl Pts',(7.72484844931582,-32.4742356128003,-5.36667817449847));
#55240=CARTESIAN_POINT('Ctrl Pts',(7.78511221664714,-32.4742356128003,-5.30760881482714));
#55241=CARTESIAN_POINT('Ctrl Pts',(7.86083082414573,-32.4742356128003,-5.23339092473813));
#55242=CARTESIAN_POINT('Ctrl Pts',(7.9357705171939,-32.4742356128004,-5.1583808441567));
#55243=CARTESIAN_POINT('Ctrl Pts',(8.00994285087825,-32.4742356128004,-5.08255688170474));
#55244=CARTESIAN_POINT('Ctrl Pts',(8.09229096248547,-32.4742356128004,-4.99837508759984));
#55245=CARTESIAN_POINT('Ctrl Pts',(8.17369314495629,-32.4742356128004,-4.91319009037416));
#55246=CARTESIAN_POINT('Ctrl Pts',(8.25412492760548,-32.4742356128004,-4.82702704996663));
#55247=CARTESIAN_POINT('Ctrl Pts',(8.31333790947206,-32.4742356128004,-4.76359478002089));
#55248=CARTESIAN_POINT('Ctrl Pts',(8.37202401218054,-32.4742356128004,-4.69963371548019));
#55249=CARTESIAN_POINT('Ctrl Pts',(8.43016285000587,-32.4742356128004,-4.63516899165583));
#55250=CARTESIAN_POINT('Ctrl Pts',(8.45791646133128,-32.4742356128004,-4.60439560580666));
#55251=CARTESIAN_POINT('Ctrl Pts',(8.48554521988306,-32.4742356128004,-4.57350770746612));
#55252=CARTESIAN_POINT('Ctrl Pts',(8.51305689825755,-32.4742356128004,-4.54249677272974));
#55253=CARTESIAN_POINT('Ctrl Pts',(8.62342507636421,-32.4742356128004,-4.41809068155457));
#55254=CARTESIAN_POINT('Ctrl Pts',(8.7318733436495,-32.4742356128004,-4.29174315144362));
#55255=CARTESIAN_POINT('Ctrl Pts',(8.8382486463566,-32.4742356128004,-4.16363335145393));
#55256=CARTESIAN_POINT('Ctrl Pts',(8.93277342320662,-32.4742356128004,-4.04979536511541));
#55257=CARTESIAN_POINT('Ctrl Pts',(9.02565819435723,-32.4742356128005,-3.93456977982075));
#55258=CARTESIAN_POINT('Ctrl Pts',(9.11679326953606,-32.4742356128005,-3.81808802140576));
#55259=CARTESIAN_POINT('Ctrl Pts',(9.19450142462868,-32.4742356128005,-3.7187675069868));
#55260=CARTESIAN_POINT('Ctrl Pts',(9.2709365589139,-32.4742356128005,-3.61853483930442));
#55261=CARTESIAN_POINT('Ctrl Pts',(9.34605185297795,-32.4742356128005,-3.51744756155323));
#55262=CARTESIAN_POINT('Ctrl Pts',(9.41503263776077,-32.4742356128005,-3.42461587078078));
#55263=CARTESIAN_POINT('Ctrl Pts',(9.48289988060696,-32.4742356128004,-3.33106404763001));
#55264=CARTESIAN_POINT('Ctrl Pts',(9.54964545463381,-32.4742356128004,-3.23680385237855));
#55265=CARTESIAN_POINT('Ctrl Pts',(9.6112390224299,-32.4742356128003,-3.14981948208372));
#55266=CARTESIAN_POINT('Ctrl Pts',(9.67187720579196,-32.4742356128002,-3.0622321188807));
#55267=CARTESIAN_POINT('Ctrl Pts',(9.73158294374893,-32.4742356128001,-2.97401646795334));
#55268=CARTESIAN_POINT('Ctrl Pts',(9.75106213192314,-32.4742356128001,-2.94523582938955));
#55269=CARTESIAN_POINT('Ctrl Pts',(9.77044232827666,-32.4742356128,-2.91638800950429));
#55270=CARTESIAN_POINT('Ctrl Pts',(9.78972512979,-32.4742356128,-2.88747118331));
#55271=CARTESIAN_POINT('Ctrl Pts',(8.98669828191,-35.3742356128,-3.15062625521));
#55272=CARTESIAN_POINT('Ctrl Pts',(9.87176476169,-32.4742356128,-2.65438916225));
#55273=CARTESIAN_POINT('Ctrl Pts',(8.97105229548,-35.3742356128,-3.18695239061));
#55274=CARTESIAN_POINT('Ctrl Pts',(9.86736571705,-32.4742356128,-2.70382530588));
#55275=CARTESIAN_POINT('Ctrl Pts',(8.95501903475,-35.3742356128,-3.22311199053));
#55276=CARTESIAN_POINT('Ctrl Pts',(9.85683264819,-32.4742356128,-2.75271530399));
#55277=CARTESIAN_POINT('Ctrl Pts',(8.93801024352,-35.3742356128,-3.26038797601));
#55278=CARTESIAN_POINT('Ctrl Pts',(9.83970156009,-32.4742356128,-2.80141079064));
#55279=CARTESIAN_POINT('Ctrl Pts',(8.92122822926,-35.3742356128,-3.29616101079));
#55280=CARTESIAN_POINT('Ctrl Pts',(9.81727888481,-32.4742356128,-2.84615108413));
#55281=CARTESIAN_POINT('Ctrl Pts',(8.90408048591,-35.3742356128,-3.33175685019));
#55282=CARTESIAN_POINT('Ctrl Pts',(9.78972512979,-32.4742356128,-2.88747118331));
#55283=CARTESIAN_POINT('',(9.87176476169,-32.4742356128,-2.65438916225));
#55284=CARTESIAN_POINT('',(9.01911869317,-35.2680072167,-3.13244885159));
#55285=CARTESIAN_POINT('Ctrl Pts',(9.78972512979,-32.4742356128,-2.88747118331));
#55286=CARTESIAN_POINT('Ctrl Pts',(9.81295259231924,-32.4742356128,-2.85263886899527));
#55287=CARTESIAN_POINT('Ctrl Pts',(9.83153875118569,-32.4742356128031,-2.81516874103241));
#55288=CARTESIAN_POINT('Ctrl Pts',(9.85907250604964,-32.4742356128031,-2.7369427732809));
#55289=CARTESIAN_POINT('Ctrl Pts',(9.86805391811268,-32.4742356128,-2.69609135240486));
#55290=CARTESIAN_POINT('Ctrl Pts',(9.87176476169,-32.4742356128,-2.65438916225));
#55291=CARTESIAN_POINT('Ctrl Pts',(9.23698117862,-35.3742356128,0.509886547139));
#55292=CARTESIAN_POINT('Ctrl Pts',(9.85462053301,-32.4742356128,2.00920484002));
#55293=CARTESIAN_POINT('Ctrl Pts',(9.29448486778,-35.3742356128,0.14300248283));
#55294=CARTESIAN_POINT('Ctrl Pts',(9.89942675021,-32.4742356128,1.54440936128));
#55295=CARTESIAN_POINT('Ctrl Pts',(9.33952412131,-35.3742356128,-0.225988266205));
#55296=CARTESIAN_POINT('Ctrl Pts',(9.93347655148,-32.4742356128,1.07876884298));
#55297=CARTESIAN_POINT('Ctrl Pts',(9.37147906182,-35.3742356128,-0.598052135313));
#55298=CARTESIAN_POINT('Ctrl Pts',(9.95684539874,-32.4742356128,0.6105872463));
#55299=CARTESIAN_POINT('Ctrl Pts',(9.39776085185,-35.3742356128,-1.34354990637));
#55300=CARTESIAN_POINT('Ctrl Pts',(9.98182966629,-32.4742356128,-0.323612218818));
#55301=CARTESIAN_POINT('Ctrl Pts',(9.31944120585,-35.3742356128,-2.08553948714));
#55302=CARTESIAN_POINT('Ctrl Pts',(9.96363436978,-32.4742356128,-1.25779968708));
#55303=CARTESIAN_POINT('Ctrl Pts',(9.24709061054,-35.3742356128,-2.45151005123));
#55304=CARTESIAN_POINT('Ctrl Pts',(9.943864011,-32.4742356128,-1.72215443881));
#55305=CARTESIAN_POINT('Ctrl Pts',(9.13406983882,-35.3742356128,-2.80846571914));
#55306=CARTESIAN_POINT('Ctrl Pts',(9.91319925962,-32.4742356128,-2.18875096266));
#55307=CARTESIAN_POINT('Ctrl Pts',(8.98669828191,-35.3742356128,-3.15062625521));
#55308=CARTESIAN_POINT('Ctrl Pts',(9.87176476169,-32.4742356128,-2.65438916225));
#55309=CARTESIAN_POINT('',(9.85462053301,-32.4742356128,2.00920484002));
#55310=CARTESIAN_POINT('',(9.26569107792,-35.2394341184,0.579579770069));
#55311=CARTESIAN_POINT('Ctrl Pts',(9.87176476169,-32.4742356128,-2.65438916225));
#55312=CARTESIAN_POINT('Ctrl Pts',(9.88154386677506,-32.4742356128,-2.54449221374346));
#55313=CARTESIAN_POINT('Ctrl Pts',(9.89059756234382,-32.4742356128,-2.43459652045344));
#55314=CARTESIAN_POINT('Ctrl Pts',(9.8989264871901,-32.4742356128,-2.32475313888866));
#55315=CARTESIAN_POINT('Ctrl Pts',(9.9081500912099,-32.4742356128,-2.20311056503328));
#55316=CARTESIAN_POINT('Ctrl Pts',(9.91648489987761,-32.4742356128,-2.08153136407751));
#55317=CARTESIAN_POINT('Ctrl Pts',(9.92393401731845,-32.4742356128,-1.96001454973233));
#55318=CARTESIAN_POINT('Ctrl Pts',(9.93353796504327,-32.4742356128,-1.80334617365589));
#55319=CARTESIAN_POINT('Ctrl Pts',(9.94166984694101,-32.4742356128,-1.64677964259028));
#55320=CARTESIAN_POINT('Ctrl Pts',(9.94833842889768,-32.4742356128,-1.49021719058124));
#55321=CARTESIAN_POINT('Ctrl Pts',(9.95450935391368,-32.4742356128,-1.34533854052529));
#55322=CARTESIAN_POINT('Ctrl Pts',(9.95942746092287,-32.4742356128,-1.20045751698348));
#55323=CARTESIAN_POINT('Ctrl Pts',(9.96309809061568,-32.4742356128,-1.05549464624314));
#55324=CARTESIAN_POINT('Ctrl Pts',(9.96618761475916,-32.4742356128,-0.933481169934575));
#55325=CARTESIAN_POINT('Ctrl Pts',(9.96839341766342,-32.4742356128,-0.811408131094685));
#55326=CARTESIAN_POINT('Ctrl Pts',(9.96971606220048,-32.4742356128,-0.689268635606535));
#55327=CARTESIAN_POINT('Ctrl Pts',(9.97087661179947,-32.4742356128,-0.582097783168821));
#55328=CARTESIAN_POINT('Ctrl Pts',(9.97135721001099,-32.4742356128,-0.474875416188859));
#55329=CARTESIAN_POINT('Ctrl Pts',(9.9711558159983,-32.4742356128,-0.367641445316077));
#55330=CARTESIAN_POINT('Ctrl Pts',(9.97112768712725,-32.4742356128,-0.352663986460755));
#55331=CARTESIAN_POINT('Ctrl Pts',(9.97108624965007,-32.4742356128,-0.337686384785283));
#55332=CARTESIAN_POINT('Ctrl Pts',(9.97103149360754,-32.4742356128,-0.322708834412021));
#55333=CARTESIAN_POINT('Ctrl Pts',(9.97058233383006,-32.4742356128,-0.199849093595623));
#55334=CARTESIAN_POINT('Ctrl Pts',(9.96923674804115,-32.4742356128,-0.0769878672143817));
#55335=CARTESIAN_POINT('Ctrl Pts',(9.96699184142756,-32.4742356128,0.045914908526925));
#55336=CARTESIAN_POINT('Ctrl Pts',(9.96446705860022,-32.4742356128,0.18414017622627));
#55337=CARTESIAN_POINT('Ctrl Pts',(9.96080479842082,-32.4742356128,0.322417042225777));
#55338=CARTESIAN_POINT('Ctrl Pts',(9.95600414301969,-32.4742356128,0.46073214033741));
#55339=CARTESIAN_POINT('Ctrl Pts',(9.94704210756475,-32.4742356128,0.718943719727021));
#55340=CARTESIAN_POINT('Ctrl Pts',(9.93411358948493,-32.4742356128,0.9772793342408));
#55341=CARTESIAN_POINT('Ctrl Pts',(9.91721974812435,-32.4742356128,1.23541623248458));
#55342=CARTESIAN_POINT('Ctrl Pts',(9.90877282744406,-32.4742356128,1.36448468160648));
#55343=CARTESIAN_POINT('Ctrl Pts',(9.89933452477601,-32.4742356128,1.4935023352826));
#55344=CARTESIAN_POINT('Ctrl Pts',(9.88890261150967,-32.4742356128,1.62246096624871));
#55345=CARTESIAN_POINT('Ctrl Pts',(9.87934749865317,-32.4742356128,1.74058064777235));
#55346=CARTESIAN_POINT('Ctrl Pts',(9.86895881847276,-32.4742356128,1.85865002300787));
#55347=CARTESIAN_POINT('Ctrl Pts',(9.85773224379276,-32.4742356128,1.97670577301818));
#55348=CARTESIAN_POINT('Ctrl Pts',(9.85670206597819,-32.4742356128,1.98753885594941));
#55349=CARTESIAN_POINT('Ctrl Pts',(9.85566483062434,-32.4742356128,1.99837186102877));
#55350=CARTESIAN_POINT('Ctrl Pts',(9.85462053301,-32.4742356128,2.00920484002));
#55351=CARTESIAN_POINT('Ctrl Pts',(8.75956299023,-35.3742356128,2.0634404101));
#55352=CARTESIAN_POINT('Ctrl Pts',(9.5731487029,-32.4742356128,4.05201631342));
#55353=CARTESIAN_POINT('Ctrl Pts',(8.9288627266048,-35.3742356128,1.78605452583546));
#55354=CARTESIAN_POINT('Ctrl Pts',(9.64554803760896,-32.4742356128,3.64899532239734));
#55355=CARTESIAN_POINT('Ctrl Pts',(9.07284086761294,-35.3742356128,1.49321342917581));
#55356=CARTESIAN_POINT('Ctrl Pts',(9.7097825158037,-32.4742356128,3.24450758797157));
#55357=CARTESIAN_POINT('Ctrl Pts',(9.12665675685958,-35.3742356128,1.15111702356286));
#55358=CARTESIAN_POINT('Ctrl Pts',(9.76785698810379,-32.4742356128,2.82296397732709));
#55359=CARTESIAN_POINT('Ctrl Pts',(9.18661000883968,-35.3742356128,0.831274530260112));
#55360=CARTESIAN_POINT('Ctrl Pts',(9.81537216530061,-32.4742356128,2.41636233386422));
#55361=CARTESIAN_POINT('Ctrl Pts',(9.2369929572006,-35.3742356128,0.509811396507259));
#55362=CARTESIAN_POINT('Ctrl Pts',(9.85462971069928,-32.4742356128,2.00910963374492));
#55363=CARTESIAN_POINT('',(9.5731487029,-32.4742356128,4.05201631342));
#55364=CARTESIAN_POINT('',(8.82321723512,-35.1473421125,2.21902487472));
#55365=CARTESIAN_POINT('Ctrl Pts',(9.5731487029,-32.4742356128,4.05201631342));
#55366=CARTESIAN_POINT('Ctrl Pts',(9.58385803994689,-32.4742356128002,3.99240129558575));
#55367=CARTESIAN_POINT('Ctrl Pts',(9.5943536855861,-32.4742356128003,3.93274277792962));
#55368=CARTESIAN_POINT('Ctrl Pts',(9.60464591256779,-32.4742356128005,3.87295958919005));
#55369=CARTESIAN_POINT('Ctrl Pts',(9.61549552175361,-32.4742356128006,3.80993880322598));
#55370=CARTESIAN_POINT('Ctrl Pts',(9.62611903415596,-32.4742356128007,3.74677981964133));
#55371=CARTESIAN_POINT('Ctrl Pts',(9.63652068269621,-32.4742356128008,3.6834457777419));
#55372=CARTESIAN_POINT('Ctrl Pts',(9.64770872862421,-32.4742356128009,3.61532348281571));
#55373=CARTESIAN_POINT('Ctrl Pts',(9.65864002597334,-32.4742356128009,3.5469991384311));
#55374=CARTESIAN_POINT('Ctrl Pts',(9.66931194496842,-32.4742356128009,3.47848631183157));
#55375=CARTESIAN_POINT('Ctrl Pts',(9.68148004640576,-32.474235612801,3.40036811919857));
#55376=CARTESIAN_POINT('Ctrl Pts',(9.69331083177808,-32.474235612801,3.32200562453762));
#55377=CARTESIAN_POINT('Ctrl Pts',(9.70479179824438,-32.4742356128009,3.24348485468374));
#55378=CARTESIAN_POINT('Ctrl Pts',(9.72018567223827,-32.4742356128009,3.13820287859042));
#55379=CARTESIAN_POINT('Ctrl Pts',(9.73495007583224,-32.4742356128008,3.0326400564569));
#55380=CARTESIAN_POINT('Ctrl Pts',(9.74904466851696,-32.4742356128007,2.92708814611498));
#55381=CARTESIAN_POINT('Ctrl Pts',(9.75943548222612,-32.4742356128006,2.84927318107538));
#55382=CARTESIAN_POINT('Ctrl Pts',(9.76946187459548,-32.4742356128006,2.77146717702865));
#55383=CARTESIAN_POINT('Ctrl Pts',(9.77911025980367,-32.4742356128005,2.69377242009859));
#55384=CARTESIAN_POINT('Ctrl Pts',(9.7877997086789,-32.4742356128004,2.62379961079951));
#55385=CARTESIAN_POINT('Ctrl Pts',(9.79618242234148,-32.4742356128003,2.55391804485846));
#55386=CARTESIAN_POINT('Ctrl Pts',(9.80425367824051,-32.4742356128003,2.484167083785));
#55387=CARTESIAN_POINT('Ctrl Pts',(9.81180034779321,-32.4742356128002,2.41894954381484));
#55388=CARTESIAN_POINT('Ctrl Pts',(9.81907464790267,-32.4742356128002,2.35384679982263));
#55389=CARTESIAN_POINT('Ctrl Pts',(9.82607895911491,-32.4742356128001,2.28884751742804));
#55390=CARTESIAN_POINT('Ctrl Pts',(9.83260578437976,-32.4742356128001,2.22827925515719));
#55391=CARTESIAN_POINT('Ctrl Pts',(9.83889814477805,-32.4742356128,2.1678010763369));
#55392=CARTESIAN_POINT('Ctrl Pts',(9.84496431448895,-32.4742356128,2.10735907911611));
#55393=CARTESIAN_POINT('Ctrl Pts',(9.84824849657925,-32.4742356128,2.07463620220458));
#55394=CARTESIAN_POINT('Ctrl Pts',(9.85146649575577,-32.4742356128,2.04192311779301));
#55395=CARTESIAN_POINT('Ctrl Pts',(9.85462053301,-32.4742356128,2.00920484002));
#55396=CARTESIAN_POINT('Ctrl Pts',(8.51721509197,-35.3742356128,2.41066261776));
#55397=CARTESIAN_POINT('Ctrl Pts',(9.47312185748,-32.4742356128,4.57687569684));
#55398=CARTESIAN_POINT('Ctrl Pts',(8.57124548357,-35.3742356128,2.34542388422));
#55399=CARTESIAN_POINT('Ctrl Pts',(9.49423281845,-32.4742356128,4.47213748961));
#55400=CARTESIAN_POINT('Ctrl Pts',(8.62160287869,-35.3742356128,2.27713826199));
#55401=CARTESIAN_POINT('Ctrl Pts',(9.51478914505,-32.4742356128,4.367292468));
#55402=CARTESIAN_POINT('Ctrl Pts',(8.66952448488,-35.3742356128,2.20708948255));
#55403=CARTESIAN_POINT('Ctrl Pts',(9.53482564259,-32.4742356128,4.26215510362));
#55404=CARTESIAN_POINT('Ctrl Pts',(8.71540499967,-35.3742356128,2.13579061508));
#55405=CARTESIAN_POINT('Ctrl Pts',(9.55426490812,-32.4742356128,4.15713558997));
#55406=CARTESIAN_POINT('Ctrl Pts',(8.75956299023,-35.3742356128,2.0634404101));
#55407=CARTESIAN_POINT('Ctrl Pts',(9.5731487029,-32.4742356128,4.05201631342));
#55408=CARTESIAN_POINT('',(9.47312185748,-32.4742356128,4.57687569684));
#55409=CARTESIAN_POINT('',(8.60091083124725,-35.1203221008745,2.60032840068696));
#55410=CARTESIAN_POINT('Origin',(-15.3007564523972,-32.4742356010378,-0.416450801703818));
#55411=CARTESIAN_POINT('Ctrl Pts',(7.21384189758,-35.3742356128,2.18958432614));
#55412=CARTESIAN_POINT('Ctrl Pts',(7.92659403983,-32.4742356128,4.74000601033));
#55413=CARTESIAN_POINT('Ctrl Pts',(7.26623945249,-35.3742356128,2.28696407666));
#55414=CARTESIAN_POINT('Ctrl Pts',(7.98210778857,-32.4742356128,4.86805404157));
#55415=CARTESIAN_POINT('Ctrl Pts',(7.33077888815,-35.3742356128,2.37781046265));
#55416=CARTESIAN_POINT('Ctrl Pts',(8.06503365985,-32.4742356128,4.98421786182));
#55417=CARTESIAN_POINT('Ctrl Pts',(7.40436869293,-35.3742356128,2.46126398331));
#55418=CARTESIAN_POINT('Ctrl Pts',(8.17216612273,-32.4742356128,5.0807589417));
#55419=CARTESIAN_POINT('Ctrl Pts',(7.56704033307,-35.3742356128,2.61160417272));
#55420=CARTESIAN_POINT('Ctrl Pts',(8.41851793763,-32.4742356128,5.22052728604));
#55421=CARTESIAN_POINT('Ctrl Pts',(7.76385631892,-35.3742356128,2.71310420624));
#55422=CARTESIAN_POINT('Ctrl Pts',(8.70021558456,-32.4742356128,5.24806936162));
#55423=CARTESIAN_POINT('Ctrl Pts',(7.87246551919,-35.3742356128,2.74929666995));
#55424=CARTESIAN_POINT('Ctrl Pts',(8.84211900681,-32.4742356128,5.23137961658));
#55425=CARTESIAN_POINT('Ctrl Pts',(8.09632446877,-35.3742356128,2.75144961057));
#55426=CARTESIAN_POINT('Ctrl Pts',(9.10596900702,-32.4742356128,5.14052628192));
#55427=CARTESIAN_POINT('Ctrl Pts',(8.29201770973,-35.3742356128,2.64306639111));
#55428=CARTESIAN_POINT('Ctrl Pts',(9.31107389815,-32.4742356128,4.95155477014));
#55429=CARTESIAN_POINT('Ctrl Pts',(8.37411601908,-35.3742356128,2.57138954697));
#55430=CARTESIAN_POINT('Ctrl Pts',(9.39185739171,-32.4742356128,4.83723274541));
#55431=CARTESIAN_POINT('Ctrl Pts',(8.4486251678,-35.3742356128,2.49348119172));
#55432=CARTESIAN_POINT('Ctrl Pts',(9.44632201614,-32.4742356128,4.7098382487));
#55433=CARTESIAN_POINT('Ctrl Pts',(8.51721509197,-35.3742356128,2.41066261776));
#55434=CARTESIAN_POINT('Ctrl Pts',(9.47312185748,-32.4742356128,4.57687569684));
#55435=CARTESIAN_POINT('Ctrl Pts',(9.47312185748,-32.4742356128,4.57687569684));
#55436=CARTESIAN_POINT('Ctrl Pts',(9.46576357172862,-32.4742356128,4.61338249695149));
#55437=CARTESIAN_POINT('Ctrl Pts',(9.45589852782759,-32.4742356128,4.64938312384879));
#55438=CARTESIAN_POINT('Ctrl Pts',(9.4436151767327,-32.4742356128001,4.68454468695718));
#55439=CARTESIAN_POINT('Ctrl Pts',(9.43116790267184,-32.4742356128001,4.72017548583586));
#55440=CARTESIAN_POINT('Ctrl Pts',(9.41623764589746,-32.4742356128001,4.75494407050594));
#55441=CARTESIAN_POINT('Ctrl Pts',(9.39896958249035,-32.4742356128001,4.78851518953424));
#55442=CARTESIAN_POINT('Ctrl Pts',(9.38152489595556,-32.4742356128002,4.82242968441788));
#55443=CARTESIAN_POINT('Ctrl Pts',(9.36169469208315,-32.4742356128002,4.85512144315062));
#55444=CARTESIAN_POINT('Ctrl Pts',(9.33967747672362,-32.4742356128002,4.88626565542905));
#55445=CARTESIAN_POINT('Ctrl Pts',(9.32473727646168,-32.4742356128002,4.90739915305088));
#55446=CARTESIAN_POINT('Ctrl Pts',(9.30879106644691,-32.4742356128002,4.92782051201125));
#55447=CARTESIAN_POINT('Ctrl Pts',(9.29191215925214,-32.4742356128002,4.94743594307661));
#55448=CARTESIAN_POINT('Ctrl Pts',(9.26807208685844,-32.4742356128001,4.97514113105093));
#55449=CARTESIAN_POINT('Ctrl Pts',(9.2423551960503,-32.4742356128002,5.00125358349318));
#55450=CARTESIAN_POINT('Ctrl Pts',(9.21499925935546,-32.4742356128004,5.02552229400269));
#55451=CARTESIAN_POINT('Ctrl Pts',(9.18812489694226,-32.4742356128005,5.04936377780233));
#55452=CARTESIAN_POINT('Ctrl Pts',(9.15966921110771,-32.4742356128007,5.07142540239296));
#55453=CARTESIAN_POINT('Ctrl Pts',(9.12988757458161,-32.4742356128009,5.09150932334396));
#55454=CARTESIAN_POINT('Ctrl Pts',(9.1177306388397,-32.474235612801,5.09970762823674));
#55455=CARTESIAN_POINT('Ctrl Pts',(9.10535306806464,-32.474235612801,5.1075768984626));
#55456=CARTESIAN_POINT('Ctrl Pts',(9.09277339742187,-32.4742356128011,5.11510591129192));
#55457=CARTESIAN_POINT('Ctrl Pts',(9.06401134948185,-32.4742356128012,5.13232017978011));
#55458=CARTESIAN_POINT('Ctrl Pts',(9.03418916029184,-32.4742356128013,5.1477537113724));
#55459=CARTESIAN_POINT('Ctrl Pts',(9.00352034950314,-32.4742356128012,5.1612883287322));
#55460=CARTESIAN_POINT('Ctrl Pts',(8.98613398992056,-32.4742356128012,5.16896119631913));
#55461=CARTESIAN_POINT('Ctrl Pts',(8.9684764199063,-32.4742356128011,5.17602435236192));
#55462=CARTESIAN_POINT('Ctrl Pts',(8.95059220546224,-32.474235612801,5.1824608849134));
#55463=CARTESIAN_POINT('Ctrl Pts',(8.91460611802292,-32.4742356128007,5.19541228537485));
#55464=CARTESIAN_POINT('Ctrl Pts',(8.8776867278997,-32.4742356128005,5.20582893332123));
#55465=CARTESIAN_POINT('Ctrl Pts',(8.84020622755982,-32.4742356128004,5.21361149973278));
#55466=CARTESIAN_POINT('Ctrl Pts',(8.80212100914067,-32.4742356128002,5.22151963166691));
#55467=CARTESIAN_POINT('Ctrl Pts',(8.76345811848754,-32.4742356128002,5.22670768415973));
#55468=CARTESIAN_POINT('Ctrl Pts',(8.72463030839696,-32.4742356128002,5.22912100680538));
#55469=CARTESIAN_POINT('Ctrl Pts',(8.68739236868495,-32.4742356128002,5.23143551187209));
#55470=CARTESIAN_POINT('Ctrl Pts',(8.65000425691521,-32.4742356128002,5.23119800092422));
#55471=CARTESIAN_POINT('Ctrl Pts',(8.6128267026259,-32.4742356128003,5.22840604118267));
#55472=CARTESIAN_POINT('Ctrl Pts',(8.58737790569537,-32.4742356128003,5.22649488758855));
#55473=CARTESIAN_POINT('Ctrl Pts',(8.56202769486349,-32.4742356128004,5.22338772754605));
#55474=CARTESIAN_POINT('Ctrl Pts',(8.53688547477249,-32.4742356128005,5.21909660544825));
#55475=CARTESIAN_POINT('Ctrl Pts',(8.50390469579943,-32.4742356128006,5.21346764551782));
#55476=CARTESIAN_POINT('Ctrl Pts',(8.47128746528097,-32.4742356128007,5.20580045842078));
#55477=CARTESIAN_POINT('Ctrl Pts',(8.4392653732531,-32.4742356128007,5.19615646079357));
#55478=CARTESIAN_POINT('Ctrl Pts',(8.43597511948344,-32.4742356128007,5.19516554491213));
#55479=CARTESIAN_POINT('Ctrl Pts',(8.43269111740371,-32.4742356128007,5.19415379222059));
#55480=CARTESIAN_POINT('Ctrl Pts',(8.42941359545578,-32.4742356128007,5.19312129233961));
#55481=CARTESIAN_POINT('Ctrl Pts',(8.3944144019285,-32.4742356128007,5.18209568710319));
#55482=CARTESIAN_POINT('Ctrl Pts',(8.36015521648491,-32.4742356128006,5.16869999519598));
#55483=CARTESIAN_POINT('Ctrl Pts',(8.32695087107122,-32.4742356128006,5.15305321371686));
#55484=CARTESIAN_POINT('Ctrl Pts',(8.29319095413242,-32.4742356128005,5.13714463197815));
#55485=CARTESIAN_POINT('Ctrl Pts',(8.26052202447813,-32.4742356128004,5.11890928463567));
#55486=CARTESIAN_POINT('Ctrl Pts',(8.22925624736326,-32.4742356128004,5.09852305936231));
#55487=CARTESIAN_POINT('Ctrl Pts',(8.20513847568554,-32.4742356128003,5.08279754821614));
#55488=CARTESIAN_POINT('Ctrl Pts',(8.18185530346072,-32.4742356128002,5.06579330067018));
#55489=CARTESIAN_POINT('Ctrl Pts',(8.15953944897647,-32.4742356128002,5.04760937719499));
#55490=CARTESIAN_POINT('Ctrl Pts',(8.13000306159537,-32.4742356128001,5.02354185120129));
#55491=CARTESIAN_POINT('Ctrl Pts',(8.1021534308539,-32.4742356128001,4.99739923287759));
#55492=CARTESIAN_POINT('Ctrl Pts',(8.07626720330521,-32.4742356128001,4.96943994770265));
#55493=CARTESIAN_POINT('Ctrl Pts',(8.0505351356036,-32.4742356128,4.94164716802253));
#55494=CARTESIAN_POINT('Ctrl Pts',(8.0267436078806,-32.4742356128,4.91205976688404));
#55495=CARTESIAN_POINT('Ctrl Pts',(8.00512575620472,-32.4742356128,4.88096523499291));
#55496=CARTESIAN_POINT('Ctrl Pts',(7.98386071885989,-32.4742356128,4.85037818167243));
#55497=CARTESIAN_POINT('Ctrl Pts',(7.96469932551459,-32.4742356128,4.81833327235114));
#55498=CARTESIAN_POINT('Ctrl Pts',(7.94782028391973,-32.4742356128,4.78512968374919));
#55499=CARTESIAN_POINT('Ctrl Pts',(7.94028653932774,-32.4742356128,4.77030968614097));
#55500=CARTESIAN_POINT('Ctrl Pts',(7.93320686704621,-32.4742356128,4.75525915977829));
#55501=CARTESIAN_POINT('Ctrl Pts',(7.92659403983,-32.4742356128,4.74000601033));
#55502=CARTESIAN_POINT('Origin',(-11.4022814987,-32.6742356128,-7.54785992694));
#55503=CARTESIAN_POINT('Origin',(-11.4022814987,-32.8742356128,-7.54785992694));
#55504=CARTESIAN_POINT('Ctrl Pts',(3.51985615629,-35.3742356128,-3.20601908088));
#55505=CARTESIAN_POINT('Ctrl Pts',(3.1350457731,-32.4742356128,-2.57376246377));
#55506=CARTESIAN_POINT('Ctrl Pts',(3.5389561844,-35.3742356128,-3.1668368061));
#55507=CARTESIAN_POINT('Ctrl Pts',(3.17276903042,-32.4742356128,-2.53334077836));
#55508=CARTESIAN_POINT('Ctrl Pts',(3.56517269185,-35.3742356128,-3.13112318899));
#55509=CARTESIAN_POINT('Ctrl Pts',(3.21038331308,-32.4742356128,-2.49281798697));
#55510=CARTESIAN_POINT('Ctrl Pts',(3.59940527056,-35.3742356128,-3.09917422736));
#55511=CARTESIAN_POINT('Ctrl Pts',(3.24932685202,-32.4742356128,-2.45063230102));
#55512=CARTESIAN_POINT('Ctrl Pts',(3.63699355357,-35.3742356128,-3.07546800882));
#55513=CARTESIAN_POINT('Ctrl Pts',(3.28665002885,-32.4742356128,-2.40998048911));
#55514=CARTESIAN_POINT('Ctrl Pts',(3.67755401867,-35.3742356128,-3.05915055738));
#55515=CARTESIAN_POINT('Ctrl Pts',(3.32386409198,-32.4742356128,-2.36922853848));
#55516=CARTESIAN_POINT('Origin',(-15.769898679409,-32.4742355606854,15.0680202722476));
#55517=CARTESIAN_POINT('Ctrl Pts',(-1.68475792039,-35.3742356128,-5.03973467448));
#55518=CARTESIAN_POINT('Ctrl Pts',(-0.682166339124,-32.4742356128,-4.8790713724));
#55519=CARTESIAN_POINT('Ctrl Pts',(-2.15538022242,-35.3742356128,-4.8080213959));
#55520=CARTESIAN_POINT('Ctrl Pts',(-1.20736921572,-32.4742356128,-4.44659694115));
#55521=CARTESIAN_POINT('Ctrl Pts',(-2.59973387128,-35.3742356128,-4.50528924317));
#55522=CARTESIAN_POINT('Ctrl Pts',(-1.71079094607,-32.4742356128,-4.00290111016));
#55523=CARTESIAN_POINT('Ctrl Pts',(-2.98121657961,-35.3742356128,-4.12686323533));
#55524=CARTESIAN_POINT('Ctrl Pts',(-2.19825830329,-32.4742356128,-3.54512092123));
#55525=CARTESIAN_POINT('Ctrl Pts',(-3.28679922947,-35.3742356128,-3.68411804659));
#55526=CARTESIAN_POINT('Ctrl Pts',(-2.67474264449,-32.4742356128,-3.06699209341));
#55527=CARTESIAN_POINT('Ctrl Pts',(-3.51985615629,-35.3742356128,-3.20601908088));
#55528=CARTESIAN_POINT('Ctrl Pts',(-3.1350457731,-32.4742356128,-2.57376246377));
#55529=CARTESIAN_POINT('',(-0.682166339124,-32.4742356128,-4.8790713724));
#55530=CARTESIAN_POINT('Ctrl Pts',(-3.1350457731,-32.4742356128,-2.57376246377));
#55531=CARTESIAN_POINT('Ctrl Pts',(-3.04574386842478,-32.4742356128,-2.66945233123215));
#55532=CARTESIAN_POINT('Ctrl Pts',(-2.95565520899676,-32.4742356128,-2.76451972688002));
#55533=CARTESIAN_POINT('Ctrl Pts',(-2.86486097840212,-32.4742356128,-2.85887905523607));
#55534=CARTESIAN_POINT('Ctrl Pts',(-2.76926551199805,-32.4742356128,-2.95822814321991));
#55535=CARTESIAN_POINT('Ctrl Pts',(-2.67288792014402,-32.4742356128,-3.05679239893703));
#55536=CARTESIAN_POINT('Ctrl Pts',(-2.57578459070286,-32.4742356128,-3.15451622941541));
#55537=CARTESIAN_POINT('Ctrl Pts',(-2.47439813201672,-32.4742356128001,
-3.25655055880935));
#55538=CARTESIAN_POINT('Ctrl Pts',(-2.37222039913981,-32.4742356128001,
-3.35766900818225));
#55539=CARTESIAN_POINT('Ctrl Pts',(-2.2692753175773,-32.4742356128001,-3.45785202544386));
#55540=CARTESIAN_POINT('Ctrl Pts',(-2.16032661276555,-32.4742356128001,
-3.56387758595748));
#55541=CARTESIAN_POINT('Ctrl Pts',(-2.05051830060976,-32.4742356128001,
-3.66885589509191));
#55542=CARTESIAN_POINT('Ctrl Pts',(-1.93983639318639,-32.4742356128001,
-3.77280566427766));
#55543=CARTESIAN_POINT('Ctrl Pts',(-1.81352928403153,-32.4742356128001,
-3.89143024483304));
#55544=CARTESIAN_POINT('Ctrl Pts',(-1.68608466211416,-32.4742356128001,
-4.00871596374921));
#55545=CARTESIAN_POINT('Ctrl Pts',(-1.55742711564637,-32.4742356128001,
-4.1247361422481));
#55546=CARTESIAN_POINT('Ctrl Pts',(-1.40954803390843,-32.4742356128001,
-4.25808982363347));
#55547=CARTESIAN_POINT('Ctrl Pts',(-1.26006594487636,-32.4742356128001,
-4.38977385603739));
#55548=CARTESIAN_POINT('Ctrl Pts',(-1.10880104134623,-32.4742356128001,
-4.51993332529904));
#55549=CARTESIAN_POINT('Ctrl Pts',(-0.968189500144993,-32.4742356128001,
-4.64092585659807));
#55550=CARTESIAN_POINT('Ctrl Pts',(-0.826035174351419,-32.4742356128001,
-4.760603642191));
#55551=CARTESIAN_POINT('Ctrl Pts',(-0.682166339124,-32.4742356128,-4.8790713724));
#55552=CARTESIAN_POINT('',(-1.65073607089,-35.2758272825,-5.03428274092));
#55553=CARTESIAN_POINT('Ctrl Pts',(-1.51727342606,-35.3742356128,-5.3088808072));
#55554=CARTESIAN_POINT('Ctrl Pts',(-0.5,-32.4742356128,-5.26505293156));
#55555=CARTESIAN_POINT('Ctrl Pts',(-1.51727346704,-35.3742356128,-5.24111839755));
#55556=CARTESIAN_POINT('Ctrl Pts',(-0.49999996933,-32.4742356128,-5.17707576222));
#55557=CARTESIAN_POINT('Ctrl Pts',(-1.53640667867,-35.3742356128,-5.1734830193));
#55558=CARTESIAN_POINT('Ctrl Pts',(-0.519349085752,-32.4742356128,-5.08894068096));
#55559=CARTESIAN_POINT('Ctrl Pts',(-1.57167084987,-35.3742356128,-5.11676901693));
#55560=CARTESIAN_POINT('Ctrl Pts',(-0.558553592228,-32.4742356128,-5.00590412413));
#55561=CARTESIAN_POINT('Ctrl Pts',(-1.62392373781,-35.3742356128,-5.06968674937));
#55562=CARTESIAN_POINT('Ctrl Pts',(-0.614278309582,-32.4742356128,-4.93497322721));
#55563=CARTESIAN_POINT('Ctrl Pts',(-1.68475792039,-35.3742356128,-5.03973467448));
#55564=CARTESIAN_POINT('Ctrl Pts',(-0.682166339124,-32.4742356128,-4.8790713724));
#55565=CARTESIAN_POINT('Ctrl Pts',(-0.5,-32.4742356128,-5.26505293156));
#55566=CARTESIAN_POINT('Ctrl Pts',(-0.499999987183553,-32.4742356128,-5.22828883820323));
#55567=CARTESIAN_POINT('Ctrl Pts',(-0.504054600653073,-32.4742356128085,
-5.19170069064497));
#55568=CARTESIAN_POINT('Ctrl Pts',(-0.520156709880915,-32.4742356128085,
-5.1199141043431));
#55569=CARTESIAN_POINT('Ctrl Pts',(-0.532168073174417,-32.4742356128085,
-5.08496970255448));
#55570=CARTESIAN_POINT('Ctrl Pts',(-0.56359844412932,-32.4742356128085,
-5.0183737839542));
#55571=CARTESIAN_POINT('Ctrl Pts',(-0.582941481982889,-32.4742356128085,
-4.98688524144264));
#55572=CARTESIAN_POINT('Ctrl Pts',(-0.628123824966223,-32.4742356128085,
-4.9288235651309));
#55573=CARTESIAN_POINT('Ctrl Pts',(-0.653788606277979,-32.4742356128,-4.90243878948513));
#55574=CARTESIAN_POINT('Ctrl Pts',(-0.682166339124,-32.4742356128,-4.8790713724));
#55575=CARTESIAN_POINT('Ctrl Pts',(-4.28541380927,-35.2854532781,6.68742874581));
#55576=CARTESIAN_POINT('Ctrl Pts',(-4.25138913038,-35.3190062343,6.67597344224));
#55577=CARTESIAN_POINT('Ctrl Pts',(-4.2237811371,-35.3599069399,6.66698101926));
#55578=CARTESIAN_POINT('Ctrl Pts',(-4.2045020858,-35.4062855354,6.66109563973));
#55579=CARTESIAN_POINT('Ctrl Pts',(-4.19468576835,-35.4554145177,6.65866342004));
#55580=CARTESIAN_POINT('Ctrl Pts',(-4.1943405118,-35.5045435,6.65962650016));
#55581=CARTESIAN_POINT('Ctrl Pts',(-4.11397205127,-35.2871903778,7.1289134397));
#55582=CARTESIAN_POINT('Ctrl Pts',(-4.08555020042,-35.3204422988,7.11511826715));
#55583=CARTESIAN_POINT('Ctrl Pts',(-4.06274263182,-35.3595779076,7.10432325981));
#55584=CARTESIAN_POINT('Ctrl Pts',(-4.04686969309,-35.4030115592,7.09721073519));
#55585=CARTESIAN_POINT('Ctrl Pts',(-4.03869401208,-35.448599951,7.09414682081));
#55586=CARTESIAN_POINT('Ctrl Pts',(-4.0382327119,-35.4941883428,7.09508332647));
#55587=CARTESIAN_POINT('Ctrl Pts',(-3.87798979897,-35.2903697142,7.5452931056));
#55588=CARTESIAN_POINT('Ctrl Pts',(-3.85569645887,-35.322762315,7.53067170905));
#55589=CARTESIAN_POINT('Ctrl Pts',(-3.8380083558,-35.3595811789,7.5193382333));
#55590=CARTESIAN_POINT('Ctrl Pts',(-3.82572295419,-35.3995642149,7.51187390423));
#55591=CARTESIAN_POINT('Ctrl Pts',(-3.81928961916,-35.4411316076,7.50858298657));
#55592=CARTESIAN_POINT('Ctrl Pts',(-3.81872923728,-35.4826990003,7.50943133393));
#55593=CARTESIAN_POINT('Ctrl Pts',(-3.58317382243,-35.2955286211,7.92387042867));
#55594=CARTESIAN_POINT('Ctrl Pts',(-3.566682617,-35.3261714515,7.91016667743));
#55595=CARTESIAN_POINT('Ctrl Pts',(-3.5536607286,-35.359954842,7.89965095547));
#55596=CARTESIAN_POINT('Ctrl Pts',(-3.54456703401,-35.395950925,7.89273240615));
#55597=CARTESIAN_POINT('Ctrl Pts',(-3.53965943927,-35.4330544417,7.88962174402));
#55598=CARTESIAN_POINT('Ctrl Pts',(-3.53895593719,-35.4701579585,7.89029829102));
#55599=CARTESIAN_POINT('Ctrl Pts',(-2.78825930398,-35.3119546911,8.68818242005));
#55600=CARTESIAN_POINT('Ctrl Pts',(-2.78273620813,-35.3367578784,8.67851811171));
#55601=CARTESIAN_POINT('Ctrl Pts',(-2.77847903433,-35.3625424695,8.67123634585));
#55602=CARTESIAN_POINT('Ctrl Pts',(-2.77550319185,-35.3889828306,8.66644973332));
#55603=CARTESIAN_POINT('Ctrl Pts',(-2.77381592126,-35.4157508538,8.66421370085));
#55604=CARTESIAN_POINT('Ctrl Pts',(-2.77342331871,-35.442518877,8.6645265191));
#55605=CARTESIAN_POINT('Ctrl Pts',(-1.7897157019,-35.3293337971,9.16292213266));
#55606=CARTESIAN_POINT('Ctrl Pts',(-1.78817752192,-35.3471147636,9.15782929567));
#55607=CARTESIAN_POINT('Ctrl Pts',(-1.78691123053,-35.3652255624,9.15399062253));
#55608=CARTESIAN_POINT('Ctrl Pts',(-1.78592585783,-35.383560442,9.15142772658));
#55609=CARTESIAN_POINT('Ctrl Pts',(-1.78522811689,-35.4020074661,9.15015177013));
#55610=CARTESIAN_POINT('Ctrl Pts',(-1.78481951479,-35.4204544903,9.15016319792));
#55611=CARTESIAN_POINT('Ctrl Pts',(-1.17958127456,-35.3376427744,9.32328709823));
#55612=CARTESIAN_POINT('Ctrl Pts',(-1.17951808488,-35.3526513961,9.31932369186));
#55613=CARTESIAN_POINT('Ctrl Pts',(-1.17962222045,-35.3679411233,9.31634876039));
#55614=CARTESIAN_POINT('Ctrl Pts',(-1.17989211248,-35.3834200246,9.31438871901));
#55615=CARTESIAN_POINT('Ctrl Pts',(-1.18032484655,-35.3989934955,9.31345658462));
#55616=CARTESIAN_POINT('Ctrl Pts',(-1.18091694182,-35.4145669664,9.31355164802));
#55617=CARTESIAN_POINT('Ctrl Pts',(-0.559260434794,-35.3376563848,9.36581532526));
#55618=CARTESIAN_POINT('Ctrl Pts',(-0.558548188498,-35.3519108871,9.36216300672));
#55619=CARTESIAN_POINT('Ctrl Pts',(-0.557879709548,-35.3663773783,9.35938680253));
#55620=CARTESIAN_POINT('Ctrl Pts',(-0.557259801436,-35.3809865088,9.35750427431));
#55621=CARTESIAN_POINT('Ctrl Pts',(-0.556692506327,-35.395666961,9.35652455583));
#55622=CARTESIAN_POINT('Ctrl Pts',(-0.556180950878,-35.4103474131,9.35644810405));
#55623=CARTESIAN_POINT('Ctrl Pts',(0.051310852811,-35.3354014219,9.29455995377));
#55624=CARTESIAN_POINT('Ctrl Pts',(0.0507151654701,-35.3508336959,9.290385971));
#55625=CARTESIAN_POINT('Ctrl Pts',(0.050239745093,-35.3665469388,9.28723363732));
#55626=CARTESIAN_POINT('Ctrl Pts',(0.0498881224817,-35.3824497265,9.28512769558));
#55627=CARTESIAN_POINT('Ctrl Pts',(0.0496623930249,-35.3984472911,9.28408069549));
#55628=CARTESIAN_POINT('Ctrl Pts',(0.0495631429636,-35.4144448557,9.28409255206));
#55629=CARTESIAN_POINT('',(-4.19434053880571,-35.5045435019704,6.65962642488774));
#55630=CARTESIAN_POINT('',(1.28564320474754E-7,-35.4141727791362,9.28969993583948));
#55631=CARTESIAN_POINT('Ctrl Pts',(-4.1943405118,-35.5045435,6.65962650016));
#55632=CARTESIAN_POINT('Ctrl Pts',(-4.17837930200538,-35.5034847390595,
6.70414969352822));
#55633=CARTESIAN_POINT('Ctrl Pts',(-4.16055959096817,-35.5023336268611,
6.75138464945794));
#55634=CARTESIAN_POINT('Ctrl Pts',(-4.14055681322333,-35.501089684398,6.80116841245276));
#55635=CARTESIAN_POINT('Ctrl Pts',(-4.12081028160109,-35.4998616774933,
6.85031441921199));
#55636=CARTESIAN_POINT('Ctrl Pts',(-4.09893583753898,-35.4985431603648,
6.9019447557283));
#55637=CARTESIAN_POINT('Ctrl Pts',(-4.07459349579852,-35.4971338643656,
6.95586055718833));
#55638=CARTESIAN_POINT('Ctrl Pts',(-4.05079014661857,-35.4957557732549,
7.00858254516111));
#55639=CARTESIAN_POINT('Ctrl Pts',(-4.02462648621315,-35.4942908306056,
7.06349021451113));
#55640=CARTESIAN_POINT('Ctrl Pts',(-3.99576468989804,-35.4927396443495,
7.12035197690877));
#55641=CARTESIAN_POINT('Ctrl Pts',(-3.98674519606888,-35.4922548888369,
7.13812163717041));
#55642=CARTESIAN_POINT('Ctrl Pts',(-3.97746208240242,-35.4917617201085,
7.15608177491406));
#55643=CARTESIAN_POINT('Ctrl Pts',(-3.96790474909657,-35.4912601864692,
7.17422430572546));
#55644=CARTESIAN_POINT('Ctrl Pts',(-3.93844658680729,-35.4897143306466,
7.23014425743976));
#55645=CARTESIAN_POINT('Ctrl Pts',(-3.90638395378748,-35.4880887908298,
7.28780020932287));
#55646=CARTESIAN_POINT('Ctrl Pts',(-3.8714013263532,-35.4863824392708,7.3469238129564));
#55647=CARTESIAN_POINT('Ctrl Pts',(-3.84516841075404,-35.4851028733916,
7.3912596624277));
#55648=CARTESIAN_POINT('Ctrl Pts',(-3.81729326251427,-35.4837779059508,
7.43641988355906));
#55649=CARTESIAN_POINT('Ctrl Pts',(-3.78764191907141,-35.4824082052946,
7.48227203951716));
#55650=CARTESIAN_POINT('Ctrl Pts',(-3.753045629466,-35.4808100800473,7.53577094656048));
#55651=CARTESIAN_POINT('Ctrl Pts',(-3.7160309687385,-35.4791503927134,7.5902128072203));
#55652=CARTESIAN_POINT('Ctrl Pts',(-3.6763871268798,-35.477419112457,7.64535684101877));
#55653=CARTESIAN_POINT('Ctrl Pts',(-3.65839989873091,-35.4766335949213,
7.67037682572456));
#55654=CARTESIAN_POINT('Ctrl Pts',(-3.64011367909671,-35.4758458242437,
7.69521128373181));
#55655=CARTESIAN_POINT('Ctrl Pts',(-3.62118640362598,-35.4750423837516,
7.72028918556664));
#55656=CARTESIAN_POINT('Ctrl Pts',(-3.60273483893631,-35.4742591366203,
7.7447367891693));
#55657=CARTESIAN_POINT('Ctrl Pts',(-3.58367398448364,-35.4734609836787,
7.76941596024569));
#55658=CARTESIAN_POINT('Ctrl Pts',(-3.56364805841191,-35.4726355159181,
7.79469365798657));
#55659=CARTESIAN_POINT('Ctrl Pts',(-3.55894115415355,-35.4724414975389,
7.80063494143642));
#55660=CARTESIAN_POINT('Ctrl Pts',(-3.55418076305494,-35.4722459707925,
7.80660914540214));
#55661=CARTESIAN_POINT('Ctrl Pts',(-3.54936194187392,-35.4720487760647,
7.812620756905));
#55662=CARTESIAN_POINT('Ctrl Pts',(-3.50132504757105,-35.4700830209682,
7.87254809919573));
#55663=CARTESIAN_POINT('Ctrl Pts',(-3.45312102456255,-35.4681824662924,
7.92915836150545));
#55664=CARTESIAN_POINT('Ctrl Pts',(-3.40514157153254,-35.4663543570109,
7.98262940663339));
#55665=CARTESIAN_POINT('Ctrl Pts',(-3.3545301321423,-35.4644259639957,8.03903368781461));
#55666=CARTESIAN_POINT('Ctrl Pts',(-3.30416891042736,-35.4625781811888,
8.09194534533543));
#55667=CARTESIAN_POINT('Ctrl Pts',(-3.2544613417438,-35.4608154968839,8.14159549761834));
#55668=CARTESIAN_POINT('Ctrl Pts',(-3.20479882986081,-35.4590544103421,
8.19120064514505));
#55669=CARTESIAN_POINT('Ctrl Pts',(-3.15578853664244,-35.4573782131692,
8.23755081827941));
#55670=CARTESIAN_POINT('Ctrl Pts',(-3.10777820415445,-35.4557879751255,
8.28088966193874));
#55671=CARTESIAN_POINT('Ctrl Pts',(-3.05787405529245,-35.4541350085255,
8.32593805034603));
#55672=CARTESIAN_POINT('Ctrl Pts',(-3.0090492646001,-35.4525748349097,8.36773430141987));
#55673=CARTESIAN_POINT('Ctrl Pts',(-2.96164060662634,-35.4511058720778,
8.40655378230749));
#55674=CARTESIAN_POINT('Ctrl Pts',(-2.91770603913525,-35.4497445543473,
8.44252858471531));
#55675=CARTESIAN_POINT('Ctrl Pts',(-2.87498738991999,-35.4484615152779,
8.47594687353619));
#55676=CARTESIAN_POINT('Ctrl Pts',(-2.83371152617201,-35.4472539635573,
8.50702594740405));
#55677=CARTESIAN_POINT('Ctrl Pts',(-2.7881274088724,-35.4459203711313,8.54134896381397));
#55678=CARTESIAN_POINT('Ctrl Pts',(-2.74430435080188,-35.4446791995284,
8.57281938357731));
#55679=CARTESIAN_POINT('Ctrl Pts',(-2.70250195888283,-35.4435296775847,
8.60172084488821));
#55680=CARTESIAN_POINT('Ctrl Pts',(-2.66331221645872,-35.4424520007626,
8.62881596486717));
#55681=CARTESIAN_POINT('Ctrl Pts',(-2.62589740734801,-35.4414547032728,
8.65365341888502));
#55682=CARTESIAN_POINT('Ctrl Pts',(-2.59043271192644,-35.4405342286928,
8.67645002768075));
#55683=CARTESIAN_POINT('Ctrl Pts',(-2.58212067393701,-35.4403184924631,
8.68179298286726));
#55684=CARTESIAN_POINT('Ctrl Pts',(-2.57391560780485,-35.4401069682295,
8.68702375355189));
#55685=CARTESIAN_POINT('Ctrl Pts',(-2.56581950543256,-35.4398995977304,
8.69214497970277));
#55686=CARTESIAN_POINT('Ctrl Pts',(-2.56543203379652,-35.4398896731787,
8.69239007663757));
#55687=CARTESIAN_POINT('Ctrl Pts',(-2.56504481172373,-35.4398797581405,
8.69263492264965));
#55688=CARTESIAN_POINT('Ctrl Pts',(-2.56465783942697,-35.4398698526091,
8.69287951802502));
#55689=CARTESIAN_POINT('Ctrl Pts',(-2.56441498501931,-35.4398636361384,
8.69303302013744));
#55690=CARTESIAN_POINT('Ctrl Pts',(-2.56417222898623,-35.439857423412,8.69318642353627));
#55691=CARTESIAN_POINT('Ctrl Pts',(-2.56392957138023,-35.4398512144283,
8.69333972829214));
#55692=CARTESIAN_POINT('Ctrl Pts',(-2.56376214454781,-35.4398469304065,
8.69344550420451));
#55693=CARTESIAN_POINT('Ctrl Pts',(-2.56359473338293,-35.4398426473919,
8.69355125215866));
#55694=CARTESIAN_POINT('Ctrl Pts',(-2.56343784477848,-35.4398386340855,
8.69365033845224));
#55695=CARTESIAN_POINT('Ctrl Pts',(-2.56250776449831,-35.4398148420632,
8.69423775018949));
#55696=CARTESIAN_POINT('Ctrl Pts',(-2.56183838046285,-35.439797731233,8.69466014382177));
#55697=CARTESIAN_POINT('Ctrl Pts',(-2.56096334291628,-35.4397753772487,
8.69521189922955));
#55698=CARTESIAN_POINT('Ctrl Pts',(-2.56052667867185,-35.4397642220867,
8.6954872381098));
#55699=CARTESIAN_POINT('Ctrl Pts',(-2.56003879045694,-35.4397517617935,
8.69579477361531));
#55700=CARTESIAN_POINT('Ctrl Pts',(-2.55944163055637,-35.4397365191539,
8.69617093880344));
#55701=CARTESIAN_POINT('Ctrl Pts',(-2.55918938502879,-35.4397300805305,
8.69632983424542));
#55702=CARTESIAN_POINT('Ctrl Pts',(-2.55891764121507,-35.4397231455062,
8.69650097358499));
#55703=CARTESIAN_POINT('Ctrl Pts',(-2.55862201831283,-35.439715603024,8.69668709372278));
#55704=CARTESIAN_POINT('Ctrl Pts',(-2.55841357168626,-35.4397102847453,
8.69681832886919));
#55705=CARTESIAN_POINT('Ctrl Pts',(-2.55819325278148,-35.4397046644545,
8.6969570120502));
#55706=CARTESIAN_POINT('Ctrl Pts',(-2.55795952442937,-35.4396987032875,
8.69710410051035));
#55707=CARTESIAN_POINT('Ctrl Pts',(-2.55777101635765,-35.4396938954494,
8.69722273122736));
#55708=CARTESIAN_POINT('Ctrl Pts',(-2.55757624887405,-35.4396889287289,
8.69734527846241));
#55709=CARTESIAN_POINT('Ctrl Pts',(-2.55738401031714,-35.4396840272794,
8.69746621131631));
#55710=CARTESIAN_POINT('Ctrl Pts',(-2.46893434127246,-35.4374288522792,
8.75310786341616));
#55711=CARTESIAN_POINT('Ctrl Pts',(-2.37904006043683,-35.4353007995903,
8.80483067803399));
#55712=CARTESIAN_POINT('Ctrl Pts',(-2.28808612479403,-35.4333174785345,
8.85264623177789));
#55713=CARTESIAN_POINT('Ctrl Pts',(-2.19146999759537,-35.4312106890036,
8.90343846621994));
#55714=CARTESIAN_POINT('Ctrl Pts',(-2.09365805541918,-35.4292668399415,
8.9498217080444));
#55715=CARTESIAN_POINT('Ctrl Pts',(-1.99507393204673,-35.4274916884687,
8.99185359254555));
#55716=CARTESIAN_POINT('Ctrl Pts',(-1.89277409786276,-35.4256496301829,
9.03546969083616));
#55717=CARTESIAN_POINT('Ctrl Pts',(-1.78964251137895,-35.4239887620901,
9.07440034576536));
#55718=CARTESIAN_POINT('Ctrl Pts',(-1.68611634000585,-35.4225062084511,
9.10875546973269));
#55719=CARTESIAN_POINT('Ctrl Pts',(-1.5875040832196,-35.4210940248629,9.14147991285326));
#55720=CARTESIAN_POINT('Ctrl Pts',(-1.48853326431828,-35.4198432538259,
9.17005348776741));
#55721=CARTESIAN_POINT('Ctrl Pts',(-1.38955619837585,-35.4187494160414,
9.1946054037486));
#55722=CARTESIAN_POINT('Ctrl Pts',(-1.31611675982145,-35.4179378054729,
9.21282254231424));
#55723=CARTESIAN_POINT('Ctrl Pts',(-1.24267047477725,-35.4172125277507,
9.22882666254555));
#55724=CARTESIAN_POINT('Ctrl Pts',(-1.16937199814094,-35.4165726765175,
9.24267804009084));
#55725=CARTESIAN_POINT('Ctrl Pts',(-1.04699987075702,-35.4155044420848,
9.2658029754947));
#55726=CARTESIAN_POINT('Ctrl Pts',(-0.925027460321667,-35.4146731250409,
9.28293054387911));
#55727=CARTESIAN_POINT('Ctrl Pts',(-0.803994903273425,-35.414083580067,
9.29440967641859));
#55728=CARTESIAN_POINT('Ctrl Pts',(-0.677910364703607,-35.4134694270836,
9.30636795578342));
#55729=CARTESIAN_POINT('Ctrl Pts',(-0.552845273492524,-35.4131170907703,
9.31219700428478));
#55730=CARTESIAN_POINT('Ctrl Pts',(-0.429367066302641,-35.4130544209605,
9.31232207470645));
#55731=CARTESIAN_POINT('Ctrl Pts',(-0.299788995201549,-35.4129886552416,
9.31245332364794));
#55732=CARTESIAN_POINT('Ctrl Pts',(-0.171958012842119,-35.4132413396774,
9.30630375762155));
#55733=CARTESIAN_POINT('Ctrl Pts',(-0.0464907907025172,-35.4138776107364,
9.29438835716944));
#55734=CARTESIAN_POINT('Ctrl Pts',(-0.030957288939788,-35.4139563844387,
9.29291316794655));
#55735=CARTESIAN_POINT('Ctrl Pts',(-0.0154599763576345,-35.4140410829517,
9.29134962256341));
#55736=CARTESIAN_POINT('Ctrl Pts',(1.08019642119928E-8,-35.4141318686722,
9.28969871436959));
#55737=CARTESIAN_POINT('',(-4.28541381254212,-35.2854532749087,6.68742874666406));
#55738=CARTESIAN_POINT('Origin',(-4.4767627864762,-35.5045528948602,6.76087185974608));
#55739=CARTESIAN_POINT('',(6.71017130748908E-10,-35.3356164375956,9.30022551106375));
#55740=CARTESIAN_POINT('Ctrl Pts',(-4.28541380927,-35.2854532781,6.68742874581));
#55741=CARTESIAN_POINT('Ctrl Pts',(-4.24121616134092,-35.2859025484266,
6.80123908869553));
#55742=CARTESIAN_POINT('Ctrl Pts',(-4.19186847493088,-35.2864674277753,
6.91304437631602));
#55743=CARTESIAN_POINT('Ctrl Pts',(-4.13760176200921,-35.2871642627959,
7.02239230617209));
#55744=CARTESIAN_POINT('Ctrl Pts',(-4.08296289616635,-35.2878658766059,
7.13249012761604));
#55745=CARTESIAN_POINT('Ctrl Pts',(-4.0233374286172,-35.2887014167807,7.24009677953585));
#55746=CARTESIAN_POINT('Ctrl Pts',(-3.95899998176384,-35.2896788346738,
7.34478595162515));
#55747=CARTESIAN_POINT('Ctrl Pts',(-3.89400268928686,-35.2906662769765,
7.4505488171142));
#55748=CARTESIAN_POINT('Ctrl Pts',(-3.82419638177896,-35.2917986928545,
7.55333404201523));
#55749=CARTESIAN_POINT('Ctrl Pts',(-3.74990195024538,-35.293072923249,7.65273807851349));
#55750=CARTESIAN_POINT('Ctrl Pts',(-3.70090134743733,-35.2939133369403,
7.71829962342909));
#55751=CARTESIAN_POINT('Ctrl Pts',(-3.64994917793588,-35.2948152022339,
7.78239108781155));
#55752=CARTESIAN_POINT('Ctrl Pts',(-3.59714596398303,-35.2957744035521,
7.844905146357));
#55753=CARTESIAN_POINT('Ctrl Pts',(-3.51612022470366,-35.2972462835781,
7.94083203091221));
#55754=CARTESIAN_POINT('Ctrl Pts',(-3.43073437116214,-35.2988540402996,
8.03304296381226));
#55755=CARTESIAN_POINT('Ctrl Pts',(-3.34138037370368,-35.3005693892819,
8.12118035250671));
#55756=CARTESIAN_POINT('Ctrl Pts',(-3.25130839572758,-35.3022985214993,
8.21002594597945));
#55757=CARTESIAN_POINT('Ctrl Pts',(-3.15720439860138,-35.3041371751793,
8.29473227506716));
#55758=CARTESIAN_POINT('Ctrl Pts',(-3.05950307372847,-35.306037411305,8.37496990585234));
#55759=CARTESIAN_POINT('Ctrl Pts',(-2.99330872457544,-35.3073248543745,
8.42933229811585));
#55760=CARTESIAN_POINT('Ctrl Pts',(-2.92546378256917,-35.3086401700654,
8.48164418952771));
#55761=CARTESIAN_POINT('Ctrl Pts',(-2.85611143541241,-35.3099628824964,
8.53181257836513));
#55762=CARTESIAN_POINT('Ctrl Pts',(-2.7579102438772,-35.3118358102646,8.60284976402952));
#55763=CARTESIAN_POINT('Ctrl Pts',(-2.65668403889593,-35.3137240757601,
8.6695883304476));
#55764=CARTESIAN_POINT('Ctrl Pts',(-2.55280108748868,-35.3155893473178,
8.73178544516782));
#55765=CARTESIAN_POINT('Ctrl Pts',(-2.44221408927618,-35.3175749934669,
8.79799642705862));
#55766=CARTESIAN_POINT('Ctrl Pts',(-2.32861692417884,-35.3195340519872,
8.85906027617959));
#55767=CARTESIAN_POINT('Ctrl Pts',(-2.2124999638606,-35.3214069653231,8.9147190921565));
#55768=CARTESIAN_POINT('Ctrl Pts',(-2.09381254498969,-35.3233213389771,
8.97161001651075));
#55769=CARTESIAN_POINT('Ctrl Pts',(-1.97249361548399,-35.325144935522,9.02285350430027));
#55770=CARTESIAN_POINT('Ctrl Pts',(-1.84910037198909,-35.3268109971623,
9.06821758004431));
#55771=CARTESIAN_POINT('Ctrl Pts',(-1.72708337710787,-35.3284584766262,
9.11307569416042));
#55772=CARTESIAN_POINT('Ctrl Pts',(-1.60303930200272,-35.3299511497321,
9.15218460722));
#55773=CARTESIAN_POINT('Ctrl Pts',(-1.47752178591338,-35.3312330133406,
9.18536663014834));
#55774=CARTESIAN_POINT('Ctrl Pts',(-1.42949741113993,-35.3317234683803,
9.19806243512044));
#55775=CARTESIAN_POINT('Ctrl Pts',(-1.38125739859416,-35.3321832123494,
9.20989110168217));
#55776=CARTESIAN_POINT('Ctrl Pts',(-1.3328327737408,-35.3326098028966,9.22084461008599));
#55777=CARTESIAN_POINT('Ctrl Pts',(-1.2154203786744,-35.3336441323935,9.24740295018603));
#55778=CARTESIAN_POINT('Ctrl Pts',(-1.09692351296306,-35.3344820309447,
9.26881355340909));
#55779=CARTESIAN_POINT('Ctrl Pts',(-0.977777965211198,-35.3351024675867,
9.28498986052386));
#55780=CARTESIAN_POINT('Ctrl Pts',(-0.862993660581534,-35.3357001935602,
9.30057404473115));
#55781=CARTESIAN_POINT('Ctrl Pts',(-0.747607895410976,-35.3360957669442,
9.31130017226629));
#55782=CARTESIAN_POINT('Ctrl Pts',(-0.631993617559925,-35.336293183438,
9.31712752395354));
#55783=CARTESIAN_POINT('Ctrl Pts',(-0.522375721082263,-35.3364803608454,
9.322652637684));
#55784=CARTESIAN_POINT('Ctrl Pts',(-0.412552756634451,-35.3364892580904,
9.32377410534818));
#55785=CARTESIAN_POINT('Ctrl Pts',(-0.302820690862792,-35.3363472934361,
9.32048915886595));
#55786=CARTESIAN_POINT('Ctrl Pts',(-0.201733708311387,-35.3362165132632,
9.31746301217496));
#55787=CARTESIAN_POINT('Ctrl Pts',(-0.100723941336883,-35.3359577568238,
9.31069766500961));
#55788=CARTESIAN_POINT('Ctrl Pts',(-1.0275302666507E-6,-35.335613767487,
9.30021571851796));
#55789=CARTESIAN_POINT('Ctrl Pts',(-5.55111512312578E-16,-35.3356137401038,
9.30021561809536));
#55790=CARTESIAN_POINT('Ctrl Pts',(-3.26505811906785E-15,-35.3545578006911,
9.29505018686761));
#55791=CARTESIAN_POINT('Ctrl Pts',(8.15014156923914E-10,-35.3739634390451,
9.29176495584985));
#55792=CARTESIAN_POINT('Ctrl Pts',(7.95444545790306E-10,-35.4004018758749,
9.28993613405734));
#55793=CARTESIAN_POINT('Ctrl Pts',(-3.35855341939055E-14,-35.4072658059936,
9.28969890048895));
#55794=CARTESIAN_POINT('Ctrl Pts',(-5.77315972805081E-14,-35.4141318686725,
9.28969871552309));
#55795=CARTESIAN_POINT('Ctrl Pts',(-4.4921212186,-35.2852060642,5.83250225932));
#55796=CARTESIAN_POINT('Ctrl Pts',(-4.45609896257,-35.3187908592,5.82727337616));
#55797=CARTESIAN_POINT('Ctrl Pts',(-4.42697003004,-35.3598847848,5.82278643887));
#55798=CARTESIAN_POINT('Ctrl Pts',(-4.40679129181,-35.4065868334,5.81933970701));
#55799=CARTESIAN_POINT('Ctrl Pts',(-4.39676908915,-35.4561050262,5.81713923581));
#55800=CARTESIAN_POINT('Ctrl Pts',(-4.39688470965,-35.505623219,5.81623490373));
#55801=CARTESIAN_POINT('Ctrl Pts',(-4.47934426829,-35.2848180141,5.95513865982));
#55802=CARTESIAN_POINT('Ctrl Pts',(-4.44240767125,-35.3184648135,5.94886804446));
#55803=CARTESIAN_POINT('Ctrl Pts',(-4.41246275486,-35.3599636587,5.94360014588));
#55804=CARTESIAN_POINT('Ctrl Pts',(-4.39168683777,-35.4073477788,5.9397026792));
#55805=CARTESIAN_POINT('Ctrl Pts',(-4.38136362076,-35.457688004,5.93741576176));
#55806=CARTESIAN_POINT('Ctrl Pts',(-4.38147338286,-35.5080282291,5.93677544119));
#55807=CARTESIAN_POINT('Ctrl Pts',(-4.46080331489,-35.2846612104,6.0774500678));
#55808=CARTESIAN_POINT('Ctrl Pts',(-4.42339099946,-35.3183175745,6.07010629864));
#55809=CARTESIAN_POINT('Ctrl Pts',(-4.39300176947,-35.3600459293,6.06403311375));
#55810=CARTESIAN_POINT('Ctrl Pts',(-4.37188741448,-35.4078395887,6.05967077608));
#55811=CARTESIAN_POINT('Ctrl Pts',(-4.36138132105,-35.4586803826,6.05729403028));
#55812=CARTESIAN_POINT('Ctrl Pts',(-4.36146441688,-35.5095211765,6.05692288884));
#55813=CARTESIAN_POINT('Ctrl Pts',(-4.43653605144,-35.2846213402,6.19885974208));
#55814=CARTESIAN_POINT('Ctrl Pts',(-4.39907245731,-35.3182793407,6.19048378347));
#55815=CARTESIAN_POINT('Ctrl Pts',(-4.36860698734,-35.360098105,6.18364473746));
#55816=CARTESIAN_POINT('Ctrl Pts',(-4.34741298485,-35.4080551513,6.17885069748));
#55817=CARTESIAN_POINT('Ctrl Pts',(-4.33684033846,-35.4590962326,6.17640727689));
#55818=CARTESIAN_POINT('Ctrl Pts',(-4.33687279452,-35.5101373139,6.17631673235));
#55819=CARTESIAN_POINT('Ctrl Pts',(-4.39382617826,-35.2846522393,6.3704629655));
#55820=CARTESIAN_POINT('Ctrl Pts',(-4.35687304692,-35.3183144911,6.36073630622));
#55821=CARTESIAN_POINT('Ctrl Pts',(-4.32681014412,-35.360077369,6.35290824863));
#55822=CARTESIAN_POINT('Ctrl Pts',(-4.3058660926,-35.4079286751,6.34756704555));
#55823=CARTESIAN_POINT('Ctrl Pts',(-4.295366459,-35.4588388005,6.34505127094));
#55824=CARTESIAN_POINT('Ctrl Pts',(-4.29530142772,-35.5097489259,6.34533949948));
#55825=CARTESIAN_POINT('Ctrl Pts',(-4.33989513123,-35.2849598896,6.53848806555));
#55826=CARTESIAN_POINT('Ctrl Pts',(-4.30425869633,-35.3185874247,6.5277361976));
#55827=CARTESIAN_POINT('Ctrl Pts',(-4.27529524943,-35.3599922268,6.51919887852));
#55828=CARTESIAN_POINT('Ctrl Pts',(-4.25509182459,-35.4072223024,6.51350637116));
#55829=CARTESIAN_POINT('Ctrl Pts',(-4.2448885603,-35.4573782014,6.51100829607));
#55830=CARTESIAN_POINT('Ctrl Pts',(-4.2446848137,-35.5075341005,6.51166242388));
#55831=CARTESIAN_POINT('Ctrl Pts',(-4.32271334112,-35.2850814359,6.58854936739));
#55832=CARTESIAN_POINT('Ctrl Pts',(-4.28754475087,-35.3186934865,6.57751968609));
#55833=CARTESIAN_POINT('Ctrl Pts',(-4.25897443759,-35.3599624877,6.56879320674));
#55834=CARTESIAN_POINT('Ctrl Pts',(-4.23903851349,-35.4069590258,6.56300941547));
#55835=CARTESIAN_POINT('Ctrl Pts',(-4.22894623833,-35.4568320218,6.56051917828));
#55836=CARTESIAN_POINT('Ctrl Pts',(-4.22869977692,-35.5067050179,6.56127483435));
#55837=CARTESIAN_POINT('Ctrl Pts',(-4.30455023491,-35.2852434072,6.6381975116));
#55838=CARTESIAN_POINT('Ctrl Pts',(-4.26991817238,-35.3188318732,6.62693608199));
#55839=CARTESIAN_POINT('Ctrl Pts',(-4.24179867527,-35.3599337083,6.61806209525));
#55840=CARTESIAN_POINT('Ctrl Pts',(-4.22216945818,-35.4066468932,6.61221922778));
#55841=CARTESIAN_POINT('Ctrl Pts',(-4.21220416739,-35.4561778332,6.6097570786));
#55842=CARTESIAN_POINT('Ctrl Pts',(-4.21190811788,-35.5057087732,6.61062231004));
#55843=CARTESIAN_POINT('Ctrl Pts',(-4.28541381497,-35.285453273,6.6874287475));
#55844=CARTESIAN_POINT('Ctrl Pts',(-4.251389142,-35.3190062299,6.67597342108));
#55845=CARTESIAN_POINT('Ctrl Pts',(-4.22378115684,-35.359906937,6.66698096996));
#55846=CARTESIAN_POINT('Ctrl Pts',(-4.20450211564,-35.4062855347,6.66109555831));
#55847=CARTESIAN_POINT('Ctrl Pts',(-4.19468580977,-35.4554145194,6.65866330444));
#55848=CARTESIAN_POINT('Ctrl Pts',(-4.1943405656,-35.5045435041,6.65962635024));
#55849=CARTESIAN_POINT('',(-4.39688473843144,-35.505623218299,5.81623468041465));
#55850=CARTESIAN_POINT('',(-4.49212120371157,-35.2852060781985,5.83250225674026));
#55851=CARTESIAN_POINT('Origin',(-4.69448488168448,-35.505632917967,5.85428086421669));
#55852=CARTESIAN_POINT('Ctrl Pts',(-4.49212120371,-35.2852060782,5.83250225674));
#55853=CARTESIAN_POINT('Ctrl Pts',(-4.47934426829,-35.2848180141,5.95513865982));
#55854=CARTESIAN_POINT('Ctrl Pts',(-4.46080331489,-35.2846612104,6.0774500678));
#55855=CARTESIAN_POINT('Ctrl Pts',(-4.43653605144,-35.2846213402,6.19885974208));
#55856=CARTESIAN_POINT('Ctrl Pts',(-4.39382617826,-35.2846522393,6.3704629655));
#55857=CARTESIAN_POINT('Ctrl Pts',(-4.33989513123,-35.2849598896,6.53848806555));
#55858=CARTESIAN_POINT('Ctrl Pts',(-4.32271334112,-35.2850814359,6.58854936739));
#55859=CARTESIAN_POINT('Ctrl Pts',(-4.30455023491,-35.2852434072,6.6381975116));
#55860=CARTESIAN_POINT('Ctrl Pts',(-4.2854138145,-35.285453273,6.68742874721));
#55861=CARTESIAN_POINT('Ctrl Pts',(-4.39688470965,-35.505623219,5.81623490373));
#55862=CARTESIAN_POINT('Ctrl Pts',(-4.38545059998313,-35.507407563559,5.90566741939867));
#55863=CARTESIAN_POINT('Ctrl Pts',(-4.37100172655426,-35.5085885511775,
5.99465197633656));
#55864=CARTESIAN_POINT('Ctrl Pts',(-4.35358930347287,-35.5091884954551,
6.08296676348967));
#55865=CARTESIAN_POINT('Ctrl Pts',(-4.33595593723731,-35.5097960523195,
6.17240216134366));
#55866=CARTESIAN_POINT('Ctrl Pts',(-4.31528465861745,-35.5098065202248,
6.26115007221233));
#55867=CARTESIAN_POINT('Ctrl Pts',(-4.29163457916425,-35.5092195580943,
6.34902509595134));
#55868=CARTESIAN_POINT('Ctrl Pts',(-4.28600488465352,-35.5090798368941,
6.36994297657631));
#55869=CARTESIAN_POINT('Ctrl Pts',(-4.28020637624591,-35.5089062055461,
6.39081161831919));
#55870=CARTESIAN_POINT('Ctrl Pts',(-4.2742397731198,-35.5086985824798,6.41162895166904));
#55871=CARTESIAN_POINT('Ctrl Pts',(-4.26005358598373,-35.5082049381717,
6.46112421393691));
#55872=CARTESIAN_POINT('Ctrl Pts',(-4.24491858163952,-35.5075194868754,
6.51032521145546));
#55873=CARTESIAN_POINT('Ctrl Pts',(-4.22884677793683,-35.506639317091,6.55919989334204));
#55874=CARTESIAN_POINT('Ctrl Pts',(-4.21778592957061,-35.5060335714819,
6.59283615815062));
#55875=CARTESIAN_POINT('Ctrl Pts',(-4.20628031810575,-35.5053354769618,
6.62632085027922));
#55876=CARTESIAN_POINT('Ctrl Pts',(-4.1943405656018,-35.5045435041,6.65962635023498));
#55877=CARTESIAN_POINT('Ctrl Pts',(-3.30528115437,-35.2990850504,2.45651113175));
#55878=CARTESIAN_POINT('Ctrl Pts',(-3.29174997169,-35.3282258256,2.47004153063));
#55879=CARTESIAN_POINT('Ctrl Pts',(-3.28123332764,-35.3601461205,2.48060031812));
#55880=CARTESIAN_POINT('Ctrl Pts',(-3.27411296889,-35.3940266351,2.48780578271));
#55881=CARTESIAN_POINT('Ctrl Pts',(-3.27059465556,-35.4288883092,2.49144970493));
#55882=CARTESIAN_POINT('Ctrl Pts',(-3.2706750272,-35.4637499833,2.49153088745));
#55883=CARTESIAN_POINT('Ctrl Pts',(-3.52263014734,-35.2997786652,2.67764867799));
#55884=CARTESIAN_POINT('Ctrl Pts',(-3.50832158865,-35.3287004593,2.68978061947));
#55885=CARTESIAN_POINT('Ctrl Pts',(-3.49718986878,-35.3603042564,2.69922432977));
#55886=CARTESIAN_POINT('Ctrl Pts',(-3.48962934617,-35.3937968185,2.70564685787));
#55887=CARTESIAN_POINT('Ctrl Pts',(-3.48585336684,-35.4282347239,2.70886780417));
#55888=CARTESIAN_POINT('Ctrl Pts',(-3.48586067783,-35.4626726292,2.70888759263));
#55889=CARTESIAN_POINT('Ctrl Pts',(-3.71975032728,-35.2998840308,2.91888544948));
#55890=CARTESIAN_POINT('Ctrl Pts',(-3.70452693031,-35.3287908762,2.92986690945));
#55891=CARTESIAN_POINT('Ctrl Pts',(-3.69266813705,-35.3603788898,2.93839702263));
#55892=CARTESIAN_POINT('Ctrl Pts',(-3.68459264153,-35.3938552567,2.94417305658));
#55893=CARTESIAN_POINT('Ctrl Pts',(-3.68052780808,-35.4282767651,2.94703197385));
#55894=CARTESIAN_POINT('Ctrl Pts',(-3.68047391974,-35.4626982735,2.94697615221));
#55895=CARTESIAN_POINT('Ctrl Pts',(-3.89420210101,-35.2992579912,3.17776652664));
#55896=CARTESIAN_POINT('Ctrl Pts',(-3.87780196962,-35.3284044612,3.18777591948));
#55897=CARTESIAN_POINT('Ctrl Pts',(-3.86500520386,-35.3603251829,3.19553496378));
#55898=CARTESIAN_POINT('Ctrl Pts',(-3.85627187964,-35.3942021449,3.20076023088));
#55899=CARTESIAN_POINT('Ctrl Pts',(-3.85185292871,-35.4290582738,3.20330006316));
#55900=CARTESIAN_POINT('Ctrl Pts',(-3.85174986217,-35.4639144026,3.20315896516));
#55901=CARTESIAN_POINT('Ctrl Pts',(-4.25043308745,-35.2963608901,3.82861914207));
#55902=CARTESIAN_POINT('Ctrl Pts',(-4.23039390269,-35.3265730217,3.83636634601));
#55903=CARTESIAN_POINT('Ctrl Pts',(-4.21468510082,-35.3600305104,3.84233146345));
#55904=CARTESIAN_POINT('Ctrl Pts',(-4.20392503792,-35.3957885434,3.84626231873));
#55905=CARTESIAN_POINT('Ctrl Pts',(-4.19845399885,-35.4326982838,3.848026993));
#55906=CARTESIAN_POINT('Ctrl Pts',(-4.19827560656,-35.4696080243,3.84763795769));
#55907=CARTESIAN_POINT('Ctrl Pts',(-4.45858902825,-35.291449905,4.54475674437));
#55908=CARTESIAN_POINT('Ctrl Pts',(-4.43308531823,-35.3233621358,4.54953750297));
#55909=CARTESIAN_POINT('Ctrl Pts',(-4.41292476175,-35.3596262841,4.55315251935));
#55910=CARTESIAN_POINT('Ctrl Pts',(-4.39907396454,-35.3990181868,4.55540464772));
#55911=CARTESIAN_POINT('Ctrl Pts',(-4.39207409827,-35.4399769064,4.55619669281));
#55912=CARTESIAN_POINT('Ctrl Pts',(-4.39192731775,-35.480935626,4.55555318454));
#55913=CARTESIAN_POINT('Ctrl Pts',(-4.52558545037,-35.2885903077,4.9733945174));
#55914=CARTESIAN_POINT('Ctrl Pts',(-4.4963387214,-35.3214318737,4.97577624036));
#55915=CARTESIAN_POINT('Ctrl Pts',(-4.4730869275,-35.3595080502,4.97747837329));
#55916=CARTESIAN_POINT('Ctrl Pts',(-4.45708682842,-35.4013807813,4.97836774601));
#55917=CARTESIAN_POINT('Ctrl Pts',(-4.44904844444,-35.4451561726,4.97838721155));
#55918=CARTESIAN_POINT('Ctrl Pts',(-4.44897072855,-35.4889315639,4.97757277822));
#55919=CARTESIAN_POINT('Ctrl Pts',(-4.53663898841,-35.2864927806,5.40585813039));
#55920=CARTESIAN_POINT('Ctrl Pts',(-4.5036945439,-35.3198754069,5.40486687422));
#55921=CARTESIAN_POINT('Ctrl Pts',(-4.4772847339,-35.3595850208,5.403864254));
#55922=CARTESIAN_POINT('Ctrl Pts',(-4.45905487062,-35.4039471568,5.40287237975));
#55923=CARTESIAN_POINT('Ctrl Pts',(-4.44995084219,-35.450642856,5.40192600583));
#55924=CARTESIAN_POINT('Ctrl Pts',(-4.44996438067,-35.4973385552,5.40106825188));
#55925=CARTESIAN_POINT('Ctrl Pts',(-4.49212121119,-35.2852060782,5.83250225872));
#55926=CARTESIAN_POINT('Ctrl Pts',(-4.45609896624,-35.3187908717,5.82727331029));
#55927=CARTESIAN_POINT('Ctrl Pts',(-4.42697004659,-35.3598847947,5.82278629135));
#55928=CARTESIAN_POINT('Ctrl Pts',(-4.40679132226,-35.4065868399,5.81933946513));
#55929=CARTESIAN_POINT('Ctrl Pts',(-4.39676913356,-35.4561050288,5.8171388925));
#55930=CARTESIAN_POINT('Ctrl Pts',(-4.39688476736,-35.5056232176,5.81623445774));
#55931=CARTESIAN_POINT('',(-3.27067489002724,-35.4637499841709,2.49153074894399));
#55932=CARTESIAN_POINT('',(-3.30528109761575,-35.2990851340947,2.45651115243885));
#55933=CARTESIAN_POINT('Origin',(-3.48386983245681,-35.4637516974525,2.2804588998513));
#55934=CARTESIAN_POINT('Ctrl Pts',(-3.30528109741,-35.2990851344,2.45651115251));
#55935=CARTESIAN_POINT('Ctrl Pts',(-3.52263014734,-35.2997786652,2.67764867799));
#55936=CARTESIAN_POINT('Ctrl Pts',(-3.71975032728,-35.2998840308,2.91888544948));
#55937=CARTESIAN_POINT('Ctrl Pts',(-3.89420210101,-35.2992579912,3.17776652664));
#55938=CARTESIAN_POINT('Ctrl Pts',(-4.25043308745,-35.2963608901,3.82861914207));
#55939=CARTESIAN_POINT('Ctrl Pts',(-4.45858902825,-35.291449905,4.54475674437));
#55940=CARTESIAN_POINT('Ctrl Pts',(-4.52558545037,-35.2885903077,4.9733945174));
#55941=CARTESIAN_POINT('Ctrl Pts',(-4.53663898841,-35.2864927806,5.40585813039));
#55942=CARTESIAN_POINT('Ctrl Pts',(-4.49212120371,-35.2852060782,5.83250225674));
#55943=CARTESIAN_POINT('Ctrl Pts',(-3.2706750272,-35.4637499833,2.49153088745));
#55944=CARTESIAN_POINT('Ctrl Pts',(-3.34813707187767,-35.4633621598035,
2.56977446344287));
#55945=CARTESIAN_POINT('Ctrl Pts',(-3.42304337318045,-35.4631429472603,
2.65189514109921));
#55946=CARTESIAN_POINT('Ctrl Pts',(-3.49496054014435,-35.463107855991,2.73777137044876));
#55947=CARTESIAN_POINT('Ctrl Pts',(-3.56711767566814,-35.4630726476315,
2.8239341460564));
#55948=CARTESIAN_POINT('Ctrl Pts',(-3.63626532925966,-35.4632228989124,
2.91387775343965));
#55949=CARTESIAN_POINT('Ctrl Pts',(-3.70196006654796,-35.4635695903925,
3.00742645561651));
#55950=CARTESIAN_POINT('Ctrl Pts',(-3.76774023884962,-35.4639167327395,
3.10109681646727));
#55951=CARTESIAN_POINT('Ctrl Pts',(-3.8300576443282,-35.4644609466404,3.19838101859501));
#55952=CARTESIAN_POINT('Ctrl Pts',(-3.88846922427447,-35.4652068351614,
3.29905040676408));
#55953=CARTESIAN_POINT('Ctrl Pts',(-3.9452868428507,-35.4659323695421,3.39697268355497));
#55954=CARTESIAN_POINT('Ctrl Pts',(-3.99840870171747,-35.4668488224885,
3.49809815904795));
#55955=CARTESIAN_POINT('Ctrl Pts',(-4.04743323499239,-35.4679527918964,
3.6021661231991));
#55956=CARTESIAN_POINT('Ctrl Pts',(-4.07131487842421,-35.4684905757773,
3.65286143525025));
#55957=CARTESIAN_POINT('Ctrl Pts',(-4.09422433966003,-35.4690727315529,
3.70425421846681));
#55958=CARTESIAN_POINT('Ctrl Pts',(-4.11611628683934,-35.4696980689031,
3.7563100790971));
#55959=CARTESIAN_POINT('Ctrl Pts',(-4.15139593057075,-35.470705822062,3.8401999314764));
#55960=CARTESIAN_POINT('Ctrl Pts',(-4.18403267406679,-35.4718258943186,
3.92581272262133));
#55961=CARTESIAN_POINT('Ctrl Pts',(-4.2138419733407,-35.4730506192599,4.01298809000643));
#55962=CARTESIAN_POINT('Ctrl Pts',(-4.21525776959202,-35.4731087877182,
4.01712849455661));
#55963=CARTESIAN_POINT('Ctrl Pts',(-4.21720500784041,-35.4731896392214,
4.02286090035683));
#55964=CARTESIAN_POINT('Ctrl Pts',(-4.21825549464136,-35.4732333631442,
4.02596768664432));
#55965=CARTESIAN_POINT('Ctrl Pts',(-4.21839192807396,-35.4732390418494,
4.02637118482935));
#55966=CARTESIAN_POINT('Ctrl Pts',(-4.21851330667239,-35.4732440920213,
4.02673037086751));
#55967=CARTESIAN_POINT('Ctrl Pts',(-4.2186165485839,-35.4732483811445,4.02703598966244));
#55968=CARTESIAN_POINT('Ctrl Pts',(-4.23183083826564,-35.4737973608668,
4.06615319729172));
#55969=CARTESIAN_POINT('Ctrl Pts',(-4.24548075738622,-35.474411102047,4.10854338064577));
#55970=CARTESIAN_POINT('Ctrl Pts',(-4.25925066744965,-35.4750969173758,
4.15428398502716));
#55971=CARTESIAN_POINT('Ctrl Pts',(-4.2727730646147,-35.4757704052354,4.1992024061472));
#55972=CARTESIAN_POINT('Ctrl Pts',(-4.28641108667379,-35.4765134451113,
4.24735239861612));
#55973=CARTESIAN_POINT('Ctrl Pts',(-4.2998170358193,-35.4773325193858,4.29879617118771));
#55974=CARTESIAN_POINT('Ctrl Pts',(-4.31304837859414,-35.4781409255916,
4.34956991209459));
#55975=CARTESIAN_POINT('Ctrl Pts',(-4.32605355488894,-35.4790234473957,
4.40355273662503));
#55976=CARTESIAN_POINT('Ctrl Pts',(-4.33845166412103,-35.4799851819289,
4.46078568264521));
#55977=CARTESIAN_POINT('Ctrl Pts',(-4.35057706096531,-35.4809257618718,
4.51675971627169));
#55978=CARTESIAN_POINT('Ctrl Pts',(-4.36212158350111,-35.4819421524447,
4.57584296420357));
#55979=CARTESIAN_POINT('Ctrl Pts',(-4.37268649070218,-35.4830373446617,
4.63804811399243));
#55980=CARTESIAN_POINT('Ctrl Pts',(-4.37771153255026,-35.4835582566411,
4.66763507343339));
#55981=CARTESIAN_POINT('Ctrl Pts',(-4.38251435031144,-35.4840969654634,
4.69792787163709));
#55982=CARTESIAN_POINT('Ctrl Pts',(-4.38704879694281,-35.4846536031822,
4.72892524743954));
#55983=CARTESIAN_POINT('Ctrl Pts',(-4.39625171328598,-35.4857833309696,
4.79183617782618));
#55984=CARTESIAN_POINT('Ctrl Pts',(-4.40435098438274,-35.4869880048322,
4.85764894737013));
#55985=CARTESIAN_POINT('Ctrl Pts',(-4.41093643203333,-35.488267734625,4.92633586345641));
#55986=CARTESIAN_POINT('Ctrl Pts',(-4.41730798087347,-35.4895058981198,
4.99279179230792));
#55987=CARTESIAN_POINT('Ctrl Pts',(-4.42226208806939,-35.4908143333423,
5.06193852712424));
#55988=CARTESIAN_POINT('Ctrl Pts',(-4.425397613255,-35.4921905896938,5.13371303089722));
#55989=CARTESIAN_POINT('Ctrl Pts',(-4.42847425789576,-35.4935410019781,
5.20413971520232));
#55990=CARTESIAN_POINT('Ctrl Pts',(-4.42979964382002,-35.4949567142392,
5.27709678642837));
#55991=CARTESIAN_POINT('Ctrl Pts',(-4.42897076191856,-35.4964327992564,
5.35248217910494));
#55992=CARTESIAN_POINT('Ctrl Pts',(-4.42816771303412,-35.4978628804589,
5.42551810302413));
#55993=CARTESIAN_POINT('Ctrl Pts',(-4.42534217899082,-35.499349607714,5.50083357556422));
#55994=CARTESIAN_POINT('Ctrl Pts',(-4.42011034884093,-35.5008861800709,
5.5782911933905));
#55995=CARTESIAN_POINT('Ctrl Pts',(-4.4148928306134,-35.5024185490605,5.65553692218727));
#55996=CARTESIAN_POINT('Ctrl Pts',(-4.40728176918284,-35.5040004542694,
5.73491352245175));
#55997=CARTESIAN_POINT('Ctrl Pts',(-4.39688476736,-35.5056232175999,5.81623445774));
#55998=CARTESIAN_POINT('Ctrl Pts',(-3.24268125491577,-35.2958973038634,
2.35935886017492));
#55999=CARTESIAN_POINT('Ctrl Pts',(-3.23323477285515,-35.3247273688969,
2.3897825108109));
#56000=CARTESIAN_POINT('Ctrl Pts',(-3.22952081745637,-35.3580485457362,
2.41773023191833));
#56001=CARTESIAN_POINT('Ctrl Pts',(-3.23194738647767,-35.3946308528826,
2.44189906566998));
#56002=CARTESIAN_POINT('Ctrl Pts',(-3.24040658365444,-35.43284772689,2.46121439404479));
#56003=CARTESIAN_POINT('Ctrl Pts',(-3.25430040542545,-35.4710646009975,
2.47508664859981));
#56004=CARTESIAN_POINT('Ctrl Pts',(-3.24863517715864,-35.2942729539699,
2.3701975687693));
#56005=CARTESIAN_POINT('Ctrl Pts',(-3.23915898528583,-35.3234246802185,
2.39878856453282));
#56006=CARTESIAN_POINT('Ctrl Pts',(-3.2350331221988,-35.3568426819669,2.42480698211996));
#56007=CARTESIAN_POINT('Ctrl Pts',(-3.23664595574859,-35.3933445979533,
2.44709362653317));
#56008=CARTESIAN_POINT('Ctrl Pts',(-3.24393136712945,-35.4313918582424,
2.46471330964264));
#56009=CARTESIAN_POINT('Ctrl Pts',(-3.25638336581306,-35.4694391186319,
2.47716637564742));
#56010=CARTESIAN_POINT('Ctrl Pts',(-3.2548709476279,-35.2930864761754,2.38098976678876));
#56011=CARTESIAN_POINT('Ctrl Pts',(-3.24525822198285,-35.3224889921552,
2.407755582698));
#56012=CARTESIAN_POINT('Ctrl Pts',(-3.24064139298909,-35.3559431246713,
2.43187281216271));
#56013=CARTESIAN_POINT('Ctrl Pts',(-3.24139525599044,-35.3923142407988,
2.45231077673936));
#56014=CARTESIAN_POINT('Ctrl Pts',(-3.2474923517538,-35.4301467373312,2.46825699792508));
#56015=CARTESIAN_POINT('Ctrl Pts',(-3.25850833911909,-35.4679792337635,
2.4792918557513));
#56016=CARTESIAN_POINT('Ctrl Pts',(-3.26132471448853,-35.2924161434336,
2.39170879431664));
#56017=CARTESIAN_POINT('Ctrl Pts',(-3.25147227203682,-35.3219985450907,
2.41665052924938));
#56018=CARTESIAN_POINT('Ctrl Pts',(-3.24628624189605,-35.3554285970707,
2.43888137042276));
#56019=CARTESIAN_POINT('Ctrl Pts',(-3.24613175788547,-35.3916164538002,
2.45749004094981));
#56020=CARTESIAN_POINT('Ctrl Pts',(-3.25101555797363,-35.4291873972929,
2.47177215112507));
#56021=CARTESIAN_POINT('Ctrl Pts',(-3.2605896658139,-35.4667583406855,2.481377904069));
#56022=CARTESIAN_POINT('Ctrl Pts',(-3.27381283591109,-35.2922258297676,
2.41169319642401));
#56023=CARTESIAN_POINT('Ctrl Pts',(-3.26330828363882,-35.3220055622133,
2.43319946208684));
#56024=CARTESIAN_POINT('Ctrl Pts',(-3.25689092113158,-35.3552658228255,
2.45190420521593));
#56025=CARTESIAN_POINT('Ctrl Pts',(-3.25491795867093,-35.3910088541773,
2.46708600579959));
#56026=CARTESIAN_POINT('Ctrl Pts',(-3.25746311070511,-35.4279936168047,
2.478225570397));
#56027=CARTESIAN_POINT('Ctrl Pts',(-3.26429697723892,-35.4649783794321,
2.48510059740241));
#56028=CARTESIAN_POINT('Ctrl Pts',(-3.28671058272193,-35.2940584356266,
2.43091393425374));
#56029=CARTESIAN_POINT('Ctrl Pts',(-3.27516135889415,-35.3237449318942,
2.44902623947939));
#56030=CARTESIAN_POINT('Ctrl Pts',(-3.26720601449316,-35.3565916803118,
2.46426478291748));
#56031=CARTESIAN_POINT('Ctrl Pts',(-3.26320423693874,-35.391677678938,2.47607271322631));
#56032=CARTESIAN_POINT('Ctrl Pts',(-3.26328413845668,-35.4278861002098,
2.48407552049272));
#56033=CARTESIAN_POINT('Ctrl Pts',(-3.26732385940126,-35.4640945215815,
2.48814889706368));
#56034=CARTESIAN_POINT('Ctrl Pts',(-3.29284930097053,-35.2953488394616,
2.43972797957268));
#56035=CARTESIAN_POINT('Ctrl Pts',(-3.28072374942692,-35.3249242484803,
2.45627460757783));
#56036=CARTESIAN_POINT('Ctrl Pts',(-3.27197784219537,-35.3575177795095,
2.46992291402891));
#56037=CARTESIAN_POINT('Ctrl Pts',(-3.26697872456239,-35.3922543161982,
2.48016821016769));
#56038=CARTESIAN_POINT('Ctrl Pts',(-3.26588739148542,-35.4280582492778,
2.4867007857863));
#56039=CARTESIAN_POINT('Ctrl Pts',(-3.26861320217918,-35.4638621823573,
2.48944916276422));
#56040=CARTESIAN_POINT('Ctrl Pts',(-3.29903564205108,-35.2970543501715,
2.44827686787325));
#56041=CARTESIAN_POINT('Ctrl Pts',(-3.28623988731176,-35.3264458529848,
2.46327459582849));
#56042=CARTESIAN_POINT('Ctrl Pts',(-3.27663206694421,-35.3587314714483,
2.47533376078653));
#56043=CARTESIAN_POINT('Ctrl Pts',(-3.27058251702853,-35.3930563620857,
2.48402805942754));
#56044=CARTESIAN_POINT('Ctrl Pts',(-3.26826827635479,-35.4284056459787,
2.4890983067967));
#56045=CARTESIAN_POINT('Ctrl Pts',(-3.26965563393973,-35.4637549298717,
2.49050120789989));
#56046=CARTESIAN_POINT('Ctrl Pts',(-3.30530033482775,-35.2990758150286,
2.45652194936013));
#56047=CARTESIAN_POINT('Ctrl Pts',(-3.29176525174297,-35.3282177516101,
2.47005157432767));
#56048=CARTESIAN_POINT('Ctrl Pts',(-3.28124477977141,-35.3601396973233,
2.48060908546945));
#56049=CARTESIAN_POINT('Ctrl Pts',(-3.27412082604265,-35.394022231877,2.48781273002727));
#56050=CARTESIAN_POINT('Ctrl Pts',(-3.27059928705473,-35.4288861031222,
2.4914543200214));
#56051=CARTESIAN_POINT('Ctrl Pts',(-3.27067686689488,-35.4637499744676,
2.49153274570348));
#56052=CARTESIAN_POINT('Ctrl Pts',(-3.24268782424592,-35.295907687789,2.35939289968608));
#56053=CARTESIAN_POINT('Ctrl Pts',(-3.25008684470559,-35.293890193334,2.37286023708758));
#56054=CARTESIAN_POINT('Ctrl Pts',(-3.25799757378118,-35.2927186181909,
2.38626991325058));
#56055=CARTESIAN_POINT('Ctrl Pts',(-3.26619360674797,-35.2925758914817,
2.39937991847623));
#56056=CARTESIAN_POINT('Ctrl Pts',(-3.26898632406456,-35.2925272587646,
2.40384702332593));
#56057=CARTESIAN_POINT('Ctrl Pts',(-3.27181181577843,-35.2925980792957,
2.4082795569164));
#56058=CARTESIAN_POINT('Ctrl Pts',(-3.27466035798211,-35.292795589977,2.41266929430184));
#56059=CARTESIAN_POINT('Ctrl Pts',(-3.2805841726001,-35.2932063322366,2.42179817098109));
#56060=CARTESIAN_POINT('Ctrl Pts',(-3.28660274669036,-35.2941627905457,
2.43072803182399));
#56061=CARTESIAN_POINT('Ctrl Pts',(-3.29270461274169,-35.2955791073848,
2.43934860706454));
#56062=CARTESIAN_POINT('Ctrl Pts',(-3.2968597946089,-35.2965435753031,2.44521895191039));
#56063=CARTESIAN_POINT('Ctrl Pts',(-3.30105340316511,-35.2977212882825,
2.45094670272042));
#56064=CARTESIAN_POINT('Ctrl Pts',(-3.30528109740205,-35.2990851343927,
2.45651115251783));
#56065=CARTESIAN_POINT('Origin',(-3.25603245768934,-35.4878985648969,2.47710123794777));
#56066=CARTESIAN_POINT('Origin',(-0.425321894002,-36.1242356128,5.30846337982));
#56067=CARTESIAN_POINT('',(-1.85962356625E-14,-36.1242356128,9.2896999221));
#56068=CARTESIAN_POINT('Origin',(0.425321894002,-36.1242356128,5.30846337982));
#56069=CARTESIAN_POINT('',(4.19434056524382,-35.5045435040676,6.6596263511468));
#56070=CARTESIAN_POINT('Ctrl Pts',(4.19434056523043,-35.5045435040781,6.65962635114224));
#56071=CARTESIAN_POINT('Ctrl Pts',(4.15305083902113,-35.50180461675,6.77480250110769));
#56072=CARTESIAN_POINT('Ctrl Pts',(4.10642935579663,-35.4989509433917,6.88821915911414));
#56073=CARTESIAN_POINT('Ctrl Pts',(4.05464196214409,-35.4960150956293,6.99937406998726));
#56074=CARTESIAN_POINT('Ctrl Pts',(4.00293218678962,-35.4930836480788,7.11036238326981));
#56075=CARTESIAN_POINT('Ctrl Pts',(3.94607207387214,-35.4900702722635,7.21909537875552));
#56076=CARTESIAN_POINT('Ctrl Pts',(3.88427619509728,-35.4870074333955,7.32508884382549));
#56077=CARTESIAN_POINT('Ctrl Pts',(3.82256508245509,-35.4839487958596,7.43093691641458));
#56078=CARTESIAN_POINT('Ctrl Pts',(3.75593187099409,-35.480840830876,7.53405263623836));
#56079=CARTESIAN_POINT('Ctrl Pts',(3.68463786454671,-35.4777158702413,7.63397461894421));
#56080=CARTESIAN_POINT('Ctrl Pts',(3.61346023977025,-35.4745960108509,7.73373348713474));
#56081=CARTESIAN_POINT('Ctrl Pts',(3.53763719705471,-35.4714592112521,7.83030872216152));
#56082=CARTESIAN_POINT('Ctrl Pts',(3.45747394171211,-35.4683376451628,7.92326682916533));
#56083=CARTESIAN_POINT('Ctrl Pts',(3.37739062673967,-35.4652191919604,8.01613223652201));
#56084=CARTESIAN_POINT('Ctrl Pts',(3.29297595264275,-35.4621159419002,8.1053874293973));
#56085=CARTESIAN_POINT('Ctrl Pts',(3.20457654052722,-35.4590599725433,8.19063039942675));
#56086=CARTESIAN_POINT('Ctrl Pts',(3.11627567267817,-35.4560074098636,8.27577834387001));
#56087=CARTESIAN_POINT('Ctrl Pts',(3.02399917934084,-35.4530020225324,8.35692273333336));
#56088=CARTESIAN_POINT('Ctrl Pts',(2.92813151663719,-35.4500757809538,8.43369730898203));
#56089=CARTESIAN_POINT('Ctrl Pts',(2.89703118657161,-35.4491264819266,8.45860367027196));
#56090=CARTESIAN_POINT('Ctrl Pts',(2.8655532088065,-35.448185512292,8.48305043444037));
#56091=CARTESIAN_POINT('Ctrl Pts',(2.83371152617554,-35.4472539635573,8.50702594740874));
#56092=CARTESIAN_POINT('Ctrl Pts',(2.73357926242005,-35.4443245303148,8.58242153551399));
#56093=CARTESIAN_POINT('Ctrl Pts',(2.62985289969705,-35.4415182005033,8.65314930294848));
#56094=CARTESIAN_POINT('Ctrl Pts',(2.52299764839741,-35.4388615158311,8.71887384610738));
#56095=CARTESIAN_POINT('Ctrl Pts',(2.4196792012438,-35.4362927648192,8.78242297126939));
#56096=CARTESIAN_POINT('Ctrl Pts',(2.31343605617025,-35.4338639166745,8.84129461962353));
#56097=CARTESIAN_POINT('Ctrl Pts',(2.20471825533705,-35.4315989638622,8.89522957075138));
#56098=CARTESIAN_POINT('Ctrl Pts',(2.09602580748759,-35.4293345392368,8.94915194425232));
#56099=CARTESIAN_POINT('Ctrl Pts',(1.98486018981476,-35.4272339335119,8.9981397472551));
#56100=CARTESIAN_POINT('Ctrl Pts',(1.87169528201999,-35.4253211223716,9.04198010558597));
#56101=CARTESIAN_POINT('Ctrl Pts',(1.75853751403165,-35.4234084319144,9.08581769793859));
#56102=CARTESIAN_POINT('Ctrl Pts',(1.64338105763938,-35.4216835123457,9.12450835777501));
#56103=CARTESIAN_POINT('Ctrl Pts',(1.52671874202298,-35.4201703348117,9.15788776566138));
#56104=CARTESIAN_POINT('Ctrl Pts',(1.41004394368312,-35.4186569953696,9.19127074510311));
#56105=CARTESIAN_POINT('Ctrl Pts',(1.29186332646816,-35.4173554432769,9.21934123844898));
#56106=CARTESIAN_POINT('Ctrl Pts',(1.1726835767396,-35.4162896573753,9.24198516497849));
#56107=CARTESIAN_POINT('Ctrl Pts',(1.05342866422859,-35.4152231993173,9.2646433722942));
#56108=CARTESIAN_POINT('Ctrl Pts',(0.93317372977555,-35.4143928049242,9.28186810641652));
#56109=CARTESIAN_POINT('Ctrl Pts',(0.81243462455955,-35.4138224984343,9.29359660883269));
#56110=CARTESIAN_POINT('Ctrl Pts',(0.691652882104724,-35.413251990549,9.30532925299696));
#56111=CARTESIAN_POINT('Ctrl Pts',(0.570387002637427,-35.4129417542919,
9.31156176915144));
#56112=CARTESIAN_POINT('Ctrl Pts',(0.449155981586392,-35.4129158393615,
9.31228343764101));
#56113=CARTESIAN_POINT('Ctrl Pts',(0.327819079588126,-35.4128899017975,
9.3130057364226));
#56114=CARTESIAN_POINT('Ctrl Pts',(0.206517472293906,-35.4131487824193,
9.308207582444));
#56115=CARTESIAN_POINT('Ctrl Pts',(0.0857684745831489,-35.4137165939942,
9.29793033600623));
#56116=CARTESIAN_POINT('Ctrl Pts',(0.0571457260649734,-35.4138511899595,
9.29549418294637));
#56117=CARTESIAN_POINT('Ctrl Pts',(0.0285540008339206,-35.414003144618,
9.29275039094128));
#56118=CARTESIAN_POINT('Ctrl Pts',(1.28564320530265E-7,-35.4141727791362,
9.28969993583948));
#56119=CARTESIAN_POINT('',(4.39688473843144,-35.505623218299,5.81623468041465));
#56120=CARTESIAN_POINT('Ctrl Pts',(4.39688470965,-35.505623219,5.81623490373));
#56121=CARTESIAN_POINT('Ctrl Pts',(4.38573643649444,-35.5073629552901,5.90343173345355));
#56122=CARTESIAN_POINT('Ctrl Pts',(4.37169824303641,-35.5085322020161,5.99037898434775));
#56123=CARTESIAN_POINT('Ctrl Pts',(4.35480069027969,-35.5091456409943,6.07679716182491));
#56124=CARTESIAN_POINT('Ctrl Pts',(4.33760460211872,-35.5097699178291,6.16474212166635));
#56125=CARTESIAN_POINT('Ctrl Pts',(4.31744838415589,-35.5098175202228,6.25213819810706));
#56126=CARTESIAN_POINT('Ctrl Pts',(4.29439012671324,-35.5092855518098,6.33873192964319));
#56127=CARTESIAN_POINT('Ctrl Pts',(4.28790249453768,-35.5091358780801,6.36309579496619));
#56128=CARTESIAN_POINT('Ctrl Pts',(4.28118522482724,-35.508940268535,6.3873964394));
#56129=CARTESIAN_POINT('Ctrl Pts',(4.27423977311736,-35.508698583756,6.41162895167755));
#56130=CARTESIAN_POINT('Ctrl Pts',(4.25993397822891,-35.5082007769869,6.46154152248722));
#56131=CARTESIAN_POINT('Ctrl Pts',(4.24466258667264,-35.5075078797346,6.51115697796593));
#56132=CARTESIAN_POINT('Ctrl Pts',(4.22844025810848,-35.5066170237349,6.56043545201076));
#56133=CARTESIAN_POINT('Ctrl Pts',(4.21772914646967,-35.5060288185319,6.59297253414401));
#56134=CARTESIAN_POINT('Ctrl Pts',(4.20660257847504,-35.5053541998305,6.62536529996203));
#56135=CARTESIAN_POINT('Ctrl Pts',(4.19507102909248,-35.5045918749017,6.65758701234463));
#56136=CARTESIAN_POINT('Ctrl Pts',(4.19482771075667,-35.504575789671,6.65826689786338));
#56137=CARTESIAN_POINT('Ctrl Pts',(4.19458421244928,-35.5045596653808,6.65894670632568));
#56138=CARTESIAN_POINT('Ctrl Pts',(4.1943405656018,-35.5045435041,6.65962635023499));
#56139=CARTESIAN_POINT('',(3.27067475303001,-35.4637499849021,2.49153061051667));
#56140=CARTESIAN_POINT('Ctrl Pts',(3.27067475303,-35.4637499849,2.49153061052));
#56141=CARTESIAN_POINT('Ctrl Pts',(3.48586067783,-35.4626726292,2.70888759263));
#56142=CARTESIAN_POINT('Ctrl Pts',(3.68047391974,-35.4626982735,2.94697615221));
#56143=CARTESIAN_POINT('Ctrl Pts',(3.85174834775,-35.4639143567,3.20314921651));
#56144=CARTESIAN_POINT('Ctrl Pts',(4.09456241628,-35.4679039697,3.65475367055));
#56145=CARTESIAN_POINT('Ctrl Pts',(4.26231352009,-35.4746596511,4.1374772467));
#56146=CARTESIAN_POINT('Ctrl Pts',(4.31696935237,-35.4777519322,4.33446216267));
#56147=CARTESIAN_POINT('Ctrl Pts',(4.40337102111,-35.4847566344,4.74599500874));
#56148=CARTESIAN_POINT('Ctrl Pts',(4.4353410064,-35.4927030817,5.16452779898));
#56149=CARTESIAN_POINT('Ctrl Pts',(4.43724557978,-35.4969389179,5.38040371826));
#56150=CARTESIAN_POINT('Ctrl Pts',(4.42458344919,-35.5012499248,5.59703086423));
#56151=CARTESIAN_POINT('Ctrl Pts',(4.3974872235,-35.5055288233,5.81150364203));
#56152=CARTESIAN_POINT('Ctrl Pts',(4.39728717711,-35.5055602891,5.81308076015));
#56153=CARTESIAN_POINT('Ctrl Pts',(4.39708635746,-35.5055917535,5.81465770549));
#56154=CARTESIAN_POINT('Ctrl Pts',(4.39688476668,-35.5056232176,5.81623445766));
#56155=CARTESIAN_POINT('',(3.25430421882,-35.4710616254,2.47509045608));
#56156=CARTESIAN_POINT('Origin',(3.25603245768934,-35.4878985648969,2.47710123794777));
#56157=CARTESIAN_POINT('',(3.25430421882,-36.1242356128,2.47509045608));
#56158=CARTESIAN_POINT('Origin',(3.46627170195,-36.1242356128,2.26279399804));
#56159=CARTESIAN_POINT('',(3.16691857253,-35.4710616262,2.28248419619));
#56160=CARTESIAN_POINT('Origin',(3.46627170195,-35.4710616316899,2.26279399804));
#56161=CARTESIAN_POINT('',(3.16691857253,-35.9226486195,2.28248419619));
#56162=CARTESIAN_POINT('Origin',(3.0399446742,-32.4742356128,0.352080371467));
#56163=CARTESIAN_POINT('',(3.16549337405758,-35.4651789109462,2.26081668330539));
#56164=CARTESIAN_POINT('Origin',(3.16701457909211,-35.4948316439558,2.28394383708707));
#56165=CARTESIAN_POINT('',(3.04626146311845,-35.4033959728417,0.448115484591892));
#56166=CARTESIAN_POINT('Ctrl Pts',(3.04626151745,-35.4033927946,0.44811631692));
#56167=CARTESIAN_POINT('Ctrl Pts',(3.05294917186292,-35.4075920678871,0.549789759532655));
#56168=CARTESIAN_POINT('Ctrl Pts',(3.05964380945705,-35.4116947932727,0.651569369125622));
#56169=CARTESIAN_POINT('Ctrl Pts',(3.06633992560627,-35.415674424655,0.753371458620647));
#56170=CARTESIAN_POINT('Ctrl Pts',(3.07076632608472,-35.4183051201002,0.820666709719334));
#56171=CARTESIAN_POINT('Ctrl Pts',(3.07519346050157,-35.4208822031627,0.887973119277254));
#56172=CARTESIAN_POINT('Ctrl Pts',(3.07962053317529,-35.4233996000391,0.955278587451633));
#56173=CARTESIAN_POINT('Ctrl Pts',(3.08757598305295,-35.4279233623867,1.07622651806314));
#56174=CARTESIAN_POINT('Ctrl Pts',(3.0955499343282,-35.4322756333094,1.19745572859887));
#56175=CARTESIAN_POINT('Ctrl Pts',(3.10353553487434,-35.436446582721,1.3188620493187));
#56176=CARTESIAN_POINT('Ctrl Pts',(3.11356049330208,-35.4416827066937,1.47127304346359));
#56177=CARTESIAN_POINT('Ctrl Pts',(3.12360407993767,-35.4466333489527,1.62396725231241));
#56178=CARTESIAN_POINT('Ctrl Pts',(3.13365681361421,-35.4513048687405,1.77680052285555));
#56179=CARTESIAN_POINT('Ctrl Pts',(3.14185238055679,-35.4551133604778,1.90139899925928));
#56180=CARTESIAN_POINT('Ctrl Pts',(3.15005425524475,-35.458737299182,2.02609337075221));
#56181=CARTESIAN_POINT('Ctrl Pts',(3.15825582228838,-35.4621835807124,2.15078306376021));
#56182=CARTESIAN_POINT('Ctrl Pts',(3.16011434868278,-35.4629645296643,2.17903852815273));
#56183=CARTESIAN_POINT('Ctrl Pts',(3.16197284588703,-35.4637363447115,2.20729354873459));
#56184=CARTESIAN_POINT('Ctrl Pts',(3.16383120921193,-35.4644990738493,2.23554653393125));
#56185=CARTESIAN_POINT('Ctrl Pts',(3.16438523801469,-35.4647264642123,2.24396951955144));
#56186=CARTESIAN_POINT('Ctrl Pts',(3.16493929387688,-35.4649530731761,2.25239291656041));
#56187=CARTESIAN_POINT('Ctrl Pts',(3.16549337399,-35.4651789177,2.26081668226));
#56188=CARTESIAN_POINT('',(3.0462613877,-36.1242356128,0.448114344193));
#56189=CARTESIAN_POINT('Origin',(2.74690825827,-36.1242356128,0.467804542343));
#56190=CARTESIAN_POINT('',(3.04580294830778,-35.403525641014,0.442075686711352));
#56191=CARTESIAN_POINT('Origin',(2.97884827228343,-36.1481218195378,0.517617073024758));
#56192=CARTESIAN_POINT('',(2.97642257187428,-35.4237537116948,0.274612461594352));
#56193=CARTESIAN_POINT('Ctrl Pts',(2.97642257183112,-35.4237537093279,0.274612461466193));
#56194=CARTESIAN_POINT('Ctrl Pts',(2.98268497977946,-35.4228712901646,0.282052265727931));
#56195=CARTESIAN_POINT('Ctrl Pts',(2.98861404818367,-35.4219372537485,0.289833403879586));
#56196=CARTESIAN_POINT('Ctrl Pts',(2.99415416837544,-35.4209522031331,0.297895150451187));
#56197=CARTESIAN_POINT('Ctrl Pts',(2.99845521021089,-35.4201874645066,0.304153843055496));
#56198=CARTESIAN_POINT('Ctrl Pts',(3.00252275175911,-35.419393257241,0.310582180982538));
#56199=CARTESIAN_POINT('Ctrl Pts',(3.0063416756095,-35.418580198429,0.317158978249665));
#56200=CARTESIAN_POINT('Ctrl Pts',(3.01229565803106,-35.4173125800988,0.327412687632905));
#56201=CARTESIAN_POINT('Ctrl Pts',(3.0176461231883,-35.4160018511495,0.338028142723121));
#56202=CARTESIAN_POINT('Ctrl Pts',(3.02235637061599,-35.4146845316183,0.348942894945375));
#56203=CARTESIAN_POINT('Ctrl Pts',(3.02459478869408,-35.4140585110326,0.354129836622479));
#56204=CARTESIAN_POINT('Ctrl Pts',(3.02668885469369,-35.4134305994858,0.359384645117005));
#56205=CARTESIAN_POINT('Ctrl Pts',(3.0286346903702,-35.4128001572719,0.364701596418767));
#56206=CARTESIAN_POINT('Ctrl Pts',(3.03270900261687,-35.4114800979968,0.375834561070054));
#56207=CARTESIAN_POINT('Ctrl Pts',(3.03613450666436,-35.4101527558927,0.387242594903746));
#56208=CARTESIAN_POINT('Ctrl Pts',(3.03887458843745,-35.4087853617665,0.398842878730332));
#56209=CARTESIAN_POINT('Ctrl Pts',(3.040216923218,-35.4081154909939,0.404525725351026));
#56210=CARTESIAN_POINT('Ctrl Pts',(3.04139473737179,-35.4074348945344,0.410254824444013));
#56211=CARTESIAN_POINT('Ctrl Pts',(3.04240435417873,-35.4067400123833,0.416016088194172));
#56212=CARTESIAN_POINT('Ctrl Pts',(3.04355345657699,-35.4059491274249,0.422573310644067));
#56213=CARTESIAN_POINT('Ctrl Pts',(3.04448461205505,-35.4051386165017,0.429172218461528));
#56214=CARTESIAN_POINT('Ctrl Pts',(3.0451946497264,-35.4043135059583,0.435785984618936));
#56215=CARTESIAN_POINT('Ctrl Pts',(3.04531298939742,-35.4041759874657,0.436888279529325));
#56216=CARTESIAN_POINT('Ctrl Pts',(3.04542519152073,-35.4040380979892,0.437990972110662));
#56217=CARTESIAN_POINT('Ctrl Pts',(3.04553124611257,-35.4038999032468,0.439093919456291));
#56218=CARTESIAN_POINT('Ctrl Pts',(3.04562679829713,-35.4037753936965,0.440087643787353));
#56219=CARTESIAN_POINT('Ctrl Pts',(3.04571743289771,-35.4036505377665,0.441082415444004));
#56220=CARTESIAN_POINT('Ctrl Pts',(3.04580293259,-35.4035256929,0.442075691324));
#56221=CARTESIAN_POINT('',(2.97642257165,-36.1242356128,0.274612461872));
#56222=CARTESIAN_POINT('Origin',(-1.14194680047E-14,-36.1242356128,2.77999550541));
#56223=CARTESIAN_POINT('',(2.97099134009343,-35.4239899492211,0.268174258363064));
#56224=CARTESIAN_POINT('Origin',(-0.668003013044919,-15.7697206409511,-2.44335760989475));
#56225=CARTESIAN_POINT('',(1.05706468499156E-8,-35.5025703486183,-1.11050957416386));
#56226=CARTESIAN_POINT('Ctrl Pts',(2.35228951035953E-7,-35.502578684161,
-1.11051031257002));
#56227=CARTESIAN_POINT('Ctrl Pts',(0.241185384589035,-35.4960792051353,
-1.11050007271629));
#56228=CARTESIAN_POINT('Ctrl Pts',(0.484484691878602,-35.4895467242639,
-1.09177342402401));
#56229=CARTESIAN_POINT('Ctrl Pts',(0.724399361223006,-35.4822690330674,
-1.05406906565677));
#56230=CARTESIAN_POINT('Ctrl Pts',(1.38288114101671,-35.4625880852057,-0.897498063662974));
#56231=CARTESIAN_POINT('Ctrl Pts',(1.99837189146,-35.4437584036,-0.600230058024));
#56232=CARTESIAN_POINT('Ctrl Pts',(2.36450092427,-35.4339226943,-0.355565614957));
#56233=CARTESIAN_POINT('Ctrl Pts',(2.69092668038,-35.4272067546,-0.063087197317));
#56234=CARTESIAN_POINT('Ctrl Pts',(2.97099133973,-35.4239899499,0.268174257969));
#56235=CARTESIAN_POINT('',(-2.97099136809806,-35.4239899489092,0.268174291485618));
#56236=CARTESIAN_POINT('Ctrl Pts',(1.28924120788854E-7,-35.5025659486026,
-1.11050920496303));
#56237=CARTESIAN_POINT('Ctrl Pts',(-0.0429285569203519,-35.501411371073,
-1.1105075801006));
#56238=CARTESIAN_POINT('Ctrl Pts',(-0.0888321496125025,-35.5001747157574,
-1.10979779951855));
#56239=CARTESIAN_POINT('Ctrl Pts',(-0.13767716483008,-35.4988459736367,
-1.10806788123278));
#56240=CARTESIAN_POINT('Ctrl Pts',(-0.187515186117301,-35.4974902185449,
-1.10630279417186));
#56241=CARTESIAN_POINT('Ctrl Pts',(-0.240415157899067,-35.496038308208,
-1.10347576735259));
#56242=CARTESIAN_POINT('Ctrl Pts',(-0.296310996488047,-35.4944803392224,
-1.09921026463204));
#56243=CARTESIAN_POINT('Ctrl Pts',(-0.319133473410654,-35.4938442147431,
-1.09746864414901));
#56244=CARTESIAN_POINT('Ctrl Pts',(-0.342455076056133,-35.49319044283,-1.0954866896958));
#56245=CARTESIAN_POINT('Ctrl Pts',(-0.366270077451304,-35.4925185684443,
-1.09323663399743));
#56246=CARTESIAN_POINT('Ctrl Pts',(-0.427112374729311,-35.4908020713328,
-1.08748821704709));
#56247=CARTESIAN_POINT('Ctrl Pts',(-0.49117761483286,-35.4889758457042,
-1.07999285810841));
#56248=CARTESIAN_POINT('Ctrl Pts',(-0.558324085371852,-35.4870390748949,
-1.07025766102687));
#56249=CARTESIAN_POINT('Ctrl Pts',(-0.56804788363689,-35.4867586019455,
-1.06884786105181));
#56250=CARTESIAN_POINT('Ctrl Pts',(-0.577836253131251,-35.4864758297699,
-1.06739101520041));
#56251=CARTESIAN_POINT('Ctrl Pts',(-0.58768871401166,-35.4861907759962,
-1.06588555345568));
#56252=CARTESIAN_POINT('Ctrl Pts',(-0.626632411505944,-35.4850640475507,
-1.0599349338605));
#56253=CARTESIAN_POINT('Ctrl Pts',(-0.666576942127623,-35.4839012711429,
-1.05322514711936));
#56254=CARTESIAN_POINT('Ctrl Pts',(-0.707485482952031,-35.482702446971,
-1.04565773996551));
#56255=CARTESIAN_POINT('Ctrl Pts',(-0.727939753364235,-35.482103034885,
-1.04187403638858));
#56256=CARTESIAN_POINT('Ctrl Pts',(-0.748635013460178,-35.4814946108542,
-1.03787586244271));
#56257=CARTESIAN_POINT('Ctrl Pts',(-0.769565863763876,-35.4808771748401,
-1.03365067292279));
#56258=CARTESIAN_POINT('Ctrl Pts',(-0.780031288915725,-35.480568456833,
-1.03153807816284));
#56259=CARTESIAN_POINT('Ctrl Pts',(-0.790555611097553,-35.4802574858298,
-1.02936872577934));
#56260=CARTESIAN_POINT('Ctrl Pts',(-0.801138124773163,-35.4799442618238,
-1.02714103006202));
#56261=CARTESIAN_POINT('Ctrl Pts',(-0.809329380747585,-35.4797018148883,
-1.02541671139699));
#56262=CARTESIAN_POINT('Ctrl Pts',(-0.8167401543102,-35.4794822111352,-1.02383326583324));
#56263=CARTESIAN_POINT('Ctrl Pts',(-0.825263582189491,-35.4792289838017,
-1.0219824928238));
#56264=CARTESIAN_POINT('Ctrl Pts',(-0.827751810200008,-35.4791550596302,
-1.02144220019642));
#56265=CARTESIAN_POINT('Ctrl Pts',(-0.830334803420739,-35.4790782692507,
-1.02087881128024));
#56266=CARTESIAN_POINT('Ctrl Pts',(-0.833059501712441,-35.4789972063979,
-1.02028131764937));
#56267=CARTESIAN_POINT('Ctrl Pts',(-0.896234129185903,-35.4771176898513,
-1.00642788012826));
#56268=CARTESIAN_POINT('Ctrl Pts',(-0.956086609344959,-35.4753254377988,
-0.991656089473372));
#56269=CARTESIAN_POINT('Ctrl Pts',(-1.01266007696826,-35.4736283141261,
-0.976403962012024));
#56270=CARTESIAN_POINT('Ctrl Pts',(-1.06934213433761,-35.4719279329152,
-0.961122558907563));
#56271=CARTESIAN_POINT('Ctrl Pts',(-1.12273264082248,-35.4703228587348,
-0.945359005522279));
#56272=CARTESIAN_POINT('Ctrl Pts',(-1.17288344770512,-35.4688128161094,
-0.929502923302393));
#56273=CARTESIAN_POINT('Ctrl Pts',(-1.18001070035384,-35.4685982142721,
-0.927249513815593));
#56274=CARTESIAN_POINT('Ctrl Pts',(-1.18707253564867,-35.4683855215034,
-0.92499415151587));
#56275=CARTESIAN_POINT('Ctrl Pts',(-1.19406911857269,-35.4681747277853,
-0.922737871423588));
#56276=CARTESIAN_POINT('Ctrl Pts',(-1.23876490132943,-35.4668281289759,
-0.908324234661447));
#56277=CARTESIAN_POINT('Ctrl Pts',(-1.28079731020406,-35.465559275466,-0.893875904218736));
#56278=CARTESIAN_POINT('Ctrl Pts',(-1.3202373196139,-35.4643698991371,-0.879643438297542));
#56279=CARTESIAN_POINT('Ctrl Pts',(-1.36483738969774,-35.4630249129564,
-0.863548894025125));
#56280=CARTESIAN_POINT('Ctrl Pts',(-1.40611459487719,-35.4617817653164,
-0.847734025493257));
#56281=CARTESIAN_POINT('Ctrl Pts',(-1.44416237838903,-35.460639586592,-0.832516813766869));
#56282=CARTESIAN_POINT('Ctrl Pts',(-1.48259275197378,-35.4594859226719,
-0.817146585133672));
#56283=CARTESIAN_POINT('Ctrl Pts',(-1.51772886531389,-35.4584351742648,
-0.802386075087822));
#56284=CARTESIAN_POINT('Ctrl Pts',(-1.54966719455541,-35.4574841305407,
-0.788509495887233));
#56285=CARTESIAN_POINT('Ctrl Pts',(-1.57705388851693,-35.4566686231539,
-0.776610513165711));
#56286=CARTESIAN_POINT('Ctrl Pts',(-1.60208946323774,-35.455926364652,-0.76536053708072));
#56287=CARTESIAN_POINT('Ctrl Pts',(-1.62483092434311,-35.4552547109233,
-0.75490221309079));
#56288=CARTESIAN_POINT('Ctrl Pts',(-1.62604898179027,-35.4552187364174,
-0.754342053857323));
#56289=CARTESIAN_POINT('Ctrl Pts',(-1.62726045663906,-35.4551829644016,
-0.753784159209078));
#56290=CARTESIAN_POINT('Ctrl Pts',(-1.62846535718975,-35.4551473944535,
-0.753228548869446));
#56291=CARTESIAN_POINT('Ctrl Pts',(-1.62907016078648,-35.4551295400068,
-0.752949658523185));
#56292=CARTESIAN_POINT('Ctrl Pts',(-1.62940227027742,-35.4551197369896,
-0.752796401278891));
#56293=CARTESIAN_POINT('Ctrl Pts',(-1.62986987180753,-35.4551059353078,
-0.752580552869857));
#56294=CARTESIAN_POINT('Ctrl Pts',(-1.63010321593046,-35.4550990479451,
-0.752472839454802));
#56295=CARTESIAN_POINT('Ctrl Pts',(-1.63037029720969,-35.4550911650331,
-0.752349530937011));
#56296=CARTESIAN_POINT('Ctrl Pts',(-1.63072180996005,-35.4550807909207,
-0.752187167151381));
#56297=CARTESIAN_POINT('Ctrl Pts',(-1.63091011889002,-35.455075233404,-0.752100187231861));
#56298=CARTESIAN_POINT('Ctrl Pts',(-1.63112265799355,-35.455068960974,-0.752001998070547));
#56299=CARTESIAN_POINT('Ctrl Pts',(-1.63136721640979,-35.4550617439627,
-0.751888982288285));
#56300=CARTESIAN_POINT('Ctrl Pts',(-1.63155281040024,-35.4550562670139,
-0.751803215254229));
#56301=CARTESIAN_POINT('Ctrl Pts',(-1.63175684491654,-35.4550502460645,
-0.751708909138482));
#56302=CARTESIAN_POINT('Ctrl Pts',(-1.63198272234932,-35.4550435808507,
-0.75160447847866));
#56303=CARTESIAN_POINT('Ctrl Pts',(-1.63212306043723,-35.4550394397404,
-0.751539595506779));
#56304=CARTESIAN_POINT('Ctrl Pts',(-1.63226874903872,-35.4550351408601,
-0.751472228292576));
#56305=CARTESIAN_POINT('Ctrl Pts',(-1.63241217610713,-35.4550309088282,
-0.751405896014871));
#56306=CARTESIAN_POINT('Ctrl Pts',(-1.72111413665979,-35.4524136237535,
-0.710382934689245));
#56307=CARTESIAN_POINT('Ctrl Pts',(-1.80669687851978,-35.4499330427393,
-0.666746612081371));
#56308=CARTESIAN_POINT('Ctrl Pts',(-1.88910495946924,-35.4476091955558,
-0.620961007577427));
#56309=CARTESIAN_POINT('Ctrl Pts',(-1.97097206739186,-35.4453006034132,
-0.575475965551931));
#56310=CARTESIAN_POINT('Ctrl Pts',(-2.04970609269493,-35.4431465042315,
-0.527870081781686));
#56311=CARTESIAN_POINT('Ctrl Pts',(-2.12529624088428,-35.4411565189214,
-0.47857300423023));
#56312=CARTESIAN_POINT('Ctrl Pts',(-2.20107691690407,-35.4391615177779,
-0.429151671528354));
#56313=CARTESIAN_POINT('Ctrl Pts',(-2.27369798971146,-35.4373313167143,
-0.378030843835462));
#56314=CARTESIAN_POINT('Ctrl Pts',(-2.34319122334006,-35.4356679682213,
-0.325613711291171));
#56315=CARTESIAN_POINT('Ctrl Pts',(-2.41869584596948,-35.4338607347151,
-0.2686623276036));
#56316=CARTESIAN_POINT('Ctrl Pts',(-2.49051042940222,-35.4322503580634,
-0.210179038333438));
#56317=CARTESIAN_POINT('Ctrl Pts',(-2.55871897458397,-35.4308321175166,
-0.15064584251512));
#56318=CARTESIAN_POINT('Ctrl Pts',(-2.6234258658855,-35.4294866858459,-0.0941689301226338));
#56319=CARTESIAN_POINT('Ctrl Pts',(-2.68488662251831,-35.4283140496414,
-0.0367481610854193));
#56320=CARTESIAN_POINT('Ctrl Pts',(-2.74321026116799,-35.4273054357926,
0.021236660147039));
#56321=CARTESIAN_POINT('Ctrl Pts',(-2.80304899701284,-35.4262706207663,
0.080727776975007));
#56322=CARTESIAN_POINT('Ctrl Pts',(-2.85958585165633,-35.4254083825495,
0.14081243092363));
#56323=CARTESIAN_POINT('Ctrl Pts',(-2.9129769049787,-35.4247056624346,0.2011197359036));
#56324=CARTESIAN_POINT('Ctrl Pts',(-2.93274284262472,-35.4244455079497,
0.22344614371272));
#56325=CARTESIAN_POINT('Ctrl Pts',(-2.95207797270929,-35.4242071876201,
0.24580346143632));
#56326=CARTESIAN_POINT('Ctrl Pts',(-2.97099133978,-35.4239899499,0.268174257926));
#56327=CARTESIAN_POINT('',(-2.97642257185497,-35.4237537116948,0.274612461610598));
#56328=CARTESIAN_POINT('Origin',(0.668003013044919,-15.7697206409511,-2.44335760989475));
#56329=CARTESIAN_POINT('',(-2.97642257165,-36.1242356128,0.274612461872));
#56330=CARTESIAN_POINT('Origin',(-2.74690825827,-36.1242356128,0.467804542343));
#56331=CARTESIAN_POINT('',(-3.04580294830777,-35.403525641014,0.442075686711237));
#56332=CARTESIAN_POINT('Ctrl Pts',(-2.97642257183112,-35.4237537093279,
0.274612461466193));
#56333=CARTESIAN_POINT('Ctrl Pts',(-2.98268497977946,-35.4228712901646,
0.282052265727931));
#56334=CARTESIAN_POINT('Ctrl Pts',(-2.98861404818367,-35.4219372537485,
0.289833403879585));
#56335=CARTESIAN_POINT('Ctrl Pts',(-2.99415416837544,-35.4209522031331,
0.297895150451187));
#56336=CARTESIAN_POINT('Ctrl Pts',(-2.99845521021089,-35.4201874645066,
0.304153843055496));
#56337=CARTESIAN_POINT('Ctrl Pts',(-3.00252275175911,-35.419393257241,0.310582180982538));
#56338=CARTESIAN_POINT('Ctrl Pts',(-3.0063416756095,-35.418580198429,0.317158978249665));
#56339=CARTESIAN_POINT('Ctrl Pts',(-3.01229565803106,-35.4173125800988,
0.327412687632905));
#56340=CARTESIAN_POINT('Ctrl Pts',(-3.0176461231883,-35.4160018511495,0.338028142723121));
#56341=CARTESIAN_POINT('Ctrl Pts',(-3.02235637061599,-35.4146845316183,
0.348942894945375));
#56342=CARTESIAN_POINT('Ctrl Pts',(-3.02459478869408,-35.4140585110326,
0.354129836622479));
#56343=CARTESIAN_POINT('Ctrl Pts',(-3.02668885469369,-35.4134305994858,
0.359384645117005));
#56344=CARTESIAN_POINT('Ctrl Pts',(-3.0286346903702,-35.4128001572719,0.364701596418767));
#56345=CARTESIAN_POINT('Ctrl Pts',(-3.03270900261686,-35.4114800979968,
0.375834561070049));
#56346=CARTESIAN_POINT('Ctrl Pts',(-3.03613450666436,-35.4101527558927,
0.387242594903735));
#56347=CARTESIAN_POINT('Ctrl Pts',(-3.03887458843745,-35.4087853617665,
0.398842878730315));
#56348=CARTESIAN_POINT('Ctrl Pts',(-3.04021692321799,-35.4081154909939,
0.404525725351014));
#56349=CARTESIAN_POINT('Ctrl Pts',(-3.04139473737179,-35.4074348945344,
0.410254824444007));
#56350=CARTESIAN_POINT('Ctrl Pts',(-3.04240435417873,-35.4067400123833,
0.416016088194172));
#56351=CARTESIAN_POINT('Ctrl Pts',(-3.04355345657699,-35.4059491274249,
0.422573310644067));
#56352=CARTESIAN_POINT('Ctrl Pts',(-3.04448461205505,-35.4051386165017,
0.429172218461528));
#56353=CARTESIAN_POINT('Ctrl Pts',(-3.0451946497264,-35.4043135059583,0.435785984618936));
#56354=CARTESIAN_POINT('Ctrl Pts',(-3.04531298939742,-35.4041759874657,
0.436888279529325));
#56355=CARTESIAN_POINT('Ctrl Pts',(-3.04542519152073,-35.4040380979892,
0.437990972110662));
#56356=CARTESIAN_POINT('Ctrl Pts',(-3.04553124611257,-35.4038999032468,
0.439093919456291));
#56357=CARTESIAN_POINT('Ctrl Pts',(-3.04562679829713,-35.4037753936965,
0.440087643787354));
#56358=CARTESIAN_POINT('Ctrl Pts',(-3.04571743289771,-35.4036505377665,
0.441082415444004));
#56359=CARTESIAN_POINT('Ctrl Pts',(-3.04580293259,-35.4035256929,0.442075691324));
#56360=CARTESIAN_POINT('',(-3.04626146311845,-35.4033959728417,0.448115484591892));
#56361=CARTESIAN_POINT('Origin',(-2.97884827228343,-36.1481218195378,0.517617073024758));
#56362=CARTESIAN_POINT('',(-3.0462613877,-35.8888189474,0.448114344193));
#56363=CARTESIAN_POINT('Origin',(-3.0399446742,-32.4742356128,0.352080371467));
#56364=CARTESIAN_POINT('',(-3.16549337405758,-35.4651789109462,2.2608166833054));
#56365=CARTESIAN_POINT('Ctrl Pts',(-3.04626151745,-35.4033927946,0.44811631692));
#56366=CARTESIAN_POINT('Ctrl Pts',(-3.05294917186292,-35.4075920678871,
0.54978975953267));
#56367=CARTESIAN_POINT('Ctrl Pts',(-3.05964380945705,-35.4116947932727,
0.651569369125652));
#56368=CARTESIAN_POINT('Ctrl Pts',(-3.06633992560627,-35.415674424655,0.753371458620691));
#56369=CARTESIAN_POINT('Ctrl Pts',(-3.07076632608472,-35.4183051201002,
0.820666709719363));
#56370=CARTESIAN_POINT('Ctrl Pts',(-3.07519346050157,-35.4208822031628,
0.887973119277269));
#56371=CARTESIAN_POINT('Ctrl Pts',(-3.07962053317529,-35.4233996000391,
0.955278587451633));
#56372=CARTESIAN_POINT('Ctrl Pts',(-3.08757598305296,-35.4279233623867,
1.07622651806343));
#56373=CARTESIAN_POINT('Ctrl Pts',(-3.09554993432824,-35.4322756333094,
1.19745572859944));
#56374=CARTESIAN_POINT('Ctrl Pts',(-3.1035355348744,-35.436446582721,1.31886204931956));
#56375=CARTESIAN_POINT('Ctrl Pts',(-3.11356049330213,-35.4416827066937,
1.4712730434643));
#56376=CARTESIAN_POINT('Ctrl Pts',(-3.12360407993771,-35.4466333489527,
1.62396725231298));
#56377=CARTESIAN_POINT('Ctrl Pts',(-3.13365681361424,-35.4513048687405,
1.77680052285598));
#56378=CARTESIAN_POINT('Ctrl Pts',(-3.14185238055683,-35.4551133604778,
1.90139899925985));
#56379=CARTESIAN_POINT('Ctrl Pts',(-3.1500542552448,-35.458737299182,2.02609337075293));
#56380=CARTESIAN_POINT('Ctrl Pts',(-3.15825582228844,-35.4621835807125,
2.15078306376108));
#56381=CARTESIAN_POINT('Ctrl Pts',(-3.16011434868282,-35.4629645296644,
2.1790385281533));
#56382=CARTESIAN_POINT('Ctrl Pts',(-3.16197284588705,-35.4637363447115,
2.20729354873488));
#56383=CARTESIAN_POINT('Ctrl Pts',(-3.16383120921194,-35.4644990738493,
2.23554653393125));
#56384=CARTESIAN_POINT('Ctrl Pts',(-3.16438523801469,-35.4647264642123,
2.24396951955144));
#56385=CARTESIAN_POINT('Ctrl Pts',(-3.16493929387688,-35.4649530731761,
2.25239291656041));
#56386=CARTESIAN_POINT('Ctrl Pts',(-3.16549337399,-35.4651789177,2.26081668226));
#56387=CARTESIAN_POINT('Origin',(-3.16701457909211,-35.4948316439558,2.28394383708707));
#56388=CARTESIAN_POINT('Ctrl Pts',(-3.21673308013,-35.297826519,2.26193293676));
#56389=CARTESIAN_POINT('Ctrl Pts',(-3.19690170746,-35.3272920967,2.26244743731));
#56390=CARTESIAN_POINT('Ctrl Pts',(-3.18141841353,-35.3596904513,2.26259731642));
#56391=CARTESIAN_POINT('Ctrl Pts',(-3.17086410369,-35.3941615562,2.26236742048));
#56392=CARTESIAN_POINT('Ctrl Pts',(-3.16555572757,-35.4296702319,2.26176465335));
#56393=CARTESIAN_POINT('Ctrl Pts',(-3.16549338332,-35.4651789077,2.26081682416));
#56394=CARTESIAN_POINT('Ctrl Pts',(-3.22044227874,-35.2947170616,2.28115435818));
#56395=CARTESIAN_POINT('Ctrl Pts',(-3.19950860612,-35.3245433432,2.27888894627));
#56396=CARTESIAN_POINT('Ctrl Pts',(-3.18307576937,-35.3575027832,2.27596054224));
#56397=CARTESIAN_POINT('Ctrl Pts',(-3.17178564006,-35.3926825601,2.27243438801));
#56398=CARTESIAN_POINT('Ctrl Pts',(-3.16599327189,-35.4289738974,2.26841670742));
#56399=CARTESIAN_POINT('Ctrl Pts',(-3.16570519157,-35.4652652348,2.26403697776));
#56400=CARTESIAN_POINT('Ctrl Pts',(-3.22504500396,-35.2927962885,2.30073764763));
#56401=CARTESIAN_POINT('Ctrl Pts',(-3.20268941154,-35.3227611226,2.2957495854));
#56402=CARTESIAN_POINT('Ctrl Pts',(-3.18504154424,-35.3561044246,2.28975874044));
#56403=CARTESIAN_POINT('Ctrl Pts',(-3.1728278134,-35.3918504917,2.28291889281));
#56404=CARTESIAN_POINT('Ctrl Pts',(-3.16645576111,-35.428799749,2.27544850897));
#56405=CARTESIAN_POINT('Ctrl Pts',(-3.16593909074,-35.4657490064,2.26759298308));
#56406=CARTESIAN_POINT('Ctrl Pts',(-3.23041275638,-35.292377214,2.32058136088));
#56407=CARTESIAN_POINT('Ctrl Pts',(-3.20637961829,-35.3222393286,2.31311572454));
#56408=CARTESIAN_POINT('Ctrl Pts',(-3.18729883271,-35.3557626768,2.30425560397));
#56409=CARTESIAN_POINT('Ctrl Pts',(-3.1740077501,-35.391902145,2.29425266577));
#56410=CARTESIAN_POINT('Ctrl Pts',(-3.16698247964,-35.4293517376,2.28345602024));
#56411=CARTESIAN_POINT('Ctrl Pts',(-3.16624513219,-35.4668013301,2.2722457786));
#56412=CARTESIAN_POINT('Ctrl Pts',(-3.2362706081,-35.293523699,2.3402171845));
#56413=CARTESIAN_POINT('Ctrl Pts',(-3.21039981727,-35.3231016776,2.33049644021));
#56414=CARTESIAN_POINT('Ctrl Pts',(-3.18974009686,-35.3566452436,2.31893365909));
#56415=CARTESIAN_POINT('Ctrl Pts',(-3.17526480943,-35.3930381712,2.30588852441));
#56416=CARTESIAN_POINT('Ctrl Pts',(-3.16753533529,-35.4308584528,2.2918609559));
#56417=CARTESIAN_POINT('Ctrl Pts',(-3.16658333925,-35.4686787344,2.27738759286));
#56418=CARTESIAN_POINT('Ctrl Pts',(-3.24268782164,-35.2959076878,2.35939290014));
#56419=CARTESIAN_POINT('Ctrl Pts',(-3.21479367828,-35.3250197311,2.34761644611));
#56420=CARTESIAN_POINT('Ctrl Pts',(-3.19237820629,-35.3584237245,2.33347294503));
#56421=CARTESIAN_POINT('Ctrl Pts',(-3.17658501762,-35.3949324563,2.31744225071));
#56422=CARTESIAN_POINT('Ctrl Pts',(-3.16808413932,-35.4329970413,2.30020446638));
#56423=CARTESIAN_POINT('Ctrl Pts',(-3.16691857253,-35.4710616262,2.28248419619));
#56424=CARTESIAN_POINT('',(-3.21673309784852,-35.2978264918237,2.26193292933744));
#56425=CARTESIAN_POINT('Origin',(-3.46485248098951,-35.4651807159992,2.24112377406711));
#56426=CARTESIAN_POINT('Ctrl Pts',(-3.2167330984,-35.297826491,2.26193292922));
#56427=CARTESIAN_POINT('Ctrl Pts',(-3.22044227874,-35.2947170616,2.28115435818));
#56428=CARTESIAN_POINT('Ctrl Pts',(-3.22504500396,-35.2927962885,2.30073764763));
#56429=CARTESIAN_POINT('Ctrl Pts',(-3.23041275638,-35.292377214,2.32058136088));
#56430=CARTESIAN_POINT('Ctrl Pts',(-3.2362706081,-35.293523699,2.3402171845));
#56431=CARTESIAN_POINT('Ctrl Pts',(-3.24268782426,-35.2959076878,2.35939289968));
#56432=CARTESIAN_POINT('Ctrl Pts',(-3.05220590584922,-35.3446113342728,
0.449759468615835));
#56433=CARTESIAN_POINT('Ctrl Pts',(-3.04985791657899,-35.3562114182906,
0.449434297522738));
#56434=CARTESIAN_POINT('Ctrl Pts',(-3.04808113948102,-35.367925917271,0.449066823931494));
#56435=CARTESIAN_POINT('Ctrl Pts',(-3.04688319620433,-35.3797171894883,
0.44865810283722));
#56436=CARTESIAN_POINT('Ctrl Pts',(-3.04626798656282,-35.3915468489271,
0.448209464821468));
#56437=CARTESIAN_POINT('Ctrl Pts',(-3.0462356131786,-35.4033765082655,0.447722490273414));
#56438=CARTESIAN_POINT('Ctrl Pts',(-3.08188318868537,-35.3301475098315,
0.811344942556501));
#56439=CARTESIAN_POINT('Ctrl Pts',(-3.07718994972766,-35.3473935565693,
0.81096891066994));
#56440=CARTESIAN_POINT('Ctrl Pts',(-3.07363512368023,-35.3649271660184,
0.810506388572203));
#56441=CARTESIAN_POINT('Ctrl Pts',(-3.07124167037135,-35.3826542366648,
0.809959664856562));
#56442=CARTESIAN_POINT('Ctrl Pts',(-3.07002134535006,-35.4004780406225,
0.809331871876777));
#56443=CARTESIAN_POINT('Ctrl Pts',(-3.06997439732721,-35.4183018444796,
0.808626899063583));
#56444=CARTESIAN_POINT('Ctrl Pts',(-3.11480925207767,-35.3179426439912,
1.17419373715894));
#56445=CARTESIAN_POINT('Ctrl Pts',(-3.10654154250054,-35.3399109405316,
1.17393374594204));
#56446=CARTESIAN_POINT('Ctrl Pts',(-3.10026058630755,-35.3625419436199,
1.17351742209672));
#56447=CARTESIAN_POINT('Ctrl Pts',(-3.09603218734286,-35.3856208231373,
1.17294874807696));
#56448=CARTESIAN_POINT('Ctrl Pts',(-3.09389012681207,-35.4089236557388,
1.17223417157854));
#56449=CARTESIAN_POINT('Ctrl Pts',(-3.09383493395118,-35.4322264883404,
1.17138232965865));
#56450=CARTESIAN_POINT('Ctrl Pts',(-3.1489742418356,-35.3091111400076,1.53615855019239));
#56451=CARTESIAN_POINT('Ctrl Pts',(-3.13669434443428,-35.3344038135106,
1.53611929468437));
#56452=CARTESIAN_POINT('Ctrl Pts',(-3.12728783123044,-35.3610192894964,
1.53584317267495));
#56453=CARTESIAN_POINT('Ctrl Pts',(-3.12093413395616,-35.388538471225,1.53533340697713));
#56454=CARTESIAN_POINT('Ctrl Pts',(-3.11772590791843,-35.4165095347782,
1.5346003353224));
#56455=CARTESIAN_POINT('Ctrl Pts',(-3.11766406573072,-35.4444805983314,
1.53366030754776));
#56456=CARTESIAN_POINT('Ctrl Pts',(-3.18313684691208,-35.302468660032,1.89896579328351));
#56457=CARTESIAN_POINT('Ctrl Pts',(-3.1669425809763,-35.3302070617239,1.89920832725791));
#56458=CARTESIAN_POINT('Ctrl Pts',(-3.15441608130232,-35.3600495371066,
1.8991452966041));
#56459=CARTESIAN_POINT('Ctrl Pts',(-3.14591669935255,-35.3913550667249,
1.89877256662065));
#56460=CARTESIAN_POINT('Ctrl Pts',(-3.14163538349214,-35.4233924917858,
1.89809997064137));
#56461=CARTESIAN_POINT('Ctrl Pts',(-3.14157289101662,-35.4554299168467,
1.89714987809648));
#56462=CARTESIAN_POINT('Ctrl Pts',(-3.21697740925793,-35.2975133737574,
2.26232402686368));
#56463=CARTESIAN_POINT('Ctrl Pts',(-3.19706412796009,-35.32701786522,2.26284293679389));
#56464=CARTESIAN_POINT('Ctrl Pts',(-3.18151421558404,-35.3594737404149,
2.26299572724175));
#56465=CARTESIAN_POINT('Ctrl Pts',(-3.17091358409877,-35.3940160628362,
2.26276704500176));
#56466=CARTESIAN_POINT('Ctrl Pts',(-3.16558198118586,-35.4296028155102,
2.26216379089102));
#56467=CARTESIAN_POINT('Ctrl Pts',(-3.16551950497327,-35.4651895681841,
2.2612139556422));
#56468=CARTESIAN_POINT('',(-3.0522160941314,-35.3447053607003,0.450150554362896));
#56469=CARTESIAN_POINT('Origin',(-3.3455585084964,-35.4033872464943,0.428430041357342));
#56470=CARTESIAN_POINT('Ctrl Pts',(-3.0522160941314,-35.3447053607003,0.450150554362896));
#56471=CARTESIAN_POINT('Ctrl Pts',(-3.06245426700421,-35.3397367883934,
0.574985908505038));
#56472=CARTESIAN_POINT('Ctrl Pts',(-3.0731265985084,-35.3351675822744,0.699868808724409));
#56473=CARTESIAN_POINT('Ctrl Pts',(-3.0840963191387,-35.3309723772982,0.824833541278553));
#56474=CARTESIAN_POINT('Ctrl Pts',(-3.09693619197235,-35.3260619606868,
0.971102651382724));
#56475=CARTESIAN_POINT('Ctrl Pts',(-3.1101827780043,-35.3216639371358,1.11748237059042));
#56476=CARTESIAN_POINT('Ctrl Pts',(-3.12364374625223,-35.3177376313134,
1.26396179960472));
#56477=CARTESIAN_POINT('Ctrl Pts',(-3.13890997728794,-35.3132847650189,
1.43008571908232));
#56478=CARTESIAN_POINT('Ctrl Pts',(-3.15445073095059,-35.3094386256381,
1.59633247350827));
#56479=CARTESIAN_POINT('Ctrl Pts',(-3.17003379270651,-35.3061398799808,
1.762664238938));
#56480=CARTESIAN_POINT('Ctrl Pts',(-3.18219023638189,-35.3035665079176,
1.89242068664661));
#56481=CARTESIAN_POINT('Ctrl Pts',(-3.19437337743973,-35.3013262609218,
2.02222732843154));
#56482=CARTESIAN_POINT('Ctrl Pts',(-3.20649671361591,-35.2993909708028,
2.15209574766422));
#56483=CARTESIAN_POINT('Ctrl Pts',(-3.20991399946423,-35.2988454576338,
2.18870262754769));
#56484=CARTESIAN_POINT('Ctrl Pts',(-3.21332666694494,-35.298324174651,2.22531468874872));
#56485=CARTESIAN_POINT('Ctrl Pts',(-3.21673309838426,-35.2978264909894,
2.26193292922132));
#56486=CARTESIAN_POINT('Ctrl Pts',(-3.05109049587,-35.3458529008,0.437996404741));
#56487=CARTESIAN_POINT('Ctrl Pts',(-3.04891977816,-35.3572426278,0.438898953129));
#56488=CARTESIAN_POINT('Ctrl Pts',(-3.04730060509,-35.3687406938,0.439760831884));
#56489=CARTESIAN_POINT('Ctrl Pts',(-3.04623977506,-35.3803114393,0.440579215085));
#56490=CARTESIAN_POINT('Ctrl Pts',(-3.04574061974,-35.3919185251,0.441351532501));
#56491=CARTESIAN_POINT('Ctrl Pts',(-3.04580294181,-35.4035256109,0.442075517619));
#56492=CARTESIAN_POINT('Ctrl Pts',(-3.05133592857,-35.3454968218,0.440376332259));
#56493=CARTESIAN_POINT('Ctrl Pts',(-3.049131145,-35.3569269779,0.441037311376));
#56494=CARTESIAN_POINT('Ctrl Pts',(-3.04748040649,-35.368466371,0.44165738234));
#56495=CARTESIAN_POINT('Ctrl Pts',(-3.04639064899,-35.3800790478,0.442234462677));
#56496=CARTESIAN_POINT('Ctrl Pts',(-3.04586531061,-35.3917283673,0.442766727044));
#56497=CARTESIAN_POINT('Ctrl Pts',(-3.04590426722,-35.4033776868,0.443252644519));
#56498=CARTESIAN_POINT('Ctrl Pts',(-3.05157202469,-35.345201709,0.44278366337));
#56499=CARTESIAN_POINT('Ctrl Pts',(-3.04933300313,-35.3566718646,0.443200875235));
#56500=CARTESIAN_POINT('Ctrl Pts',(-3.04765109714,-35.3682522692,0.443576907233));
#56501=CARTESIAN_POINT('Ctrl Pts',(-3.04653338889,-35.3799066391,0.443910429375));
#56502=CARTESIAN_POINT('Ctrl Pts',(-3.04598342453,-35.3915979921,0.44420038209));
#56503=CARTESIAN_POINT('Ctrl Pts',(-3.0460011471,-35.4032893451,0.444445979659));
#56504=CARTESIAN_POINT('Ctrl Pts',(-3.05179796269,-35.3449700438,0.445216729023));
#56505=CARTESIAN_POINT('Ctrl Pts',(-3.04952458771,-35.3564797113,0.445388154931));
#56506=CARTESIAN_POINT('Ctrl Pts',(-3.04781198307,-35.3681007576,0.445518095267));
#56507=CARTESIAN_POINT('Ctrl Pts',(-3.04666739039,-35.3797965316,0.445605990135));
#56508=CARTESIAN_POINT('Ctrl Pts',(-3.04609446477,-35.3915296692,0.44565156091));
#56509=CARTESIAN_POINT('Ctrl Pts',(-3.04609320711,-35.4032628068,0.445654782512));
#56510=CARTESIAN_POINT('Ctrl Pts',(-3.05201291474,-35.344804036,0.447673318567));
#56511=CARTESIAN_POINT('Ctrl Pts',(-3.04970513582,-35.3563526648,0.447597170527));
#56512=CARTESIAN_POINT('Ctrl Pts',(-3.04796238182,-35.3680139256,0.447479196662));
#56513=CARTESIAN_POINT('Ctrl Pts',(-3.04679206061,-35.3797507581,0.447319633895));
#56514=CARTESIAN_POINT('Ctrl Pts',(-3.04619793931,-35.3915253768,0.447118989828));
#56515=CARTESIAN_POINT('Ctrl Pts',(-3.04618007217,-35.4032999955,0.446878030094));
#56516=CARTESIAN_POINT('Ctrl Pts',(-3.05221609529,-35.3447053607,0.45015055449));
#56517=CARTESIAN_POINT('Ctrl Pts',(-3.04987393679,-35.3562923356,0.449825338819));
#56518=CARTESIAN_POINT('Ctrl Pts',(-3.04810166196,-35.3679933207,0.449457922766));
#56519=CARTESIAN_POINT('Ctrl Pts',(-3.04690685539,-35.3797708063,0.449049358968));
#56520=CARTESIAN_POINT('Ctrl Pts',(-3.04629339744,-35.3915865426,0.448600974315));
#56521=CARTESIAN_POINT('Ctrl Pts',(-3.0462613893,-35.403402279,0.448114344323));
#56522=CARTESIAN_POINT('',(-3.05109044990346,-35.3458530848237,0.437996448767244));
#56523=CARTESIAN_POINT('Origin',(-3.34464260822978,-35.4035208271414,0.416342692624979));
#56524=CARTESIAN_POINT('Origin',(-3.03578495082005,-35.4311381890655,0.45269626373329));
#56525=CARTESIAN_POINT('Ctrl Pts',(-2.98571747284,-35.3277286717,0.261093980788));
#56526=CARTESIAN_POINT('Ctrl Pts',(-2.981461349,-35.3462477664,0.265774778659));
#56527=CARTESIAN_POINT('Ctrl Pts',(-2.97837661309,-35.3652776361,0.269499859243));
#56528=CARTESIAN_POINT('Ctrl Pts',(-2.97650103488,-35.3846541126,0.272227694446));
#56529=CARTESIAN_POINT('Ctrl Pts',(-2.97585138777,-35.4042039111,0.273933889101));
#56530=CARTESIAN_POINT('Ctrl Pts',(-2.9764225699,-35.4237537096,0.274612459172));
#56531=CARTESIAN_POINT('Ctrl Pts',(-2.99904170374,-35.3293548375,0.278294108299));
#56532=CARTESIAN_POINT('Ctrl Pts',(-2.99483616983,-35.347248816,0.282402750811));
#56533=CARTESIAN_POINT('Ctrl Pts',(-2.99178501636,-35.3655962934,0.285705549944));
#56534=CARTESIAN_POINT('Ctrl Pts',(-2.98992270743,-35.3842510435,0.288169202034));
#56535=CARTESIAN_POINT('Ctrl Pts',(-2.98926461676,-35.4030594457,0.289773532404));
#56536=CARTESIAN_POINT('Ctrl Pts',(-2.98980629628,-35.4218678479,0.290512461752));
#56537=CARTESIAN_POINT('Ctrl Pts',(-3.01081156168,-35.3311436809,0.296626108381));
#56538=CARTESIAN_POINT('Ctrl Pts',(-3.00676278967,-35.3483431627,0.300206793547));
#56539=CARTESIAN_POINT('Ctrl Pts',(-3.00382878865,-35.3659388616,0.303127857359));
#56540=CARTESIAN_POINT('Ctrl Pts',(-3.00203974789,-35.3838026166,0.305362985112));
#56541=CARTESIAN_POINT('Ctrl Pts',(-3.00140909733,-35.4018004061,0.306895543103));
#56542=CARTESIAN_POINT('Ctrl Pts',(-3.00193290967,-35.4197981956,0.307719289765));
#56543=CARTESIAN_POINT('Ctrl Pts',(-3.0211060441,-35.3328533463,0.316096062934));
#56544=CARTESIAN_POINT('Ctrl Pts',(-3.01723125611,-35.3493133446,0.319149425303));
#56545=CARTESIAN_POINT('Ctrl Pts',(-3.01441086074,-35.3661160441,0.321674359752));
#56546=CARTESIAN_POINT('Ctrl Pts',(-3.01267195982,-35.3831506732,0.32365017578));
#56547=CARTESIAN_POINT('Ctrl Pts',(-3.01202647228,-35.4003009737,0.325063889692));
#56548=CARTESIAN_POINT('Ctrl Pts',(-3.01247041893,-35.4174512741,0.325909903855));
#56549=CARTESIAN_POINT('Ctrl Pts',(-3.03608811322,-35.3362145716,0.351770920136));
#56550=CARTESIAN_POINT('Ctrl Pts',(-3.03261306094,-35.3513090757,0.353941667697));
#56551=CARTESIAN_POINT('Ctrl Pts',(-3.03006547046,-35.366660463,0.355785992804));
#56552=CARTESIAN_POINT('Ctrl Pts',(-3.02846382328,-35.3821846623,0.357292574606));
#56553=CARTESIAN_POINT('Ctrl Pts',(-3.02781696962,-35.3977954963,0.3584530028));
#56554=CARTESIAN_POINT('Ctrl Pts',(-3.02812402787,-35.4134063304,0.35926266557));
#56555=CARTESIAN_POINT('Ctrl Pts',(-3.04544130267,-35.3402488915,0.389133416749));
#56556=CARTESIAN_POINT('Ctrl Pts',(-3.04250648845,-35.3538042987,0.390631987385));
#56557=CARTESIAN_POINT('Ctrl Pts',(-3.040339577,-35.3675437775,0.391955910767));
#56558=CARTESIAN_POINT('Ctrl Pts',(-3.03895408512,-35.3814072732,0.393098415575));
#56559=CARTESIAN_POINT('Ctrl Pts',(-3.03835622743,-35.3953326096,0.394054612964));
#56560=CARTESIAN_POINT('Ctrl Pts',(-3.03854461847,-35.4092579459,0.394821151154));
#56561=CARTESIAN_POINT('Ctrl Pts',(-3.04837800292,-35.3421028535,0.405371326337));
#56562=CARTESIAN_POINT('Ctrl Pts',(-3.04569735965,-35.354968334,0.406623296912));
#56563=CARTESIAN_POINT('Ctrl Pts',(-3.04371425581,-35.367989887,0.407755259395));
#56564=CARTESIAN_POINT('Ctrl Pts',(-3.04243717253,-35.3811153925,0.408763338852));
#56565=CARTESIAN_POINT('Ctrl Pts',(-3.0418710033,-35.3942935555,0.40964296396));
#56566=CARTESIAN_POINT('Ctrl Pts',(-3.0420174994,-35.4074717185,0.410390857869));
#56567=CARTESIAN_POINT('Ctrl Pts',(-3.0502457294,-35.3440064303,0.421621283978));
#56568=CARTESIAN_POINT('Ctrl Pts',(-3.04782750294,-35.3561342576,0.422702630881));
#56569=CARTESIAN_POINT('Ctrl Pts',(-3.04603083038,-35.3683919899,0.423709393311));
#56570=CARTESIAN_POINT('Ctrl Pts',(-3.04486559316,-35.3807375362,0.424637122745));
#56571=CARTESIAN_POINT('Ctrl Pts',(-3.04433601307,-35.3931265369,0.425482937737));
#56572=CARTESIAN_POINT('Ctrl Pts',(-3.04444019246,-35.4055155376,0.426244325555));
#56573=CARTESIAN_POINT('Ctrl Pts',(-3.05109044578,-35.345853084,0.437996449073));
#56574=CARTESIAN_POINT('Ctrl Pts',(-3.04891974336,-35.357242792,0.438899021788));
#56575=CARTESIAN_POINT('Ctrl Pts',(-3.0473005821,-35.368740838,0.439760925705));
#56576=CARTESIAN_POINT('Ctrl Pts',(-3.04623976029,-35.380311563,0.440579334845));
#56577=CARTESIAN_POINT('Ctrl Pts',(-3.04574060956,-35.391918628,0.441351678913));
#56578=CARTESIAN_POINT('Ctrl Pts',(-3.04580293259,-35.4035256929,0.442075691324));
#56579=CARTESIAN_POINT('',(-2.98571747517108,-35.3277286769967,0.261093984850969));
#56580=CARTESIAN_POINT('Origin',(-3.20593730394412,-35.4237537994827,0.0814200323574604));
#56581=CARTESIAN_POINT('Ctrl Pts',(-2.98571747472,-35.3277286768,0.261093985219));
#56582=CARTESIAN_POINT('Ctrl Pts',(-2.99904170374,-35.3293548375,0.278294108299));
#56583=CARTESIAN_POINT('Ctrl Pts',(-3.01081156168,-35.3311436809,0.296626108381));
#56584=CARTESIAN_POINT('Ctrl Pts',(-3.0211060441,-35.3328533463,0.316096062934));
#56585=CARTESIAN_POINT('Ctrl Pts',(-3.03608811322,-35.3362145716,0.351770920136));
#56586=CARTESIAN_POINT('Ctrl Pts',(-3.04544130267,-35.3402488915,0.389133416749));
#56587=CARTESIAN_POINT('Ctrl Pts',(-3.04837800292,-35.3421028535,0.405371326337));
#56588=CARTESIAN_POINT('Ctrl Pts',(-3.0502457294,-35.3440064303,0.421621283978));
#56589=CARTESIAN_POINT('Ctrl Pts',(-3.05109044571,-35.345853084,0.437996449075));
#56590=CARTESIAN_POINT('Ctrl Pts',(-2.98281092022,-35.3272070934,0.257308726577));
#56591=CARTESIAN_POINT('Ctrl Pts',(-2.97803806995,-35.345862362,0.261512162033));
#56592=CARTESIAN_POINT('Ctrl Pts',(-2.97443750788,-35.3650398118,0.264729196731));
#56593=CARTESIAN_POINT('Ctrl Pts',(-2.97205219293,-35.3845716985,0.266921998871));
#56594=CARTESIAN_POINT('Ctrl Pts',(-2.97090376513,-35.4042808232,0.268070674403));
#56595=CARTESIAN_POINT('Ctrl Pts',(-2.97099139651,-35.4239899479,0.268174325124));
#56596=CARTESIAN_POINT('Ctrl Pts',(-2.98353703291,-35.3273786743,0.258262507142));
#56597=CARTESIAN_POINT('Ctrl Pts',(-2.97889447281,-35.3460005999,0.262582653758));
#56598=CARTESIAN_POINT('Ctrl Pts',(-2.97542363609,-35.3651416718,0.26592442057));
#56599=CARTESIAN_POINT('Ctrl Pts',(-2.97316614056,-35.3846350952,0.268249073819));
#56600=CARTESIAN_POINT('Ctrl Pts',(-2.97214238275,-35.4043047141,0.26953560217));
#56601=CARTESIAN_POINT('Ctrl Pts',(-2.97235045678,-35.4239743331,0.269781826657));
#56602=CARTESIAN_POINT('Ctrl Pts',(-2.98426364409,-35.3275231471,0.259211611404));
#56603=CARTESIAN_POINT('Ctrl Pts',(-2.97975071316,-35.3461112518,0.263650265626));
#56604=CARTESIAN_POINT('Ctrl Pts',(-2.97640915872,-35.3652155879,0.267118330752));
#56605=CARTESIAN_POINT('Ctrl Pts',(-2.97427928943,-35.3846702746,0.269576156755));
#56606=CARTESIAN_POINT('Ctrl Pts',(-2.97338027656,-35.4043001557,0.271001608633));
#56607=CARTESIAN_POINT('Ctrl Pts',(-2.97370914102,-35.4239300369,0.271391235523));
#56608=CARTESIAN_POINT('Ctrl Pts',(-2.98499053061,-35.3276399509,0.260155575417));
#56609=CARTESIAN_POINT('Ctrl Pts',(-2.98060644818,-35.3461937726,0.264714470388));
#56610=CARTESIAN_POINT('Ctrl Pts',(-2.97739362648,-35.3652610343,0.268310331454));
#56611=CARTESIAN_POINT('Ctrl Pts',(-2.97539109347,-35.3846767315,0.270902576923));
#56612=CARTESIAN_POINT('Ctrl Pts',(-2.9746168118,-35.404266665,0.272467944099));
#56613=CARTESIAN_POINT('Ctrl Pts',(-2.97506673688,-35.4238565985,0.27300171487));
#56614=CARTESIAN_POINT('Ctrl Pts',(-2.98571747678,-35.3277286766,0.26109398396));
#56615=CARTESIAN_POINT('Ctrl Pts',(-2.98146135285,-35.3462477712,0.26577478149));
#56616=CARTESIAN_POINT('Ctrl Pts',(-2.97837661705,-35.3652776408,0.269499861748));
#56617=CARTESIAN_POINT('Ctrl Pts',(-2.97650103844,-35.384654117,0.272227696729));
#56618=CARTESIAN_POINT('Ctrl Pts',(-2.97585139066,-35.4042039153,0.273933891593));
#56619=CARTESIAN_POINT('Ctrl Pts',(-2.97642257226,-35.4237537135,0.274612461819));
#56620=CARTESIAN_POINT('',(-2.98281092160732,-35.3272070855929,0.257308724107702));
#56621=CARTESIAN_POINT('Origin',(-3.20008735670538,-35.4239900447452,0.074485419786941));
#56622=CARTESIAN_POINT('Ctrl Pts',(-2.98281092022,-35.3272070934,0.257308726577));
#56623=CARTESIAN_POINT('Ctrl Pts',(-2.9837790702192,-35.3274358680927,0.258580433779342));
#56624=CARTESIAN_POINT('Ctrl Pts',(-2.98474821549444,-35.3276103756947,
0.259842772924741));
#56625=CARTESIAN_POINT('Ctrl Pts',(-2.98571747633655,-35.3277286775049,
0.261093983900082));
#56626=CARTESIAN_POINT('Ctrl Pts',(0.0562124907764,-35.2853263177,-1.2047009047));
#56627=CARTESIAN_POINT('Ctrl Pts',(0.0549190904069,-35.3188634055,-1.16900714311));
#56628=CARTESIAN_POINT('Ctrl Pts',(0.0535306616313,-35.3596876325,-1.14016366385));
#56629=CARTESIAN_POINT('Ctrl Pts',(0.0521190751148,-35.4059409749,-1.1201647488));
#56630=CARTESIAN_POINT('Ctrl Pts',(0.0507668332647,-35.454920083,-1.11017926619));
#56631=CARTESIAN_POINT('Ctrl Pts',(0.0495419561802,-35.503899191,-1.11019486262));
#56632=CARTESIAN_POINT('Ctrl Pts',(-0.201788256316,-35.2863590312,-1.20002331734));
#56633=CARTESIAN_POINT('Ctrl Pts',(-0.20059637751,-35.3196953033,-1.1671828612));
#56634=CARTESIAN_POINT('Ctrl Pts',(-0.199891058502,-35.3593803738,-1.14082521527));
#56635=CARTESIAN_POINT('Ctrl Pts',(-0.199745892902,-35.4037391848,-1.12259845523));
#56636=CARTESIAN_POINT('Ctrl Pts',(-0.200177402058,-35.4504424505,-1.11345401234));
#56637=CARTESIAN_POINT('Ctrl Pts',(-0.201137869134,-35.4971457162,-1.11338731493));
#56638=CARTESIAN_POINT('Ctrl Pts',(-0.458005640948,-35.2884465433,-1.1743412925));
#56639=CARTESIAN_POINT('Ctrl Pts',(-0.45532002803,-35.3213377511,-1.14466296307));
#56640=CARTESIAN_POINT('Ctrl Pts',(-0.4535812271,-35.3596601469,-1.12100512273));
#56641=CARTESIAN_POINT('Ctrl Pts',(-0.452922785697,-35.4019345515,-1.1046878387));
#56642=CARTESIAN_POINT('Ctrl Pts',(-0.453380153067,-35.4461899162,-1.09646210546));
#56643=CARTESIAN_POINT('Ctrl Pts',(-0.454881185093,-35.4904452809,-1.09632868214));
#56644=CARTESIAN_POINT('Ctrl Pts',(-0.713379137931,-35.2906784141,-1.12765964252));
#56645=CARTESIAN_POINT('Ctrl Pts',(-0.709079348273,-35.3228447776,-1.10136638154));
#56646=CARTESIAN_POINT('Ctrl Pts',(-0.70594831441,-35.3595655977,-1.08053117586));
#56647=CARTESIAN_POINT('Ctrl Pts',(-0.704166625027,-35.3995661124,-1.06618227068));
#56648=CARTESIAN_POINT('Ctrl Pts',(-0.703813714965,-35.4412096849,-1.05889834036));
#56649=CARTESIAN_POINT('Ctrl Pts',(-0.70484928931,-35.4828532574,-1.05868437313));
#56650=CARTESIAN_POINT('Ctrl Pts',(-1.38784510535,-35.2993373321,-0.947254707752));
#56651=CARTESIAN_POINT('Ctrl Pts',(-1.38135732447,-35.3286900482,-0.929878628182));
#56652=CARTESIAN_POINT('Ctrl Pts',(-1.37657158883,-35.3605166385,-0.91635466331));
#56653=CARTESIAN_POINT('Ctrl Pts',(-1.37367161422,-35.3940608782,-0.907077564055));
#56654=CARTESIAN_POINT('Ctrl Pts',(-1.37274039474,-35.4284641756,-0.90225909603));
#56655=CARTESIAN_POINT('Ctrl Pts',(-1.37374872204,-35.4628674729,-0.901908813904));
#56656=CARTESIAN_POINT('Ctrl Pts',(-2.01355395003,-35.311130732,-0.626706350821));
#56657=CARTESIAN_POINT('Ctrl Pts',(-2.00730643429,-35.336016544,-0.616608977986));
#56658=CARTESIAN_POINT('Ctrl Pts',(-2.00258568894,-35.3621198501,-0.608811606003));
#56659=CARTESIAN_POINT('Ctrl Pts',(-1.9994933297,-35.389055262,-0.603446176196));
#56660=CARTESIAN_POINT('Ctrl Pts',(-1.99808657075,-35.4164068328,-0.600583823803));
#56661=CARTESIAN_POINT('Ctrl Pts',(-1.99837189146,-35.4437584036,-0.600230058024));
#56662=CARTESIAN_POINT('Ctrl Pts',(-2.37717939564,-35.3191393972,-0.374243399004));
#56663=CARTESIAN_POINT('Ctrl Pts',(-2.37186878863,-35.3409656481,-0.367119757236));
#56664=CARTESIAN_POINT('Ctrl Pts',(-2.36789713578,-35.363631483,-0.361625053168));
#56665=CARTESIAN_POINT('Ctrl Pts',(-2.36532978406,-35.3868707128,-0.35784451611));
#56666=CARTESIAN_POINT('Ctrl Pts',(-2.36419887789,-35.4103967036,-0.355823775657));
#56667=CARTESIAN_POINT('Ctrl Pts',(-2.36450092427,-35.4339226943,-0.355565614957));
#56668=CARTESIAN_POINT('Ctrl Pts',(-2.70262665161,-35.324607016,-0.0770523694869));
#56669=CARTESIAN_POINT('Ctrl Pts',(-2.69780857299,-35.3442953406,-0.0717175970589));
#56670=CARTESIAN_POINT('Ctrl Pts',(-2.69419322648,-35.3646024007,-0.067613422701));
#56671=CARTESIAN_POINT('Ctrl Pts',(-2.69182933906,-35.3853302459,-0.0647926244646));
#56672=CARTESIAN_POINT('Ctrl Pts',(-2.69074110489,-35.4062685003,-0.0632832758083));
#56673=CARTESIAN_POINT('Ctrl Pts',(-2.69092668038,-35.4272067546,-0.063087197317));
#56674=CARTESIAN_POINT('Ctrl Pts',(-2.98281092266,-35.3272070795,0.257308721393));
#56675=CARTESIAN_POINT('Ctrl Pts',(-2.97803806023,-35.345862351,0.261512145638));
#56676=CARTESIAN_POINT('Ctrl Pts',(-2.97443748635,-35.3650398039,0.264729168335));
#56677=CARTESIAN_POINT('Ctrl Pts',(-2.97205215937,-35.3845716938,0.266921957853));
#56678=CARTESIAN_POINT('Ctrl Pts',(-2.97090371967,-35.4042808219,0.268070620572));
#56679=CARTESIAN_POINT('Ctrl Pts',(-2.97099133978,-35.4239899499,0.268174257926));
#56680=CARTESIAN_POINT('',(-9.45935213686968E-8,-35.2855840760402,-1.203282378976));
#56681=CARTESIAN_POINT('Ctrl Pts',(-9.45935213686968E-8,-35.2855840760402,
-1.203282378976));
#56682=CARTESIAN_POINT('Ctrl Pts',(-0.246462141036511,-35.2867310709528,
-1.19529915853671));
#56683=CARTESIAN_POINT('Ctrl Pts',(-0.491376340832031,-35.2887499565309,
-1.16811525832979));
#56684=CARTESIAN_POINT('Ctrl Pts',(-0.735140444018721,-35.2909646174122,
-1.121794106446));
#56685=CARTESIAN_POINT('Ctrl Pts',(-1.3979442783783,-35.2995330331731,-0.942077192818583));
#56686=CARTESIAN_POINT('Ctrl Pts',(-2.01355281302879,-35.3111352611287,
-0.626704513172324));
#56687=CARTESIAN_POINT('Ctrl Pts',(-2.37717842914973,-35.3191433694965,
-0.37424210255291));
#56688=CARTESIAN_POINT('Ctrl Pts',(-2.702625774756,-35.3246105992,-0.0770513985971862));
#56689=CARTESIAN_POINT('Ctrl Pts',(-2.98281092224,-35.3272070795,0.257308721649));
#56690=CARTESIAN_POINT('Origin',(1.43496042263357E-12,-35.5025674380817,
-1.41067474285734));
#56691=CARTESIAN_POINT('Ctrl Pts',(-0.0562124907764,-35.2853263177,-1.2047009047));
#56692=CARTESIAN_POINT('Ctrl Pts',(-0.0549190904069,-35.3188634055,-1.16900714311));
#56693=CARTESIAN_POINT('Ctrl Pts',(-0.0535306616313,-35.3596876325,-1.14016366385));
#56694=CARTESIAN_POINT('Ctrl Pts',(-0.0521190751148,-35.4059409749,-1.1201647488));
#56695=CARTESIAN_POINT('Ctrl Pts',(-0.0507668332647,-35.454920083,-1.11017926619));
#56696=CARTESIAN_POINT('Ctrl Pts',(-0.0495419561802,-35.503899191,-1.11019486262));
#56697=CARTESIAN_POINT('Ctrl Pts',(0.201788256316,-35.2863590312,-1.20002331734));
#56698=CARTESIAN_POINT('Ctrl Pts',(0.20059637751,-35.3196953033,-1.1671828612));
#56699=CARTESIAN_POINT('Ctrl Pts',(0.199891058502,-35.3593803738,-1.14082521527));
#56700=CARTESIAN_POINT('Ctrl Pts',(0.199745892902,-35.4037391848,-1.12259845523));
#56701=CARTESIAN_POINT('Ctrl Pts',(0.200177402058,-35.4504424505,-1.11345401234));
#56702=CARTESIAN_POINT('Ctrl Pts',(0.201137869134,-35.4971457162,-1.11338731493));
#56703=CARTESIAN_POINT('Ctrl Pts',(0.458005640948,-35.2884465433,-1.1743412925));
#56704=CARTESIAN_POINT('Ctrl Pts',(0.45532002803,-35.3213377511,-1.14466296307));
#56705=CARTESIAN_POINT('Ctrl Pts',(0.4535812271,-35.3596601469,-1.12100512273));
#56706=CARTESIAN_POINT('Ctrl Pts',(0.452922785697,-35.4019345515,-1.1046878387));
#56707=CARTESIAN_POINT('Ctrl Pts',(0.453380153067,-35.4461899162,-1.09646210546));
#56708=CARTESIAN_POINT('Ctrl Pts',(0.454881185093,-35.4904452809,-1.09632868214));
#56709=CARTESIAN_POINT('Ctrl Pts',(0.713379137931,-35.2906784141,-1.12765964252));
#56710=CARTESIAN_POINT('Ctrl Pts',(0.709079348273,-35.3228447776,-1.10136638154));
#56711=CARTESIAN_POINT('Ctrl Pts',(0.70594831441,-35.3595655977,-1.08053117586));
#56712=CARTESIAN_POINT('Ctrl Pts',(0.704166625027,-35.3995661124,-1.06618227068));
#56713=CARTESIAN_POINT('Ctrl Pts',(0.703813714965,-35.4412096849,-1.05889834036));
#56714=CARTESIAN_POINT('Ctrl Pts',(0.70484928931,-35.4828532574,-1.05868437313));
#56715=CARTESIAN_POINT('Ctrl Pts',(1.38784510535,-35.2993373321,-0.947254707752));
#56716=CARTESIAN_POINT('Ctrl Pts',(1.38135732447,-35.3286900482,-0.929878628182));
#56717=CARTESIAN_POINT('Ctrl Pts',(1.37657158883,-35.3605166385,-0.91635466331));
#56718=CARTESIAN_POINT('Ctrl Pts',(1.37367161422,-35.3940608782,-0.907077564055));
#56719=CARTESIAN_POINT('Ctrl Pts',(1.37274039474,-35.4284641756,-0.90225909603));
#56720=CARTESIAN_POINT('Ctrl Pts',(1.37374872204,-35.4628674729,-0.901908813904));
#56721=CARTESIAN_POINT('Ctrl Pts',(2.01355395003,-35.311130732,-0.626706350821));
#56722=CARTESIAN_POINT('Ctrl Pts',(2.00730643429,-35.336016544,-0.616608977986));
#56723=CARTESIAN_POINT('Ctrl Pts',(2.00258568894,-35.3621198501,-0.608811606003));
#56724=CARTESIAN_POINT('Ctrl Pts',(1.9994933297,-35.389055262,-0.603446176196));
#56725=CARTESIAN_POINT('Ctrl Pts',(1.99808657075,-35.4164068328,-0.600583823803));
#56726=CARTESIAN_POINT('Ctrl Pts',(1.99837189146,-35.4437584036,-0.600230058024));
#56727=CARTESIAN_POINT('Ctrl Pts',(2.37717939564,-35.3191393972,-0.374243399004));
#56728=CARTESIAN_POINT('Ctrl Pts',(2.37186878863,-35.3409656481,-0.367119757236));
#56729=CARTESIAN_POINT('Ctrl Pts',(2.36789713578,-35.363631483,-0.361625053168));
#56730=CARTESIAN_POINT('Ctrl Pts',(2.36532978406,-35.3868707128,-0.35784451611));
#56731=CARTESIAN_POINT('Ctrl Pts',(2.36419887789,-35.4103967036,-0.355823775657));
#56732=CARTESIAN_POINT('Ctrl Pts',(2.36450092427,-35.4339226943,-0.355565614957));
#56733=CARTESIAN_POINT('Ctrl Pts',(2.70262665161,-35.324607016,-0.0770523694869));
#56734=CARTESIAN_POINT('Ctrl Pts',(2.69780857299,-35.3442953406,-0.0717175970589));
#56735=CARTESIAN_POINT('Ctrl Pts',(2.69419322648,-35.3646024007,-0.067613422701));
#56736=CARTESIAN_POINT('Ctrl Pts',(2.69182933906,-35.3853302459,-0.0647926244646));
#56737=CARTESIAN_POINT('Ctrl Pts',(2.69074110489,-35.4062685003,-0.0632832758083));
#56738=CARTESIAN_POINT('Ctrl Pts',(2.69092668038,-35.4272067546,-0.063087197317));
#56739=CARTESIAN_POINT('Ctrl Pts',(2.98281092266,-35.3272070795,0.257308721393));
#56740=CARTESIAN_POINT('Ctrl Pts',(2.97803806023,-35.345862351,0.261512145638));
#56741=CARTESIAN_POINT('Ctrl Pts',(2.97443748635,-35.3650398039,0.264729168335));
#56742=CARTESIAN_POINT('Ctrl Pts',(2.97205215937,-35.3845716938,0.266921957853));
#56743=CARTESIAN_POINT('Ctrl Pts',(2.97090371967,-35.4042808219,0.268070620572));
#56744=CARTESIAN_POINT('Ctrl Pts',(2.97099133978,-35.4239899499,0.268174257926));
#56745=CARTESIAN_POINT('',(2.98281092138865,-35.3272070856442,0.257308723513503));
#56746=CARTESIAN_POINT('Origin',(3.20008730232451,-35.423990048778,0.074485335177551));
#56747=CARTESIAN_POINT('Ctrl Pts',(-9.45222527193312E-8,-35.285576877971,
-1.20327550011348));
#56748=CARTESIAN_POINT('Ctrl Pts',(0.0614972181873807,-35.2858729988589,
-1.20127673805126));
#56749=CARTESIAN_POINT('Ctrl Pts',(0.12475096035803,-35.2862554013519,-1.19776918615153));
#56750=CARTESIAN_POINT('Ctrl Pts',(0.189714992976335,-35.286710572023,-1.19250029860945));
#56751=CARTESIAN_POINT('Ctrl Pts',(0.253080303565567,-35.2871545412439,
-1.18736107491739));
#56752=CARTESIAN_POINT('Ctrl Pts',(0.318073164574926,-35.2876676839599,
-1.18054592797751));
#56753=CARTESIAN_POINT('Ctrl Pts',(0.384603016748727,-35.2882448843954,
-1.17181797651484));
#56754=CARTESIAN_POINT('Ctrl Pts',(0.453001767346575,-35.2888382990407,
-1.16284484707266));
#56755=CARTESIAN_POINT('Ctrl Pts',(0.523025330275769,-35.2894995032065,
-1.15184974180236));
#56756=CARTESIAN_POINT('Ctrl Pts',(0.59451821079149,-35.2902309277385,-1.13857562603336));
#56757=CARTESIAN_POINT('Ctrl Pts',(0.651801537075522,-35.290816978123,-1.12793980468663));
#56758=CARTESIAN_POINT('Ctrl Pts',(0.710026730424283,-35.2914483971486,
-1.11584085180069));
#56759=CARTESIAN_POINT('Ctrl Pts',(0.769089812910904,-35.2921284387114,
-1.10214793193385));
#56760=CARTESIAN_POINT('Ctrl Pts',(0.859844617649464,-35.2931733729857,
-1.08110774546716));
#56761=CARTESIAN_POINT('Ctrl Pts',(0.952636103171223,-35.2943240410569,
-1.05629997486956));
#56762=CARTESIAN_POINT('Ctrl Pts',(1.04705097486316,-35.2955911403668,-1.02723022917726));
#56763=CARTESIAN_POINT('Ctrl Pts',(1.09723468979318,-35.2962646333179,-1.01177897870402));
#56764=CARTESIAN_POINT('Ctrl Pts',(1.14787610914596,-35.2969706853886,-0.995123811975983));
#56765=CARTESIAN_POINT('Ctrl Pts',(1.19891695691765,-35.2977048215787,-0.977191637208916));
#56766=CARTESIAN_POINT('Ctrl Pts',(1.20129469642974,-35.2977390213364,-0.976356266278715));
#56767=CARTESIAN_POINT('Ctrl Pts',(1.20367328632146,-35.2977732882489,-0.975518124932157));
#56768=CARTESIAN_POINT('Ctrl Pts',(1.20605272170261,-35.2978076216918,-0.974677205666163));
#56769=CARTESIAN_POINT('Ctrl Pts',(1.27725989092447,-35.2988350869861,-0.949511789975523));
#56770=CARTESIAN_POINT('Ctrl Pts',(1.34922652726592,-35.2999228250693,-0.921858000564636));
#56771=CARTESIAN_POINT('Ctrl Pts',(1.42174183512206,-35.3010717162344,-0.891524167229231));
#56772=CARTESIAN_POINT('Ctrl Pts',(1.4592110629062,-35.3016653573019,-0.875850437855217));
#56773=CARTESIAN_POINT('Ctrl Pts',(1.49682629106069,-35.3022752902411,-0.859461217061494));
#56774=CARTESIAN_POINT('Ctrl Pts',(1.53455512107422,-35.3029014543288,-0.842330615007104));
#56775=CARTESIAN_POINT('Ctrl Pts',(1.55341953608098,-35.3032145363727,-0.833765313979908));
#56776=CARTESIAN_POINT('Ctrl Pts',(1.57231234894133,-35.3035316723579,-0.825014661717318));
#56777=CARTESIAN_POINT('Ctrl Pts',(1.59122924975292,-35.3038528498659,-0.816075491944981));
#56778=CARTESIAN_POINT('Ctrl Pts',(1.60068770015871,-35.3040134386198,-0.811605907058813));
#56779=CARTESIAN_POINT('Ctrl Pts',(1.61015217242701,-35.3041750376006,-0.807089192543942));
#56780=CARTESIAN_POINT('Ctrl Pts',(1.61962211971477,-35.304337644519,-0.802524954373084));
#56781=CARTESIAN_POINT('Ctrl Pts',(1.62435709335865,-35.3044189479782,-0.800242835287656));
#56782=CARTESIAN_POINT('Ctrl Pts',(1.62909343574822,-35.3045005034126,-0.797948835272099));
#56783=CARTESIAN_POINT('Ctrl Pts',(1.63383107763051,-35.3045823105274,-0.795642905349689));
#56784=CARTESIAN_POINT('Ctrl Pts',(1.63619989857166,-35.3046232140848,-0.794489940388483));
#56785=CARTESIAN_POINT('Ctrl Pts',(1.63856904438543,-35.3046641805619,-0.793333992949638));
#56786=CARTESIAN_POINT('Ctrl Pts',(1.64093850635605,-35.3047052099212,-0.792175056930587));
#56787=CARTESIAN_POINT('Ctrl Pts',(1.64330796832666,-35.3047462392806,-0.791016120911536));
#56788=CARTESIAN_POINT('Ctrl Pts',(1.6443966453675,-35.3047650866673,-0.79048386835501));
#56789=CARTESIAN_POINT('Ctrl Pts',(1.6480476607185,-35.3048292587342,-0.788688863658591));
#56790=CARTESIAN_POINT('Ctrl Pts',(1.70123429550726,-35.3057640935558,-0.762539902327496));
#56791=CARTESIAN_POINT('Ctrl Pts',(1.75111821236543,-35.3066639064797,-0.736590388689801));
#56792=CARTESIAN_POINT('Ctrl Pts',(1.79782737592309,-35.3075185789543,-0.711197975455024));
#56793=CARTESIAN_POINT('Ctrl Pts',(1.84589424537922,-35.3083980943884,-0.685067475159823));
#56794=CARTESIAN_POINT('Ctrl Pts',(1.89059973686305,-35.3092298180379,-0.659526935062845));
#56795=CARTESIAN_POINT('Ctrl Pts',(1.93209089082562,-35.3100071852016,-0.634911745427993));
#56796=CARTESIAN_POINT('Ctrl Pts',(1.97408375056434,-35.3107939521907,-0.609998912039198));
#56797=CARTESIAN_POINT('Ctrl Pts',(2.0127846495597,-35.3115250983264,-0.586033789444093));
#56798=CARTESIAN_POINT('Ctrl Pts',(2.04834444134429,-35.3121977596016,-0.563310572130525));
#56799=CARTESIAN_POINT('Ctrl Pts',(2.0843157894759,-35.3128782060185,-0.54032436440446));
#56800=CARTESIAN_POINT('Ctrl Pts',(2.11707341328875,-35.3134988804558,-0.518608822018224));
#56801=CARTESIAN_POINT('Ctrl Pts',(2.14676353560029,-35.3140598031597,-0.498416392096874));
#56802=CARTESIAN_POINT('Ctrl Pts',(2.1543486405602,-35.3142031052836,-0.49325771680608));
#56803=CARTESIAN_POINT('Ctrl Pts',(2.16173346496828,-35.3143425193064,-0.488198196245356));
#56804=CARTESIAN_POINT('Ctrl Pts',(2.16892028603487,-35.3144780671423,-0.483241521533293));
#56805=CARTESIAN_POINT('Ctrl Pts',(2.19778835526041,-35.315022536564,-0.463331518572251));
#56806=CARTESIAN_POINT('Ctrl Pts',(2.22346417948716,-35.315504554706,-0.445084466403678));
#56807=CARTESIAN_POINT('Ctrl Pts',(2.24608377138598,-35.3159269723923,-0.428705133107888));
#56808=CARTESIAN_POINT('Ctrl Pts',(2.26830884505752,-35.3163420225063,-0.412611478950989));
#56809=CARTESIAN_POINT('Ctrl Pts',(2.28758359799759,-35.3166995980441,-0.398320624291156));
#56810=CARTESIAN_POINT('Ctrl Pts',(2.30401276785091,-35.3170028614933,-0.385979989195755));
#56811=CARTESIAN_POINT('Ctrl Pts',(2.32087939004264,-35.317314199806,-0.373310765393305));
#56812=CARTESIAN_POINT('Ctrl Pts',(2.33474734337766,-35.3175683488764,-0.362696973253167));
#56813=CARTESIAN_POINT('Ctrl Pts',(2.34570019490273,-35.3177683471626,-0.354249400480844));
#56814=CARTESIAN_POINT('Ctrl Pts',(2.35117662066526,-35.3178683463057,-0.350025614094683));
#56815=CARTESIAN_POINT('Ctrl Pts',(2.35592376016089,-35.3179547964115,-0.346342639570059));
#56816=CARTESIAN_POINT('Ctrl Pts',(2.3599489400905,-35.3180279872108,-0.34320990432561));
#56817=CARTESIAN_POINT('Ctrl Pts',(2.3619615300553,-35.3180645826105,-0.341643536703386));
#56818=CARTESIAN_POINT('Ctrl Pts',(2.36379359571024,-35.3180978620434,-0.340214684300089));
#56819=CARTESIAN_POINT('Ctrl Pts',(2.36544584989918,-35.318127854485,-0.338924255123493));
#56820=CARTESIAN_POINT('Ctrl Pts',(2.36638037096635,-35.3181448183206,-0.338194383618681));
#56821=CARTESIAN_POINT('Ctrl Pts',(2.3672573665503,-35.3181607305319,-0.337508791467333));
#56822=CARTESIAN_POINT('Ctrl Pts',(2.36807694618827,-35.3181755956209,-0.336867617636297));
#56823=CARTESIAN_POINT('Ctrl Pts',(2.36866408946375,-35.3181862449057,-0.336408283502235));
#56824=CARTESIAN_POINT('Ctrl Pts',(2.36922497418766,-35.3181964149313,-0.335969231388025));
#56825=CARTESIAN_POINT('Ctrl Pts',(2.36974609787095,-35.3182058617932,-0.335561112266989));
#56826=CARTESIAN_POINT('Ctrl Pts',(2.36978365244749,-35.3182065425777,-0.335531701320494));
#56827=CARTESIAN_POINT('Ctrl Pts',(2.36982098686393,-35.3182072193589,-0.335502461737859));
#56828=CARTESIAN_POINT('Ctrl Pts',(2.36985809230613,-35.3182078919776,-0.335473400459684));
#56829=CARTESIAN_POINT('Ctrl Pts',(2.3701780251888,-35.3182136914725,-0.335222826475173));
#56830=CARTESIAN_POINT('Ctrl Pts',(2.37049274317138,-35.318219406958,-0.334977240828002));
#56831=CARTESIAN_POINT('Ctrl Pts',(2.37249838105661,-35.3182557329203,-0.333403765987897));
#56832=CARTESIAN_POINT('Ctrl Pts',(2.436709599302,-35.3194187216703,-0.283028403064282));
#56833=CARTESIAN_POINT('Ctrl Pts',(2.49734850532433,-35.3204801616452,-0.232367280315841));
#56834=CARTESIAN_POINT('Ctrl Pts',(2.55458115188229,-35.3214330129731,-0.181871002070266));
#56835=CARTESIAN_POINT('Ctrl Pts',(2.61305107463453,-35.3224064633879,-0.130283076893613));
#56836=CARTESIAN_POINT('Ctrl Pts',(2.66796645352324,-35.3232666833824,-0.0788672652294133));
#56837=CARTESIAN_POINT('Ctrl Pts',(2.71953139329132,-35.3240162990872,-0.0280559043515061));
#56838=CARTESIAN_POINT('Ctrl Pts',(2.77276235772848,-35.3247901343153,0.0243971336246918));
#56839=CARTESIAN_POINT('Ctrl Pts',(2.82242345816926,-35.3254462594998,0.0762059115642822));
#56840=CARTESIAN_POINT('Ctrl Pts',(2.86875884666911,-35.3259962351236,0.12694712440495));
#56841=CARTESIAN_POINT('Ctrl Pts',(2.90926007567917,-35.3264769624771,0.171299433688266));
#56842=CARTESIAN_POINT('Ctrl Pts',(2.94722090693888,-35.326876810181,0.214836970860647));
#56843=CARTESIAN_POINT('Ctrl Pts',(2.9828109225733,-35.3272070796485,0.257308721368552));
#56844=CARTESIAN_POINT('Ctrl Pts',(2.98281092022,-35.3272070934,0.257308726577));
#56845=CARTESIAN_POINT('Ctrl Pts',(2.97803806995,-35.345862362,0.261512162033));
#56846=CARTESIAN_POINT('Ctrl Pts',(2.97443750788,-35.3650398118,0.264729196731));
#56847=CARTESIAN_POINT('Ctrl Pts',(2.97205219293,-35.3845716985,0.266921998871));
#56848=CARTESIAN_POINT('Ctrl Pts',(2.97090376513,-35.4042808232,0.268070674403));
#56849=CARTESIAN_POINT('Ctrl Pts',(2.97099139651,-35.4239899479,0.268174325124));
#56850=CARTESIAN_POINT('Ctrl Pts',(2.98353703291,-35.3273786743,0.258262507142));
#56851=CARTESIAN_POINT('Ctrl Pts',(2.97889447281,-35.3460005999,0.262582653758));
#56852=CARTESIAN_POINT('Ctrl Pts',(2.97542363609,-35.3651416718,0.26592442057));
#56853=CARTESIAN_POINT('Ctrl Pts',(2.97316614056,-35.3846350952,0.268249073819));
#56854=CARTESIAN_POINT('Ctrl Pts',(2.97214238275,-35.4043047141,0.26953560217));
#56855=CARTESIAN_POINT('Ctrl Pts',(2.97235045678,-35.4239743331,0.269781826657));
#56856=CARTESIAN_POINT('Ctrl Pts',(2.98426364409,-35.3275231471,0.259211611404));
#56857=CARTESIAN_POINT('Ctrl Pts',(2.97975071316,-35.3461112518,0.263650265626));
#56858=CARTESIAN_POINT('Ctrl Pts',(2.97640915872,-35.3652155879,0.267118330752));
#56859=CARTESIAN_POINT('Ctrl Pts',(2.97427928943,-35.3846702746,0.269576156755));
#56860=CARTESIAN_POINT('Ctrl Pts',(2.97338027656,-35.4043001557,0.271001608633));
#56861=CARTESIAN_POINT('Ctrl Pts',(2.97370914102,-35.4239300369,0.271391235523));
#56862=CARTESIAN_POINT('Ctrl Pts',(2.98499053061,-35.3276399509,0.260155575417));
#56863=CARTESIAN_POINT('Ctrl Pts',(2.98060644818,-35.3461937726,0.264714470388));
#56864=CARTESIAN_POINT('Ctrl Pts',(2.97739362648,-35.3652610343,0.268310331454));
#56865=CARTESIAN_POINT('Ctrl Pts',(2.97539109347,-35.3846767315,0.270902576923));
#56866=CARTESIAN_POINT('Ctrl Pts',(2.9746168118,-35.404266665,0.272467944099));
#56867=CARTESIAN_POINT('Ctrl Pts',(2.97506673688,-35.4238565985,0.27300171487));
#56868=CARTESIAN_POINT('Ctrl Pts',(2.98571747678,-35.3277286766,0.26109398396));
#56869=CARTESIAN_POINT('Ctrl Pts',(2.98146135285,-35.3462477712,0.26577478149));
#56870=CARTESIAN_POINT('Ctrl Pts',(2.97837661705,-35.3652776408,0.269499861748));
#56871=CARTESIAN_POINT('Ctrl Pts',(2.97650103844,-35.384654117,0.272227696729));
#56872=CARTESIAN_POINT('Ctrl Pts',(2.97585139066,-35.4042039153,0.273933891593));
#56873=CARTESIAN_POINT('Ctrl Pts',(2.97642257226,-35.4237537135,0.274612461819));
#56874=CARTESIAN_POINT('',(2.98571747516532,-35.3277286769942,0.261093984855667));
#56875=CARTESIAN_POINT('Origin',(3.20593733485692,-35.4237538137774,0.0814200066647186));
#56876=CARTESIAN_POINT('Ctrl Pts',(2.98281092022,-35.3272070934,0.257308726577));
#56877=CARTESIAN_POINT('Ctrl Pts',(2.9837790702192,-35.3274358680927,0.258580433779342));
#56878=CARTESIAN_POINT('Ctrl Pts',(2.98474821549444,-35.3276103756947,0.259842772924741));
#56879=CARTESIAN_POINT('Ctrl Pts',(2.98571747633655,-35.3277286775049,0.261093983900082));
#56880=CARTESIAN_POINT('Ctrl Pts',(2.98571747284,-35.3277286717,0.261093980788));
#56881=CARTESIAN_POINT('Ctrl Pts',(2.981461349,-35.3462477664,0.265774778659));
#56882=CARTESIAN_POINT('Ctrl Pts',(2.97837661309,-35.3652776361,0.269499859243));
#56883=CARTESIAN_POINT('Ctrl Pts',(2.97650103488,-35.3846541126,0.272227694446));
#56884=CARTESIAN_POINT('Ctrl Pts',(2.97585138777,-35.4042039111,0.273933889101));
#56885=CARTESIAN_POINT('Ctrl Pts',(2.9764225699,-35.4237537096,0.274612459172));
#56886=CARTESIAN_POINT('Ctrl Pts',(2.99904170374,-35.3293548375,0.278294108299));
#56887=CARTESIAN_POINT('Ctrl Pts',(2.99483616983,-35.347248816,0.282402750811));
#56888=CARTESIAN_POINT('Ctrl Pts',(2.99178501636,-35.3655962934,0.285705549944));
#56889=CARTESIAN_POINT('Ctrl Pts',(2.98992270743,-35.3842510435,0.288169202034));
#56890=CARTESIAN_POINT('Ctrl Pts',(2.98926461676,-35.4030594457,0.289773532404));
#56891=CARTESIAN_POINT('Ctrl Pts',(2.98980629628,-35.4218678479,0.290512461752));
#56892=CARTESIAN_POINT('Ctrl Pts',(3.01081156168,-35.3311436809,0.296626108381));
#56893=CARTESIAN_POINT('Ctrl Pts',(3.00676278967,-35.3483431627,0.300206793547));
#56894=CARTESIAN_POINT('Ctrl Pts',(3.00382878865,-35.3659388616,0.303127857359));
#56895=CARTESIAN_POINT('Ctrl Pts',(3.00203974789,-35.3838026166,0.305362985112));
#56896=CARTESIAN_POINT('Ctrl Pts',(3.00140909733,-35.4018004061,0.306895543103));
#56897=CARTESIAN_POINT('Ctrl Pts',(3.00193290967,-35.4197981956,0.307719289765));
#56898=CARTESIAN_POINT('Ctrl Pts',(3.0211060441,-35.3328533463,0.316096062934));
#56899=CARTESIAN_POINT('Ctrl Pts',(3.01723125611,-35.3493133446,0.319149425303));
#56900=CARTESIAN_POINT('Ctrl Pts',(3.01441086074,-35.3661160441,0.321674359752));
#56901=CARTESIAN_POINT('Ctrl Pts',(3.01267195982,-35.3831506732,0.32365017578));
#56902=CARTESIAN_POINT('Ctrl Pts',(3.01202647228,-35.4003009737,0.325063889693));
#56903=CARTESIAN_POINT('Ctrl Pts',(3.01247041893,-35.4174512741,0.325909903855));
#56904=CARTESIAN_POINT('Ctrl Pts',(3.03608811322,-35.3362145716,0.351770920136));
#56905=CARTESIAN_POINT('Ctrl Pts',(3.03261306094,-35.3513090757,0.353941667697));
#56906=CARTESIAN_POINT('Ctrl Pts',(3.03006547046,-35.366660463,0.355785992804));
#56907=CARTESIAN_POINT('Ctrl Pts',(3.02846382328,-35.3821846623,0.357292574606));
#56908=CARTESIAN_POINT('Ctrl Pts',(3.02781696962,-35.3977954963,0.3584530028));
#56909=CARTESIAN_POINT('Ctrl Pts',(3.02812402787,-35.4134063304,0.35926266557));
#56910=CARTESIAN_POINT('Ctrl Pts',(3.04544130267,-35.3402488915,0.389133416749));
#56911=CARTESIAN_POINT('Ctrl Pts',(3.04250648845,-35.3538042987,0.390631987385));
#56912=CARTESIAN_POINT('Ctrl Pts',(3.040339577,-35.3675437775,0.391955910767));
#56913=CARTESIAN_POINT('Ctrl Pts',(3.03895408512,-35.3814072732,0.393098415575));
#56914=CARTESIAN_POINT('Ctrl Pts',(3.03835622743,-35.3953326096,0.394054612964));
#56915=CARTESIAN_POINT('Ctrl Pts',(3.03854461847,-35.4092579459,0.394821151154));
#56916=CARTESIAN_POINT('Ctrl Pts',(3.04837800292,-35.3421028535,0.405371326337));
#56917=CARTESIAN_POINT('Ctrl Pts',(3.04569735965,-35.354968334,0.406623296912));
#56918=CARTESIAN_POINT('Ctrl Pts',(3.04371425581,-35.367989887,0.407755259395));
#56919=CARTESIAN_POINT('Ctrl Pts',(3.04243717253,-35.3811153925,0.408763338852));
#56920=CARTESIAN_POINT('Ctrl Pts',(3.0418710033,-35.3942935555,0.40964296396));
#56921=CARTESIAN_POINT('Ctrl Pts',(3.0420174994,-35.4074717185,0.410390857869));
#56922=CARTESIAN_POINT('Ctrl Pts',(3.0502457294,-35.3440064303,0.421621283978));
#56923=CARTESIAN_POINT('Ctrl Pts',(3.04782750294,-35.3561342576,0.422702630881));
#56924=CARTESIAN_POINT('Ctrl Pts',(3.04603083038,-35.3683919899,0.423709393311));
#56925=CARTESIAN_POINT('Ctrl Pts',(3.04486559316,-35.3807375362,0.424637122745));
#56926=CARTESIAN_POINT('Ctrl Pts',(3.04433601307,-35.3931265369,0.425482937737));
#56927=CARTESIAN_POINT('Ctrl Pts',(3.04444019246,-35.4055155376,0.426244325555));
#56928=CARTESIAN_POINT('Ctrl Pts',(3.05109044578,-35.345853084,0.437996449073));
#56929=CARTESIAN_POINT('Ctrl Pts',(3.04891974336,-35.357242792,0.438899021788));
#56930=CARTESIAN_POINT('Ctrl Pts',(3.0473005821,-35.368740838,0.439760925705));
#56931=CARTESIAN_POINT('Ctrl Pts',(3.04623976029,-35.380311563,0.440579334845));
#56932=CARTESIAN_POINT('Ctrl Pts',(3.04574060956,-35.391918628,0.441351678913));
#56933=CARTESIAN_POINT('Ctrl Pts',(3.04580293259,-35.4035256929,0.442075691324));
#56934=CARTESIAN_POINT('',(3.05109044990354,-35.3458530848239,0.437996448765818));
#56935=CARTESIAN_POINT('Origin',(3.34464449040265,-35.4035194920317,0.416364015877388));
#56936=CARTESIAN_POINT('Ctrl Pts',(2.9857174744567,-35.3277286766852,0.261093985433823));
#56937=CARTESIAN_POINT('Ctrl Pts',(2.99164509856773,-35.3284521172012,0.268745900785589));
#56938=CARTESIAN_POINT('Ctrl Pts',(2.99729005843478,-35.3292209076218,0.276777206877757));
#56939=CARTESIAN_POINT('Ctrl Pts',(3.00261892051309,-35.3300138265231,0.285196864882465));
#56940=CARTESIAN_POINT('Ctrl Pts',(3.00830106634229,-35.3308593130007,0.294174714920944));
#56941=CARTESIAN_POINT('Ctrl Pts',(3.01362328701173,-35.3317331213617,0.303594619723798));
#56942=CARTESIAN_POINT('Ctrl Pts',(3.01851367686819,-35.3326519248837,0.313432781673084));
#56943=CARTESIAN_POINT('Ctrl Pts',(3.02375368720857,-35.3336364148931,0.323974286922699));
#56944=CARTESIAN_POINT('Ctrl Pts',(3.02849607780734,-35.3346755074925,0.334996514888742));
#56945=CARTESIAN_POINT('Ctrl Pts',(3.03263528909564,-35.3358079210548,0.346423067558966));
#56946=CARTESIAN_POINT('Ctrl Pts',(3.03394300126408,-35.3361656875209,0.350033089113673));
#56947=CARTESIAN_POINT('Ctrl Pts',(3.03519051631512,-35.3365326913694,0.353683104974461));
#56948=CARTESIAN_POINT('Ctrl Pts',(3.0363747716968,-35.3369095627627,0.357369717393274));
#56949=CARTESIAN_POINT('Ctrl Pts',(3.03988840496031,-35.3380277234941,0.368307733149693));
#56950=CARTESIAN_POINT('Ctrl Pts',(3.04284311652455,-35.3392359571205,0.379569460963959));
#56951=CARTESIAN_POINT('Ctrl Pts',(3.04517508581328,-35.3405165043927,0.391069582657007));
#56952=CARTESIAN_POINT('Ctrl Pts',(3.04698057772651,-35.3415079487294,0.399973377753454));
#56953=CARTESIAN_POINT('Ctrl Pts',(3.04841326094402,-35.3425418417111,0.409017474653859));
#56954=CARTESIAN_POINT('Ctrl Pts',(3.04945570098349,-35.3435920710794,0.418177350402306));
#56955=CARTESIAN_POINT('Ctrl Pts',(3.05020053253474,-35.344342468167,0.424722153177225));
#56956=CARTESIAN_POINT('Ctrl Pts',(3.05074635985724,-35.3451008715098,0.43132620995016));
#56957=CARTESIAN_POINT('Ctrl Pts',(3.05109044577719,-35.3458530840132,0.437996449070046));
#56958=CARTESIAN_POINT('Ctrl Pts',(3.05109049587,-35.3458529008,0.437996404741));
#56959=CARTESIAN_POINT('Ctrl Pts',(3.04891977816,-35.3572426278,0.438898953129));
#56960=CARTESIAN_POINT('Ctrl Pts',(3.04730060509,-35.3687406938,0.439760831884));
#56961=CARTESIAN_POINT('Ctrl Pts',(3.04623977506,-35.3803114393,0.440579215085));
#56962=CARTESIAN_POINT('Ctrl Pts',(3.04574061974,-35.3919185251,0.441351532501));
#56963=CARTESIAN_POINT('Ctrl Pts',(3.04580294181,-35.4035256109,0.442075517619));
#56964=CARTESIAN_POINT('Ctrl Pts',(3.05133592857,-35.3454968218,0.440376332259));
#56965=CARTESIAN_POINT('Ctrl Pts',(3.049131145,-35.3569269779,0.441037311376));
#56966=CARTESIAN_POINT('Ctrl Pts',(3.04748040649,-35.368466371,0.44165738234));
#56967=CARTESIAN_POINT('Ctrl Pts',(3.04639064899,-35.3800790478,0.442234462677));
#56968=CARTESIAN_POINT('Ctrl Pts',(3.04586531061,-35.3917283673,0.442766727044));
#56969=CARTESIAN_POINT('Ctrl Pts',(3.04590426722,-35.4033776868,0.443252644519));
#56970=CARTESIAN_POINT('Ctrl Pts',(3.05157202469,-35.345201709,0.44278366337));
#56971=CARTESIAN_POINT('Ctrl Pts',(3.04933300313,-35.3566718646,0.443200875235));
#56972=CARTESIAN_POINT('Ctrl Pts',(3.04765109714,-35.3682522692,0.443576907233));
#56973=CARTESIAN_POINT('Ctrl Pts',(3.04653338889,-35.3799066391,0.443910429375));
#56974=CARTESIAN_POINT('Ctrl Pts',(3.04598342453,-35.3915979921,0.44420038209));
#56975=CARTESIAN_POINT('Ctrl Pts',(3.0460011471,-35.4032893451,0.444445979659));
#56976=CARTESIAN_POINT('Ctrl Pts',(3.05179796269,-35.3449700438,0.445216729023));
#56977=CARTESIAN_POINT('Ctrl Pts',(3.04952458771,-35.3564797113,0.445388154931));
#56978=CARTESIAN_POINT('Ctrl Pts',(3.04781198307,-35.3681007576,0.445518095267));
#56979=CARTESIAN_POINT('Ctrl Pts',(3.04666739039,-35.3797965316,0.445605990135));
#56980=CARTESIAN_POINT('Ctrl Pts',(3.04609446477,-35.3915296692,0.44565156091));
#56981=CARTESIAN_POINT('Ctrl Pts',(3.04609320711,-35.4032628068,0.445654782512));
#56982=CARTESIAN_POINT('Ctrl Pts',(3.05201291474,-35.344804036,0.447673318567));
#56983=CARTESIAN_POINT('Ctrl Pts',(3.04970513582,-35.3563526648,0.447597170527));
#56984=CARTESIAN_POINT('Ctrl Pts',(3.04796238182,-35.3680139256,0.447479196662));
#56985=CARTESIAN_POINT('Ctrl Pts',(3.04679206061,-35.3797507581,0.447319633895));
#56986=CARTESIAN_POINT('Ctrl Pts',(3.04619793931,-35.3915253768,0.447118989828));
#56987=CARTESIAN_POINT('Ctrl Pts',(3.04618007217,-35.4032999955,0.446878030094));
#56988=CARTESIAN_POINT('Ctrl Pts',(3.05221609529,-35.3447053607,0.45015055449));
#56989=CARTESIAN_POINT('Ctrl Pts',(3.04987393679,-35.3562923356,0.449825338819));
#56990=CARTESIAN_POINT('Ctrl Pts',(3.04810166196,-35.3679933207,0.449457922766));
#56991=CARTESIAN_POINT('Ctrl Pts',(3.04690685539,-35.3797708063,0.449049358968));
#56992=CARTESIAN_POINT('Ctrl Pts',(3.04629339744,-35.3915865426,0.448600974315));
#56993=CARTESIAN_POINT('Ctrl Pts',(3.0462613893,-35.403402279,0.448114344323));
#56994=CARTESIAN_POINT('',(3.05221609413,-35.3447053607,0.450150554363));
#56995=CARTESIAN_POINT('Origin',(3.34555850698237,-35.4033872461924,0.428430037062882));
#56996=CARTESIAN_POINT('Origin',(3.03578495082005,-35.4311381890655,0.45269626373329));
#56997=CARTESIAN_POINT('Ctrl Pts',(3.05220443551777,-35.344591778873,0.449686712477512));
#56998=CARTESIAN_POINT('Ctrl Pts',(3.0498551255609,-35.3561950376791,0.449361491242345));
#56999=CARTESIAN_POINT('Ctrl Pts',(3.04807734683564,-35.3679128088571,0.448993942438477));
#57000=CARTESIAN_POINT('Ctrl Pts',(3.04687872963453,-35.3797074189195,0.448585121824359));
#57001=CARTESIAN_POINT('Ctrl Pts',(3.04626317818814,-35.3915404490275,0.448136361067163));
#57002=CARTESIAN_POINT('Ctrl Pts',(3.04623079520836,-35.4033734790351,0.447649241926326));
#57003=CARTESIAN_POINT('Ctrl Pts',(3.08188814853274,-35.3301154645781,0.811301434518424));
#57004=CARTESIAN_POINT('Ctrl Pts',(3.07719180838287,-35.3473672155455,0.810925370095392));
#57005=CARTESIAN_POINT('Ctrl Pts',(3.07363462275993,-35.3649068079318,0.810462755253741));
#57006=CARTESIAN_POINT('Ctrl Pts',(3.07123958057232,-35.3826400500681,0.809915880370152));
#57007=CARTESIAN_POINT('Ctrl Pts',(3.07001845225687,-35.4004701197944,0.809287880684534));
#57008=CARTESIAN_POINT('Ctrl Pts',(3.06997148677425,-35.41830018942,0.808582649476606));
#57009=CARTESIAN_POINT('Ctrl Pts',(3.11482379895319,-35.3179001315653,1.1741796201593));
#57010=CARTESIAN_POINT('Ctrl Pts',(3.10654999847949,-35.3398758977186,1.17391975325062));
#57011=CARTESIAN_POINT('Ctrl Pts',(3.10026437692076,-35.3625150846797,1.17350343193823));
#57012=CARTESIAN_POINT('Ctrl Pts',(3.09603282920114,-35.3856026344426,1.17293464162748));
#57013=CARTESIAN_POINT('Ctrl Pts',(3.09388918336483,-35.4089143804985,1.17221983646385));
#57014=CARTESIAN_POINT('Ctrl Pts',(3.09383396923983,-35.4322261265545,1.17136766300268));
#57015=CARTESIAN_POINT('Ctrl Pts',(3.14899944508157,-35.3090615611284,1.53617325026364));
#57016=CARTESIAN_POINT('Ctrl Pts',(3.1367101555031,-35.3343621966333,1.53613435112931));
#57017=CARTESIAN_POINT('Ctrl Pts',(3.12729631378655,-35.3609871657593,1.53585839375451));
#57018=CARTESIAN_POINT('Ctrl Pts',(3.12093762711669,-35.3885169025336,1.53534859968354));
#57019=CARTESIAN_POINT('Ctrl Pts',(3.11772689345012,-35.4164990521042,1.53461531686096));
#57020=CARTESIAN_POINT('Ctrl Pts',(3.11766502652187,-35.4444812016747,1.53367491460431));
#57021=CARTESIAN_POINT('Ctrl Pts',(3.18317242840243,-35.3024139984956,1.89900948084932));
#57022=CARTESIAN_POINT('Ctrl Pts',(3.16696570563031,-35.3301602171214,1.89925261763301));
#57023=CARTESIAN_POINT('Ctrl Pts',(3.15442927680899,-35.3600129806224,1.89918994885649));
#57024=CARTESIAN_POINT('Ctrl Pts',(3.14592306246191,-35.3913305665038,1.89881732341841));
#57025=CARTESIAN_POINT('Ctrl Pts',(3.14163831779052,-35.4233809324929,1.89814458126707));
#57026=CARTESIAN_POINT('Ctrl Pts',(3.14157580097331,-35.4554312984821,1.89719411861838));
#57027=CARTESIAN_POINT('Ctrl Pts',(3.21702289873695,-35.2974551605344,2.2623967664111));
#57028=CARTESIAN_POINT('Ctrl Pts',(3.19709436867799,-35.3269668716473,2.26291650186676));
#57029=CARTESIAN_POINT('Ctrl Pts',(3.18153205145727,-35.3594334352724,2.26306983940211));
#57030=CARTESIAN_POINT('Ctrl Pts',(3.17092279371148,-35.3939890002597,2.26284138838012));
#57031=CARTESIAN_POINT('Ctrl Pts',(3.16558686556525,-35.429590274611,2.26223804886464));
#57032=CARTESIAN_POINT('Ctrl Pts',(3.16552436512682,-35.4651915489622,2.26128784530879));
#57033=CARTESIAN_POINT('',(3.21673308953453,-35.2978265044789,2.26193293203227));
#57034=CARTESIAN_POINT('Origin',(3.46485271691158,-35.4651808043912,2.24112619649787));
#57035=CARTESIAN_POINT('Ctrl Pts',(3.05221609413,-35.3447053607,0.450150554363));
#57036=CARTESIAN_POINT('Ctrl Pts',(3.09862686998935,-35.32217505587,1.01604816889915));
#57037=CARTESIAN_POINT('Ctrl Pts',(3.15705633676715,-35.3065450332706,1.62042102657061));
#57038=CARTESIAN_POINT('Ctrl Pts',(3.2167330984,-35.297826491,2.26193292922));
#57039=CARTESIAN_POINT('Ctrl Pts',(3.21673308013,-35.297826519,2.26193293676));
#57040=CARTESIAN_POINT('Ctrl Pts',(3.19690170746,-35.3272920967,2.26244743731));
#57041=CARTESIAN_POINT('Ctrl Pts',(3.18141841353,-35.3596904513,2.26259731642));
#57042=CARTESIAN_POINT('Ctrl Pts',(3.17086410369,-35.3941615562,2.26236742048));
#57043=CARTESIAN_POINT('Ctrl Pts',(3.16555572757,-35.4296702319,2.26176465335));
#57044=CARTESIAN_POINT('Ctrl Pts',(3.16549338332,-35.4651789077,2.26081682416));
#57045=CARTESIAN_POINT('Ctrl Pts',(3.22044227874,-35.2947170616,2.28115435818));
#57046=CARTESIAN_POINT('Ctrl Pts',(3.19950860612,-35.3245433432,2.27888894627));
#57047=CARTESIAN_POINT('Ctrl Pts',(3.18307576937,-35.3575027832,2.27596054224));
#57048=CARTESIAN_POINT('Ctrl Pts',(3.17178564006,-35.3926825601,2.27243438801));
#57049=CARTESIAN_POINT('Ctrl Pts',(3.16599327189,-35.4289738974,2.26841670742));
#57050=CARTESIAN_POINT('Ctrl Pts',(3.16570519157,-35.4652652348,2.26403697776));
#57051=CARTESIAN_POINT('Ctrl Pts',(3.22504500396,-35.2927962885,2.30073764763));
#57052=CARTESIAN_POINT('Ctrl Pts',(3.20268941154,-35.3227611226,2.2957495854));
#57053=CARTESIAN_POINT('Ctrl Pts',(3.18504154424,-35.3561044246,2.28975874044));
#57054=CARTESIAN_POINT('Ctrl Pts',(3.1728278134,-35.3918504917,2.28291889281));
#57055=CARTESIAN_POINT('Ctrl Pts',(3.16645576111,-35.428799749,2.27544850897));
#57056=CARTESIAN_POINT('Ctrl Pts',(3.16593909074,-35.4657490064,2.26759298308));
#57057=CARTESIAN_POINT('Ctrl Pts',(3.23041275638,-35.292377214,2.32058136088));
#57058=CARTESIAN_POINT('Ctrl Pts',(3.20637961829,-35.3222393286,2.31311572454));
#57059=CARTESIAN_POINT('Ctrl Pts',(3.18729883271,-35.3557626768,2.30425560397));
#57060=CARTESIAN_POINT('Ctrl Pts',(3.1740077501,-35.391902145,2.29425266577));
#57061=CARTESIAN_POINT('Ctrl Pts',(3.16698247964,-35.4293517376,2.28345602024));
#57062=CARTESIAN_POINT('Ctrl Pts',(3.16624513219,-35.4668013301,2.2722457786));
#57063=CARTESIAN_POINT('Ctrl Pts',(3.2362706081,-35.293523699,2.3402171845));
#57064=CARTESIAN_POINT('Ctrl Pts',(3.21039981727,-35.3231016776,2.33049644021));
#57065=CARTESIAN_POINT('Ctrl Pts',(3.18974009686,-35.3566452436,2.31893365909));
#57066=CARTESIAN_POINT('Ctrl Pts',(3.17526480943,-35.3930381712,2.30588852441));
#57067=CARTESIAN_POINT('Ctrl Pts',(3.16753533529,-35.4308584528,2.2918609559));
#57068=CARTESIAN_POINT('Ctrl Pts',(3.16658333925,-35.4686787344,2.27738759286));
#57069=CARTESIAN_POINT('Ctrl Pts',(3.24268782164,-35.2959076878,2.35939290014));
#57070=CARTESIAN_POINT('Ctrl Pts',(3.21479367828,-35.3250197311,2.34761644611));
#57071=CARTESIAN_POINT('Ctrl Pts',(3.19237820629,-35.3584237245,2.33347294503));
#57072=CARTESIAN_POINT('Ctrl Pts',(3.17658501762,-35.3949324563,2.31744225071));
#57073=CARTESIAN_POINT('Ctrl Pts',(3.16808413932,-35.4329970413,2.30020446638));
#57074=CARTESIAN_POINT('Ctrl Pts',(3.16691857253,-35.4710616262,2.28248419619));
#57075=CARTESIAN_POINT('',(3.24268782128875,-35.2959076708926,2.35939286373149));
#57076=CARTESIAN_POINT('Origin',(3.46627170195,-35.4710616254,2.26279399804));
#57077=CARTESIAN_POINT('Ctrl Pts',(3.21673308013,-35.297826519,2.26193293676));
#57078=CARTESIAN_POINT('Ctrl Pts',(3.21862893786144,-35.2962372030246,2.27175745310809));
#57079=CARTESIAN_POINT('Ctrl Pts',(3.22079144998373,-35.2950355889071,2.28162723545145));
#57080=CARTESIAN_POINT('Ctrl Pts',(3.22317351887659,-35.2942698852058,2.29151507432848));
#57081=CARTESIAN_POINT('Ctrl Pts',(3.22559924436156,-35.2934901483192,2.30158412935339));
#57082=CARTESIAN_POINT('Ctrl Pts',(3.22825105142807,-35.2931626326134,2.31167001671416));
#57083=CARTESIAN_POINT('Ctrl Pts',(3.23108861335652,-35.2932948476651,2.32171513954936));
#57084=CARTESIAN_POINT('Ctrl Pts',(3.23368257328602,-35.2934157121801,2.33089789812114));
#57085=CARTESIAN_POINT('Ctrl Pts',(3.23643096040602,-35.2939205810558,2.34004530617035));
#57086=CARTESIAN_POINT('Ctrl Pts',(3.23932672580918,-35.2947802838016,2.34911168757664));
#57087=CARTESIAN_POINT('Ctrl Pts',(3.2404252315784,-35.2951064111961,2.35255101048238));
#57088=CARTESIAN_POINT('Ctrl Pts',(3.24154526402325,-35.2954832297334,2.35597874623171));
#57089=CARTESIAN_POINT('Ctrl Pts',(3.24268781017429,-35.2959076835405,2.35939286587855));
#57090=CARTESIAN_POINT('Origin',(3.46627170195,-35.4710616254,2.26279399804));
#57091=CARTESIAN_POINT('Origin',(3.46628252368698,-35.4710657830243,2.26278661726328));
#57092=CARTESIAN_POINT('Ctrl Pts',(3.24268777888,-35.2959076894,2.3593927975));
#57093=CARTESIAN_POINT('Ctrl Pts',(3.23324424211,-35.3247373359,2.38980935628));
#57094=CARTESIAN_POINT('Ctrl Pts',(3.22953158346,-35.3580565085,2.41774990543));
#57095=CARTESIAN_POINT('Ctrl Pts',(3.23195755579,-35.3946355813,2.44191215472));
#57096=CARTESIAN_POINT('Ctrl Pts',(3.24041432389,-35.4328486033,2.46122208494));
#57097=CARTESIAN_POINT('Ctrl Pts',(3.25430421882,-35.4710616254,2.47509045608));
#57098=CARTESIAN_POINT('Ctrl Pts',(3.24863991984,-35.2942847243,2.3702266206));
#57099=CARTESIAN_POINT('Ctrl Pts',(3.23916638892,-35.3234356974,2.39881134044));
#57100=CARTESIAN_POINT('Ctrl Pts',(3.23504178418,-35.3568515124,2.42482352544));
#57101=CARTESIAN_POINT('Ctrl Pts',(3.23665426145,-35.3933501406,2.4471045325));
#57102=CARTESIAN_POINT('Ctrl Pts',(3.24393773616,-35.4313935606,2.46471965345));
#57103=CARTESIAN_POINT('Ctrl Pts',(3.25638647798,-35.4694369807,2.47716948856));
#57104=CARTESIAN_POINT('Ctrl Pts',(3.25487358313,-35.2930993638,2.38101394136));
#57105=CARTESIAN_POINT('Ctrl Pts',(3.24526333648,-35.3225008542,2.40777429176));
#57106=CARTESIAN_POINT('Ctrl Pts',(3.24064780293,-35.3559526709,2.43188619171));
#57107=CARTESIAN_POINT('Ctrl Pts',(3.24140158851,-35.3923204861,2.45231942081));
#57108=CARTESIAN_POINT('Ctrl Pts',(3.24749724241,-35.4301491895,2.46826188149));
#57109=CARTESIAN_POINT('Ctrl Pts',(3.25851062528,-35.4679778928,2.4792941471));
#57110=CARTESIAN_POINT('Ctrl Pts',(3.26132499233,-35.2924297767,2.39172809926));
#57111=CARTESIAN_POINT('Ctrl Pts',(3.25147493949,-35.3220109395,2.41666518604));
#57112=CARTESIAN_POINT('Ctrl Pts',(3.24629031107,-35.3554385943,2.43889159306));
#57113=CARTESIAN_POINT('Ctrl Pts',(3.24613606992,-35.3916231814,2.45749640868));
#57114=CARTESIAN_POINT('Ctrl Pts',(3.25101894524,-35.429190416,2.4717755436));
#57115=CARTESIAN_POINT('Ctrl Pts',(3.26059110338,-35.4667576505,2.4813793476));
#57116=CARTESIAN_POINT('Ctrl Pts',(3.27380803754,-35.2922400204,2.41170299529));
#57117=CARTESIAN_POINT('Ctrl Pts',(3.26330589806,-35.3220182267,2.4332062407));
#57118=CARTESIAN_POINT('Ctrl Pts',(3.25689030732,-35.3552760482,2.4519082859));
#57119=CARTESIAN_POINT('Ctrl Pts',(3.2549183258,-35.3910159567,2.4670879438));
#57120=CARTESIAN_POINT('Ctrl Pts',(3.25746361688,-35.4279972557,2.47822608485));
#57121=CARTESIAN_POINT('Ctrl Pts',(3.26429684209,-35.4649785547,2.48510046341));
#57122=CARTESIAN_POINT('Ctrl Pts',(3.28670020806,-35.294071477,2.43091483974));
#57123=CARTESIAN_POINT('Ctrl Pts',(3.27515379345,-35.3237564299,2.44902572332));
#57124=CARTESIAN_POINT('Ctrl Pts',(3.26720088432,-35.356600918,2.46426325104));
#57125=CARTESIAN_POINT('Ctrl Pts',(3.26320102423,-35.3916841292,2.47607069605));
#57126=CARTESIAN_POINT('Ctrl Pts',(3.26328224545,-35.4278894975,2.48407361934));
#57127=CARTESIAN_POINT('Ctrl Pts',(3.26732268033,-35.4640948659,2.48814770965));
#57128=CARTESIAN_POINT('Ctrl Pts',(3.29283605957,-35.2953609408,2.43972470037));
#57129=CARTESIAN_POINT('Ctrl Pts',(3.28071360005,-35.3249348657,2.4562706651));
#57130=CARTESIAN_POINT('Ctrl Pts',(3.27197052657,-35.3575262865,2.46991873562));
#57131=CARTESIAN_POINT('Ctrl Pts',(3.2669738349,-35.392260236,2.48016433481));
#57132=CARTESIAN_POINT('Ctrl Pts',(3.26588441111,-35.4280613535,2.48669778017));
#57133=CARTESIAN_POINT('Ctrl Pts',(3.26861160084,-35.463862471,2.48944754786));
#57134=CARTESIAN_POINT('Ctrl Pts',(3.29901947016,-35.297065145,2.44826966141));
#57135=CARTESIAN_POINT('Ctrl Pts',(3.28622719246,-35.3264553013,2.46326747504));
#57136=CARTESIAN_POINT('Ctrl Pts',(3.27662267867,-35.3587390046,2.47532721835));
#57137=CARTESIAN_POINT('Ctrl Pts',(3.27057612082,-35.3930615858,2.48402260776));
#57138=CARTESIAN_POINT('Ctrl Pts',(3.26826446238,-35.4284083467,2.48909446671));
#57139=CARTESIAN_POINT('Ctrl Pts',(3.26965390752,-35.4637551076,2.49049946556));
#57140=CARTESIAN_POINT('Ctrl Pts',(3.30528109747,-35.2990851344,2.45651115245));
#57141=CARTESIAN_POINT('Ctrl Pts',(3.29174991618,-35.3282259173,2.47004146075));
#57142=CARTESIAN_POINT('Ctrl Pts',(3.28123325218,-35.3601462025,2.48060016935));
#57143=CARTESIAN_POINT('Ctrl Pts',(3.27411284989,-35.3940266946,2.48780557152));
#57144=CARTESIAN_POINT('Ctrl Pts',(3.2705944695,-35.4288883397,2.49144945081));
#57145=CARTESIAN_POINT('Ctrl Pts',(3.27067475303,-35.4637499849,2.49153061051));
#57146=CARTESIAN_POINT('',(3.30528110210951,-35.2990851341165,2.45651115699452));
#57147=CARTESIAN_POINT('Origin',(3.48387386404311,-35.4637520991879,2.28046099487966));
#57148=CARTESIAN_POINT('Ctrl Pts',(3.24268782427112,-35.2959076878087,2.35939289967519));
#57149=CARTESIAN_POINT('Ctrl Pts',(3.24767529781159,-35.2945477578349,2.3684708690015));
#57150=CARTESIAN_POINT('Ctrl Pts',(3.25287413301336,-35.2935658779458,2.37746859783919));
#57151=CARTESIAN_POINT('Ctrl Pts',(3.25822104692206,-35.2930305733796,2.38636188968886));
#57152=CARTESIAN_POINT('Ctrl Pts',(3.26356796083076,-35.2924952688133,2.39525518153853));
#57153=CARTESIAN_POINT('Ctrl Pts',(3.26906288166411,-35.2924074772293,2.40404332277373));
#57154=CARTESIAN_POINT('Ctrl Pts',(3.27466035755344,-35.2927955912655,2.41266929519308));
#57155=CARTESIAN_POINT('Ctrl Pts',(3.27960885693669,-35.2931387070033,2.42029516443148));
#57156=CARTESIAN_POINT('Ctrl Pts',(3.28463783441383,-35.2938512388069,2.42779111046201));
#57157=CARTESIAN_POINT('Ctrl Pts',(3.28973967766946,-35.2949119682808,2.43511159557974));
#57158=CARTESIAN_POINT('Ctrl Pts',(3.29414279634187,-35.2958274252085,2.44142950130478));
#57159=CARTESIAN_POINT('Ctrl Pts',(3.29859918080919,-35.2970041061196,2.44761753756102));
#57160=CARTESIAN_POINT('Ctrl Pts',(3.30312239520438,-35.2984029479339,2.45365075531648));
#57161=CARTESIAN_POINT('Ctrl Pts',(3.3038401776055,-35.2986249281339,2.45460815798385));
#57162=CARTESIAN_POINT('Ctrl Pts',(3.30455970208021,-35.2988524136235,2.45556165911652));
#57163=CARTESIAN_POINT('Ctrl Pts',(3.30528109745196,-35.2990851344388,2.45651115246804));
#57164=CARTESIAN_POINT('Ctrl Pts',(3.30528115437,-35.2990850504,2.45651113175));
#57165=CARTESIAN_POINT('Ctrl Pts',(3.29174997169,-35.3282258256,2.47004153063));
#57166=CARTESIAN_POINT('Ctrl Pts',(3.28123332764,-35.3601461205,2.48060031812));
#57167=CARTESIAN_POINT('Ctrl Pts',(3.27411296889,-35.3940266351,2.48780578271));
#57168=CARTESIAN_POINT('Ctrl Pts',(3.27059465556,-35.4288883092,2.49144970493));
#57169=CARTESIAN_POINT('Ctrl Pts',(3.2706750272,-35.4637499833,2.49153088745));
#57170=CARTESIAN_POINT('Ctrl Pts',(3.52263014734,-35.2997786652,2.67764867799));
#57171=CARTESIAN_POINT('Ctrl Pts',(3.50832158865,-35.3287004593,2.68978061947));
#57172=CARTESIAN_POINT('Ctrl Pts',(3.49718986878,-35.3603042564,2.69922432977));
#57173=CARTESIAN_POINT('Ctrl Pts',(3.48962934617,-35.3937968185,2.70564685787));
#57174=CARTESIAN_POINT('Ctrl Pts',(3.48585336684,-35.4282347239,2.70886780417));
#57175=CARTESIAN_POINT('Ctrl Pts',(3.48586067783,-35.4626726292,2.70888759263));
#57176=CARTESIAN_POINT('Ctrl Pts',(3.71975032728,-35.2998840308,2.91888544948));
#57177=CARTESIAN_POINT('Ctrl Pts',(3.70452693031,-35.3287908762,2.92986690945));
#57178=CARTESIAN_POINT('Ctrl Pts',(3.69266813705,-35.3603788898,2.93839702263));
#57179=CARTESIAN_POINT('Ctrl Pts',(3.68459264153,-35.3938552567,2.94417305658));
#57180=CARTESIAN_POINT('Ctrl Pts',(3.68052780808,-35.4282767651,2.94703197385));
#57181=CARTESIAN_POINT('Ctrl Pts',(3.68047391974,-35.4626982735,2.94697615221));
#57182=CARTESIAN_POINT('Ctrl Pts',(3.89420210101,-35.2992579912,3.17776652664));
#57183=CARTESIAN_POINT('Ctrl Pts',(3.87780196962,-35.3284044612,3.18777591948));
#57184=CARTESIAN_POINT('Ctrl Pts',(3.86500520386,-35.3603251829,3.19553496378));
#57185=CARTESIAN_POINT('Ctrl Pts',(3.85627187964,-35.3942021449,3.20076023088));
#57186=CARTESIAN_POINT('Ctrl Pts',(3.85185292871,-35.4290582738,3.20330006316));
#57187=CARTESIAN_POINT('Ctrl Pts',(3.85174986217,-35.4639144026,3.20315896516));
#57188=CARTESIAN_POINT('Ctrl Pts',(4.25043308745,-35.2963608901,3.82861914207));
#57189=CARTESIAN_POINT('Ctrl Pts',(4.23039390269,-35.3265730217,3.83636634601));
#57190=CARTESIAN_POINT('Ctrl Pts',(4.21468510082,-35.3600305104,3.84233146345));
#57191=CARTESIAN_POINT('Ctrl Pts',(4.20392503792,-35.3957885434,3.84626231873));
#57192=CARTESIAN_POINT('Ctrl Pts',(4.19845399885,-35.4326982838,3.848026993));
#57193=CARTESIAN_POINT('Ctrl Pts',(4.19827560656,-35.4696080243,3.84763795769));
#57194=CARTESIAN_POINT('Ctrl Pts',(4.45858902825,-35.291449905,4.54475674437));
#57195=CARTESIAN_POINT('Ctrl Pts',(4.43308531823,-35.3233621358,4.54953750297));
#57196=CARTESIAN_POINT('Ctrl Pts',(4.41292476175,-35.3596262841,4.55315251935));
#57197=CARTESIAN_POINT('Ctrl Pts',(4.39907396454,-35.3990181868,4.55540464772));
#57198=CARTESIAN_POINT('Ctrl Pts',(4.39207409827,-35.4399769064,4.55619669281));
#57199=CARTESIAN_POINT('Ctrl Pts',(4.39192731775,-35.480935626,4.55555318454));
#57200=CARTESIAN_POINT('Ctrl Pts',(4.52558545037,-35.2885903077,4.9733945174));
#57201=CARTESIAN_POINT('Ctrl Pts',(4.4963387214,-35.3214318737,4.97577624036));
#57202=CARTESIAN_POINT('Ctrl Pts',(4.4730869275,-35.3595080502,4.97747837329));
#57203=CARTESIAN_POINT('Ctrl Pts',(4.45708682842,-35.4013807813,4.97836774601));
#57204=CARTESIAN_POINT('Ctrl Pts',(4.44904844444,-35.4451561726,4.97838721155));
#57205=CARTESIAN_POINT('Ctrl Pts',(4.44897072855,-35.4889315639,4.97757277822));
#57206=CARTESIAN_POINT('Ctrl Pts',(4.53663898841,-35.2864927806,5.40585813039));
#57207=CARTESIAN_POINT('Ctrl Pts',(4.5036945439,-35.3198754069,5.40486687422));
#57208=CARTESIAN_POINT('Ctrl Pts',(4.4772847339,-35.3595850208,5.403864254));
#57209=CARTESIAN_POINT('Ctrl Pts',(4.45905487062,-35.4039471568,5.40287237975));
#57210=CARTESIAN_POINT('Ctrl Pts',(4.44995084219,-35.450642856,5.40192600583));
#57211=CARTESIAN_POINT('Ctrl Pts',(4.44996438067,-35.4973385552,5.40106825188));
#57212=CARTESIAN_POINT('Ctrl Pts',(4.49212121119,-35.2852060782,5.83250225872));
#57213=CARTESIAN_POINT('Ctrl Pts',(4.45609896624,-35.3187908717,5.82727331029));
#57214=CARTESIAN_POINT('Ctrl Pts',(4.42697004659,-35.3598847947,5.82278629135));
#57215=CARTESIAN_POINT('Ctrl Pts',(4.40679132226,-35.4065868399,5.81933946513));
#57216=CARTESIAN_POINT('Ctrl Pts',(4.39676913356,-35.4561050288,5.8171388925));
#57217=CARTESIAN_POINT('Ctrl Pts',(4.39688476736,-35.5056232176,5.81623445774));
#57218=CARTESIAN_POINT('',(4.49212120455654,-35.2852060791303,5.8325022569351));
#57219=CARTESIAN_POINT('Origin',(4.69448464672372,-35.5056329710941,5.8542829595805));
#57220=CARTESIAN_POINT('Ctrl Pts',(3.30528111534306,-35.2990851344485,2.45651117077468));
#57221=CARTESIAN_POINT('Ctrl Pts',(3.36062613515312,-35.2992617286018,2.5128208708643));
#57222=CARTESIAN_POINT('Ctrl Pts',(3.416086838459,-35.2993978352638,2.57241171064848));
#57223=CARTESIAN_POINT('Ctrl Pts',(3.47126284716246,-35.2994805332259,2.63546717927527));
#57224=CARTESIAN_POINT('Ctrl Pts',(3.52540792063213,-35.2995616860193,2.69734448902798));
#57225=CARTESIAN_POINT('Ctrl Pts',(3.5792787609624,-35.299591322044,2.76255861405961));
#57226=CARTESIAN_POINT('Ctrl Pts',(3.63245486835527,-35.2995592106656,2.83125670383386));
#57227=CARTESIAN_POINT('Ctrl Pts',(3.68420374847358,-35.2995279611448,2.89811096200321));
#57228=CARTESIAN_POINT('Ctrl Pts',(3.73529451314419,-35.2994381618817,2.96826505591086));
#57229=CARTESIAN_POINT('Ctrl Pts',(3.78530126722225,-35.2992834232217,3.04182356895941));
#57230=CARTESIAN_POINT('Ctrl Pts',(3.80177924062247,-35.2992324345189,3.06606219919488));
#57231=CARTESIAN_POINT('Ctrl Pts',(3.81813920729258,-35.2991744243497,3.09067020136823));
#57232=CARTESIAN_POINT('Ctrl Pts',(3.83436503438466,-35.2991092594134,3.11565044021741));
#57233=CARTESIAN_POINT('Ctrl Pts',(3.88203349803657,-35.2989178169445,3.18903773818631));
#57234=CARTESIAN_POINT('Ctrl Pts',(3.92854659437473,-35.2986642858774,3.26564064025194));
#57235=CARTESIAN_POINT('Ctrl Pts',(3.97347340024928,-35.2983481716719,3.34550625691759));
#57236=CARTESIAN_POINT('Ctrl Pts',(4.01705811664467,-35.2980415006827,3.4229860640028));
#57237=CARTESIAN_POINT('Ctrl Pts',(4.05914965679832,-35.2976758978132,3.50353684824634));
#57238=CARTESIAN_POINT('Ctrl Pts',(4.09932647608738,-35.2972554741226,3.58716217895609));
#57239=CARTESIAN_POINT('Ctrl Pts',(4.12275798127302,-35.2970102790062,3.63593327146291));
#57240=CARTESIAN_POINT('Ctrl Pts',(4.14553770629444,-35.2967465263988,3.68574934450856));
#57241=CARTESIAN_POINT('Ctrl Pts',(4.16757792554145,-35.296465838294,3.73660398153786));
#57242=CARTESIAN_POINT('Ctrl Pts',(4.201498880351,-35.2960338458346,3.81487170769765));
#57243=CARTESIAN_POINT('Ctrl Pts',(4.23366892450562,-35.2955616315989,3.89560128685815));
#57244=CARTESIAN_POINT('Ctrl Pts',(4.26375490829378,-35.2950584202033,3.97874208646125));
#57245=CARTESIAN_POINT('Ctrl Pts',(4.26669543912757,-35.2950092375462,3.98686806587081));
#57246=CARTESIAN_POINT('Ctrl Pts',(4.26993248876024,-35.2949543601435,3.9959049877927));
#57247=CARTESIAN_POINT('Ctrl Pts',(4.2727290262001,-35.2949073184052,4.00379030146189));
#57248=CARTESIAN_POINT('Ctrl Pts',(4.27354346307177,-35.2948936184184,4.00608674495136));
#57249=CARTESIAN_POINT('Ctrl Pts',(4.27432087485892,-35.2948805857688,4.00828539207123));
#57250=CARTESIAN_POINT('Ctrl Pts',(4.27504380979966,-35.294868560589,4.01033502539987));
#57251=CARTESIAN_POINT('Ctrl Pts',(4.31123404893338,-35.294266578163,4.11293999871085));
#57252=CARTESIAN_POINT('Ctrl Pts',(4.34336177273321,-35.2936522261943,4.21671280069685));
#57253=CARTESIAN_POINT('Ctrl Pts',(4.37143663731291,-35.293027724738,4.32157074836816));
#57254=CARTESIAN_POINT('Ctrl Pts',(4.39964431341538,-35.2924002690024,4.42692473916969));
#57255=CARTESIAN_POINT('Ctrl Pts',(4.42376085007101,-35.2917625780507,4.53337486959008));
#57256=CARTESIAN_POINT('Ctrl Pts',(4.44374590523629,-35.2911134178544,4.64085244068075));
#57257=CARTESIAN_POINT('Ctrl Pts',(4.46024409592059,-35.2905775189733,4.72957801323864));
#57258=CARTESIAN_POINT('Ctrl Pts',(4.47392582307022,-35.2900337287775,4.81900424037342));
#57259=CARTESIAN_POINT('Ctrl Pts',(4.48474179324417,-35.2894796369031,4.90909506800667));
#57260=CARTESIAN_POINT('Ctrl Pts',(4.49963111233193,-35.2887168712344,5.03311455566615));
#57261=CARTESIAN_POINT('Ctrl Pts',(4.50891101504119,-35.288019710402,5.15755949064399));
#57262=CARTESIAN_POINT('Ctrl Pts',(4.51258247618356,-35.2874031701943,5.28190637099523));
#57263=CARTESIAN_POINT('Ctrl Pts',(4.51618936873142,-35.2867974728454,5.40406640992722));
#57264=CARTESIAN_POINT('Ctrl Pts',(4.51438337543916,-35.2862696797958,5.52613139504472));
#57265=CARTESIAN_POINT('Ctrl Pts',(4.50721377571749,-35.285823887096,5.64761401154141));
#57266=CARTESIAN_POINT('Ctrl Pts',(4.50356644424897,-35.2855971026443,5.70941486336414));
#57267=CARTESIAN_POINT('Ctrl Pts',(4.4985318012427,-35.285391367349,5.77106518411329));
#57268=CARTESIAN_POINT('Ctrl Pts',(4.49212120720968,-35.2852060820123,5.83250225711667));
#57269=CARTESIAN_POINT('Ctrl Pts',(4.4921212186,-35.2852060642,5.83250225932));
#57270=CARTESIAN_POINT('Ctrl Pts',(4.45609896257,-35.3187908592,5.82727337616));
#57271=CARTESIAN_POINT('Ctrl Pts',(4.42697003004,-35.3598847848,5.82278643887));
#57272=CARTESIAN_POINT('Ctrl Pts',(4.40679129181,-35.4065868334,5.81933970701));
#57273=CARTESIAN_POINT('Ctrl Pts',(4.39676908915,-35.4561050262,5.81713923581));
#57274=CARTESIAN_POINT('Ctrl Pts',(4.39688470965,-35.505623219,5.81623490373));
#57275=CARTESIAN_POINT('Ctrl Pts',(4.47934426829,-35.2848180141,5.95513865982));
#57276=CARTESIAN_POINT('Ctrl Pts',(4.44240767125,-35.3184648135,5.94886804446));
#57277=CARTESIAN_POINT('Ctrl Pts',(4.41246275486,-35.3599636587,5.94360014588));
#57278=CARTESIAN_POINT('Ctrl Pts',(4.39168683777,-35.4073477788,5.9397026792));
#57279=CARTESIAN_POINT('Ctrl Pts',(4.38136362076,-35.457688004,5.93741576176));
#57280=CARTESIAN_POINT('Ctrl Pts',(4.38147338286,-35.5080282291,5.93677544119));
#57281=CARTESIAN_POINT('Ctrl Pts',(4.46080331489,-35.2846612104,6.0774500678));
#57282=CARTESIAN_POINT('Ctrl Pts',(4.42339099946,-35.3183175745,6.07010629864));
#57283=CARTESIAN_POINT('Ctrl Pts',(4.39300176947,-35.3600459293,6.06403311375));
#57284=CARTESIAN_POINT('Ctrl Pts',(4.37188741448,-35.4078395887,6.05967077608));
#57285=CARTESIAN_POINT('Ctrl Pts',(4.36138132105,-35.4586803826,6.05729403028));
#57286=CARTESIAN_POINT('Ctrl Pts',(4.36146441688,-35.5095211765,6.05692288884));
#57287=CARTESIAN_POINT('Ctrl Pts',(4.43653605144,-35.2846213402,6.19885974208));
#57288=CARTESIAN_POINT('Ctrl Pts',(4.39907245731,-35.3182793407,6.19048378347));
#57289=CARTESIAN_POINT('Ctrl Pts',(4.36860698734,-35.360098105,6.18364473746));
#57290=CARTESIAN_POINT('Ctrl Pts',(4.34741298485,-35.4080551513,6.17885069748));
#57291=CARTESIAN_POINT('Ctrl Pts',(4.33684033846,-35.4590962326,6.17640727689));
#57292=CARTESIAN_POINT('Ctrl Pts',(4.33687279452,-35.5101373139,6.17631673235));
#57293=CARTESIAN_POINT('Ctrl Pts',(4.39382617826,-35.2846522393,6.3704629655));
#57294=CARTESIAN_POINT('Ctrl Pts',(4.35687304692,-35.3183144911,6.36073630622));
#57295=CARTESIAN_POINT('Ctrl Pts',(4.32681014412,-35.360077369,6.35290824863));
#57296=CARTESIAN_POINT('Ctrl Pts',(4.3058660926,-35.4079286751,6.34756704555));
#57297=CARTESIAN_POINT('Ctrl Pts',(4.295366459,-35.4588388005,6.34505127094));
#57298=CARTESIAN_POINT('Ctrl Pts',(4.29530142772,-35.5097489259,6.34533949948));
#57299=CARTESIAN_POINT('Ctrl Pts',(4.33989513123,-35.2849598896,6.53848806555));
#57300=CARTESIAN_POINT('Ctrl Pts',(4.30425869633,-35.3185874247,6.5277361976));
#57301=CARTESIAN_POINT('Ctrl Pts',(4.27529524943,-35.3599922268,6.51919887852));
#57302=CARTESIAN_POINT('Ctrl Pts',(4.25509182459,-35.4072223024,6.51350637116));
#57303=CARTESIAN_POINT('Ctrl Pts',(4.2448885603,-35.4573782014,6.51100829607));
#57304=CARTESIAN_POINT('Ctrl Pts',(4.2446848137,-35.5075341005,6.51166242388));
#57305=CARTESIAN_POINT('Ctrl Pts',(4.32271334112,-35.2850814359,6.58854936739));
#57306=CARTESIAN_POINT('Ctrl Pts',(4.28754475087,-35.3186934865,6.57751968609));
#57307=CARTESIAN_POINT('Ctrl Pts',(4.25897443759,-35.3599624877,6.56879320674));
#57308=CARTESIAN_POINT('Ctrl Pts',(4.23903851349,-35.4069590258,6.56300941547));
#57309=CARTESIAN_POINT('Ctrl Pts',(4.22894623833,-35.4568320218,6.56051917828));
#57310=CARTESIAN_POINT('Ctrl Pts',(4.22869977692,-35.5067050179,6.56127483435));
#57311=CARTESIAN_POINT('Ctrl Pts',(4.30455023491,-35.2852434072,6.6381975116));
#57312=CARTESIAN_POINT('Ctrl Pts',(4.26991817238,-35.3188318732,6.62693608199));
#57313=CARTESIAN_POINT('Ctrl Pts',(4.24179867527,-35.3599337083,6.61806209525));
#57314=CARTESIAN_POINT('Ctrl Pts',(4.22216945818,-35.4066468932,6.61221922778));
#57315=CARTESIAN_POINT('Ctrl Pts',(4.21220416739,-35.4561778332,6.6097570786));
#57316=CARTESIAN_POINT('Ctrl Pts',(4.21190811788,-35.5057087732,6.61062231004));
#57317=CARTESIAN_POINT('Ctrl Pts',(4.28541381497,-35.285453273,6.6874287475));
#57318=CARTESIAN_POINT('Ctrl Pts',(4.251389142,-35.3190062299,6.67597342108));
#57319=CARTESIAN_POINT('Ctrl Pts',(4.22378115684,-35.359906937,6.66698096996));
#57320=CARTESIAN_POINT('Ctrl Pts',(4.20450211564,-35.4062855347,6.66109555831));
#57321=CARTESIAN_POINT('Ctrl Pts',(4.19468580977,-35.4554145194,6.65866330444));
#57322=CARTESIAN_POINT('Ctrl Pts',(4.1943405656,-35.5045435041,6.65962635024));
#57323=CARTESIAN_POINT('',(4.28541381260123,-35.2854532749764,6.68742874668675));
#57324=CARTESIAN_POINT('Origin',(4.4767625297971,-35.5045528794638,6.76087257923098));
#57325=CARTESIAN_POINT('Ctrl Pts',(4.49212120362943,-35.2852060781576,5.83250225714692));
#57326=CARTESIAN_POINT('Ctrl Pts',(4.48501821379885,-35.28499034928,5.90067858056652));
#57327=CARTESIAN_POINT('Ctrl Pts',(4.475829510371,-35.2848603581573,5.96821991475356));
#57328=CARTESIAN_POINT('Ctrl Pts',(4.46467408476022,-35.2847795393672,6.03493028032477));
#57329=CARTESIAN_POINT('Ctrl Pts',(4.45188175642594,-35.2846868615497,6.1114294592411));
#57330=CARTESIAN_POINT('Ctrl Pts',(4.43650318723529,-35.2846578504948,6.18683720321124));
#57331=CARTESIAN_POINT('Ctrl Pts',(4.41873689817154,-35.2846719377395,6.26092150264478));
#57332=CARTESIAN_POINT('Ctrl Pts',(4.4044190107383,-35.2846832906779,6.32062618582616));
#57333=CARTESIAN_POINT('Ctrl Pts',(4.38855082920743,-35.2847233237578,6.3794730929799));
#57334=CARTESIAN_POINT('Ctrl Pts',(4.37124286446852,-35.2848002119189,6.43735428099128));
#57335=CARTESIAN_POINT('Ctrl Pts',(4.35373712223533,-35.2848779786783,6.49589687526874));
#57336=CARTESIAN_POINT('Ctrl Pts',(4.33475645529202,-35.2849936461652,6.55345665712876));
#57337=CARTESIAN_POINT('Ctrl Pts',(4.31442499448376,-35.2851691523084,6.60992387941392));
#57338=CARTESIAN_POINT('Ctrl Pts',(4.30503833801705,-35.2852501802231,6.63599374336607));
#57339=CARTESIAN_POINT('Ctrl Pts',(4.29536409669719,-35.2853441502275,6.66183019340778));
#57340=CARTESIAN_POINT('Ctrl Pts',(4.28541381473644,-35.2854532732707,6.68742874730075));
#57341=CARTESIAN_POINT('Ctrl Pts',(4.2857571149995,-35.2854498008873,6.68654438213887));
#57342=CARTESIAN_POINT('Ctrl Pts',(4.25155378038641,-35.3191684201121,6.67503743859588));
#57343=CARTESIAN_POINT('Ctrl Pts',(4.22383204100074,-35.3603102200634,6.6660165794383));
#57344=CARTESIAN_POINT('Ctrl Pts',(4.20453371664109,-35.4069770322371,6.66013544312534));
#57345=CARTESIAN_POINT('Ctrl Pts',(4.19480628016729,-35.4563954305725,6.65774375063294));
#57346=CARTESIAN_POINT('Ctrl Pts',(4.19464691082663,-35.5057728190552,6.65877872825311));
#57347=CARTESIAN_POINT('Ctrl Pts',(4.11435014520936,-35.2871852849674,7.12824617423143));
#57348=CARTESIAN_POINT('Ctrl Pts',(4.08577860869936,-35.3206021659747,7.11438447090243));
#57349=CARTESIAN_POINT('Ctrl Pts',(4.06287836005714,-35.3599631233916,7.10355205693462));
#57350=CARTESIAN_POINT('Ctrl Pts',(4.04699017908423,-35.4036584698343,7.09644153341169));
#57351=CARTESIAN_POINT('Ctrl Pts',(4.03888572751518,-35.4495094136804,7.09342297952844));
#57352=CARTESIAN_POINT('Ctrl Pts',(4.03857492304847,-35.4953282298792,7.09444332714258));
#57353=CARTESIAN_POINT('Ctrl Pts',(3.87834409676772,-35.2903635149614,7.54483809333952));
#57354=CARTESIAN_POINT('Ctrl Pts',(3.85593408038674,-35.3229175784704,7.53014366147255));
#57355=CARTESIAN_POINT('Ctrl Pts',(3.83817610056273,-35.3599431212855,7.51876969980455));
#57356=CARTESIAN_POINT('Ctrl Pts',(3.82587986171587,-35.4001589270382,7.51130626410611));
#57357=CARTESIAN_POINT('Ctrl Pts',(3.81949988822795,-35.4419595846812,7.5080608625387));
#57358=CARTESIAN_POINT('Ctrl Pts',(3.819053097548,-35.4837366209665,7.5089954441848));
#57359=CARTESIAN_POINT('Ctrl Pts',(3.58344977045482,-35.2955229188271,7.9236050894372));
#57360=CARTESIAN_POINT('Ctrl Pts',(3.56687361287628,-35.3263185284973,7.90983251579037));
#57361=CARTESIAN_POINT('Ctrl Pts',(3.55380176218302,-35.3602864301414,7.89927969686287));
#57362=CARTESIAN_POINT('Ctrl Pts',(3.54470005686475,-35.3964847830565,7.892361948371));
#57363=CARTESIAN_POINT('Ctrl Pts',(3.53982931256782,-35.433790776985,7.88929217376211));
#57364=CARTESIAN_POINT('Ctrl Pts',(3.53920539592514,-35.4710802621639,7.89004706986091));
#57365=CARTESIAN_POINT('Ctrl Pts',(2.7884326259249,-35.3119516745262,8.68810001722839));
#57366=CARTESIAN_POINT('Ctrl Pts',(2.78288166507677,-35.3368781016926,8.6783873695996));
#57367=CARTESIAN_POINT('Ctrl Pts',(2.77860928612365,-35.362795726313,8.67108096090887));
#57368=CARTESIAN_POINT('Ctrl Pts',(2.7756311279895,-35.3893740464784,8.66629508813301));
#57369=CARTESIAN_POINT('Ctrl Pts',(2.77395449793439,-35.4162800377925,8.66408572229646));
#57370=CARTESIAN_POINT('Ctrl Pts',(2.77358557207991,-35.4431811452579,8.66445053727045));
#57371=CARTESIAN_POINT('Ctrl Pts',(1.7897157019,-35.3293337971,9.16292213266));
#57372=CARTESIAN_POINT('Ctrl Pts',(1.78816995510962,-35.3472022339894,9.15780424233925));
#57373=CARTESIAN_POINT('Ctrl Pts',(1.78689877850668,-35.3654037562666,9.15395288550329));
#57374=CARTESIAN_POINT('Ctrl Pts',(1.78591133611386,-35.3838310440629,9.15138999603306));
#57375=CARTESIAN_POINT('Ctrl Pts',(1.78521442899343,-35.4023704701083,9.15012684960892));
#57376=CARTESIAN_POINT('Ctrl Pts',(1.78480953452593,-35.4209082248919,9.15016379054982));
#57377=CARTESIAN_POINT('Ctrl Pts',(1.17958127456,-35.3376427744,9.32328709823));
#57378=CARTESIAN_POINT('Ctrl Pts',(1.1795177740293,-35.3527252284187,9.31930419456785));
#57379=CARTESIAN_POINT('Ctrl Pts',(1.17962324905309,-35.3680915604398,9.31631951498919));
#57380=CARTESIAN_POINT('Ctrl Pts',(1.17989610757511,-35.3836484756564,9.31435986643977));
#57381=CARTESIAN_POINT('Ctrl Pts',(1.18033338523472,-35.3992999531728,9.31343839198126));
#57382=CARTESIAN_POINT('Ctrl Pts',(1.18093154393229,-35.4149500212705,9.31355423483848));
#57383=CARTESIAN_POINT('Ctrl Pts',(0.559260434794,-35.3376563848,9.36581532526));
#57384=CARTESIAN_POINT('Ctrl Pts',(0.558544684725532,-35.3519810096587,
9.36214503977062));
#57385=CARTESIAN_POINT('Ctrl Pts',(0.557873133674002,-35.366519714233,9.35935950961906));
#57386=CARTESIAN_POINT('Ctrl Pts',(0.557250656370557,-35.3812021204197,
9.35747655687641));
#57387=CARTESIAN_POINT('Ctrl Pts',(0.55668135112757,-35.3959558431041,9.35650540869865));
#57388=CARTESIAN_POINT('Ctrl Pts',(0.556168381827813,-35.4107085027404,
9.35644644218252));
#57389=CARTESIAN_POINT('Ctrl Pts',(-0.051310852811,-35.3354014219,9.29455995377));
#57390=CARTESIAN_POINT('Ctrl Pts',(-0.0507122350892525,-35.3509096123029,
9.29036543781367));
#57391=CARTESIAN_POINT('Ctrl Pts',(-0.0502350705067947,-35.366701542761,
9.28720264732302));
#57392=CARTESIAN_POINT('Ctrl Pts',(-0.0498829422298899,-35.3826844332909,
9.28509669210183));
#57393=CARTESIAN_POINT('Ctrl Pts',(-0.0496579695573275,-35.3987620938252,
9.28406024710945));
#57394=CARTESIAN_POINT('Ctrl Pts',(-0.049560732354575,-35.4148383418483,
9.28409309993256));
#57395=CARTESIAN_POINT('Ctrl Pts',(4.28541380927,-35.2854532781,6.68742874581));
#57396=CARTESIAN_POINT('Ctrl Pts',(4.24024106746993,-35.2859109819706,6.80375439668074));
#57397=CARTESIAN_POINT('Ctrl Pts',(4.18962800213566,-35.2865074754667,6.91808857909236));
#57398=CARTESIAN_POINT('Ctrl Pts',(4.1338105460796,-35.2872466077222,7.02993790187778));
#57399=CARTESIAN_POINT('Ctrl Pts',(4.08906901210241,-35.2878390731132,7.11959283474865));
#57400=CARTESIAN_POINT('Ctrl Pts',(4.04098438539919,-35.2885230593247,7.20765199327025));
#57401=CARTESIAN_POINT('Ctrl Pts',(3.98969543243286,-35.2892965735864,7.29387761510677));
#57402=CARTESIAN_POINT('Ctrl Pts',(3.93205810027539,-35.2901658309188,7.39077596297399));
#57403=CARTESIAN_POINT('Ctrl Pts',(3.87037356895584,-35.2911490776896,7.4853566990516));
#57404=CARTESIAN_POINT('Ctrl Pts',(3.80486079630046,-35.292245051124,7.57729493777813));
#57405=CARTESIAN_POINT('Ctrl Pts',(3.77210440997277,-35.2927930378412,7.62326405714139));
#57406=CARTESIAN_POINT('Ctrl Pts',(3.73839133114429,-35.2933692054693,7.66857282309408));
#57407=CARTESIAN_POINT('Ctrl Pts',(3.70375113596166,-35.2939734289908,7.71318231425977));
#57408=CARTESIAN_POINT('Ctrl Pts',(3.68643103837034,-35.2942755407515,7.73548705984261));
#57409=CARTESIAN_POINT('Ctrl Pts',(3.66887917674681,-35.2945846811323,7.75761699771901));
#57410=CARTESIAN_POINT('Ctrl Pts',(3.65109939460978,-35.2949008234548,7.77956738237956));
#57411=CARTESIAN_POINT('Ctrl Pts',(3.64220950354126,-35.295058894616,7.79054257470984));
#57412=CARTESIAN_POINT('Ctrl Pts',(3.63326263329915,-35.2952187171955,7.80147287941059));
#57413=CARTESIAN_POINT('Ctrl Pts',(3.62425927144795,-35.2953802907213,7.81235770916504));
#57414=CARTESIAN_POINT('Ctrl Pts',(3.61975759052235,-35.2954610774842,7.81780012404226));
#57415=CARTESIAN_POINT('Ctrl Pts',(3.61524178675509,-35.2955423020413,7.82323117023066));
#57416=CARTESIAN_POINT('Ctrl Pts',(3.61071192163445,-35.2956239643472,7.8286507747736));
#57417=CARTESIAN_POINT('Ctrl Pts',(3.60844698907413,-35.2956647955002,7.83136057704507));
#57418=CARTESIAN_POINT('Ctrl Pts',(3.60617854117927,-35.295705736094,7.8340675189082));
#57419=CARTESIAN_POINT('Ctrl Pts',(3.60390658567017,-35.2957467861229,7.83677159127279));
#57420=CARTESIAN_POINT('Ctrl Pts',(3.60163463016106,-35.2957878361517,7.83947566363739));
#57421=CARTESIAN_POINT('Ctrl Pts',(3.5984657767767,-35.295845173692,7.84323465315565));
#57422=CARTESIAN_POINT('Ctrl Pts',(3.59708020403902,-35.2958702645169,7.84487519079636));
#57423=CARTESIAN_POINT('Ctrl Pts',(3.57251009288989,-35.2963151955827,7.87396654852909));
#57424=CARTESIAN_POINT('Ctrl Pts',(3.54536199564617,-35.2968211811022,7.90528994862769));
#57425=CARTESIAN_POINT('Ctrl Pts',(3.51542410262016,-35.2973885258685,7.9386354704925));
#57426=CARTESIAN_POINT('Ctrl Pts',(3.48572084541715,-35.2979514241158,7.97171964951802));
#57427=CARTESIAN_POINT('Ctrl Pts',(3.45327090926628,-35.2985747630115,8.00679463923754));
#57428=CARTESIAN_POINT('Ctrl Pts',(3.41784676062168,-35.2992589206647,8.0436089066258));
#57429=CARTESIAN_POINT('Ctrl Pts',(3.38301285837218,-35.2999316787048,8.07980976509822));
#57430=CARTESIAN_POINT('Ctrl Pts',(3.34530251111634,-35.3006633028627,8.11769260113828));
#57431=CARTESIAN_POINT('Ctrl Pts',(3.30448645840364,-35.3014535220577,8.15696995549352));
#57432=CARTESIAN_POINT('Ctrl Pts',(3.27765591397394,-35.3019729748174,8.18278903232897));
#57433=CARTESIAN_POINT('Ctrl Pts',(3.24948309679918,-35.3025177359954,8.20920970917208));
#57434=CARTESIAN_POINT('Ctrl Pts',(3.21990151995639,-35.3030873574058,8.23613808459519));
#57435=CARTESIAN_POINT('Ctrl Pts',(3.17653599361247,-35.30392240188,8.27561411320639));
#57436=CARTESIAN_POINT('Ctrl Pts',(3.13014290708392,-35.3048106190462,8.31618346611674));
#57437=CARTESIAN_POINT('Ctrl Pts',(3.08051048119044,-35.305754786797,8.35750853562693));
#57438=CARTESIAN_POINT('Ctrl Pts',(3.03487856903338,-35.3066228519598,8.3955026877931));
#57439=CARTESIAN_POINT('Ctrl Pts',(2.98650811680595,-35.3075382802448,8.43413524351376));
#57440=CARTESIAN_POINT('Ctrl Pts',(2.93524278845432,-35.308499231208,8.47310597847456));
#57441=CARTESIAN_POINT('Ctrl Pts',(2.90959514805766,-35.3089799874137,8.49260273053693));
#57442=CARTESIAN_POINT('Ctrl Pts',(2.88322259430676,-35.3094725726033,8.51218358748032));
#57443=CARTESIAN_POINT('Ctrl Pts',(2.85610655008563,-35.3099778173175,8.53180663003467));
#57444=CARTESIAN_POINT('Ctrl Pts',(2.82664631909365,-35.3105267405256,8.55312608805378));
#57445=CARTESIAN_POINT('Ctrl Pts',(2.79630846918575,-35.3110906045039,8.57449539050833));
#57446=CARTESIAN_POINT('Ctrl Pts',(2.76506896671193,-35.3116707290185,8.59585757517973));
#57447=CARTESIAN_POINT('Ctrl Pts',(2.73507234703232,-35.3122277729229,8.61636985221264));
#57448=CARTESIAN_POINT('Ctrl Pts',(2.70424395977659,-35.3128021725465,8.63687447551125));
#57449=CARTESIAN_POINT('Ctrl Pts',(2.67256696449636,-35.313386467183,8.65732090004896));
#57450=CARTESIAN_POINT('Ctrl Pts',(2.66415276262506,-35.3135416704458,8.66275198156678));
#57451=CARTESIAN_POINT('Ctrl Pts',(2.65567867942147,-35.3136975738044,8.66817894503978));
#57452=CARTESIAN_POINT('Ctrl Pts',(2.6471443888335,-35.3138541517961,8.67360075492415));
#57453=CARTESIAN_POINT('Ctrl Pts',(2.64294391768473,-35.3139312175265,8.67626930197661));
#57454=CARTESIAN_POINT('Ctrl Pts',(2.63872886152726,-35.3140084466549,8.67893660035388));
#57455=CARTESIAN_POINT('Ctrl Pts',(2.63449918232813,-35.3140858359642,8.68160252527109));
#57456=CARTESIAN_POINT('Ctrl Pts',(2.63190476989879,-35.3141333052347,8.68323775773561));
#57457=CARTESIAN_POINT('Ctrl Pts',(2.62930485572997,-35.314180834769,8.68487247343467));
#57458=CARTESIAN_POINT('Ctrl Pts',(2.62669943115083,-35.314228423802,8.6865066434089));
#57459=CARTESIAN_POINT('Ctrl Pts',(2.62514069149448,-35.3142568947521,8.68748431344565));
#57460=CARTESIAN_POINT('Ctrl Pts',(2.62358292210444,-35.3142853333759,8.68845995462797));
#57461=CARTESIAN_POINT('Ctrl Pts',(2.6220064146994,-35.3143140988695,8.68944586462671));
#57462=CARTESIAN_POINT('Ctrl Pts',(2.61354724677354,-35.3144684477419,8.6947360257845));
#57463=CARTESIAN_POINT('Ctrl Pts',(2.60467180624005,-35.3146299330446,8.70024225252914));
#57464=CARTESIAN_POINT('Ctrl Pts',(2.59602944765013,-35.3147866965919,8.70555954544832));
#57465=CARTESIAN_POINT('Ctrl Pts',(2.59177578678166,-35.3148638536503,8.70817665055698));
#57466=CARTESIAN_POINT('Ctrl Pts',(2.58757877086762,-35.3149398678404,8.71074828419458));
#57467=CARTESIAN_POINT('Ctrl Pts',(2.58351682731367,-35.3150133321632,8.71322783392397));
#57468=CARTESIAN_POINT('Ctrl Pts',(2.58099028799958,-35.3150590271605,8.71477012021853));
#57469=CARTESIAN_POINT('Ctrl Pts',(2.57851601941034,-35.3151037357486,8.71627680231907));
#57470=CARTESIAN_POINT('Ctrl Pts',(2.57611300778938,-35.3151471203659,8.71773685678189));
#57471=CARTESIAN_POINT('Ctrl Pts',(2.57520999908579,-35.3151634235276,8.71828551908388));
#57472=CARTESIAN_POINT('Ctrl Pts',(2.57431880219543,-35.3151795082263,8.71882654127799));
#57473=CARTESIAN_POINT('Ctrl Pts',(2.57342464839827,-35.3151956411518,8.71936890343435));
#57474=CARTESIAN_POINT('Ctrl Pts',(2.50161040160182,-35.3164913621921,8.76292889263726));
#57475=CARTESIAN_POINT('Ctrl Pts',(2.43070155120575,-35.3177371289784,8.80298312010605));
#57476=CARTESIAN_POINT('Ctrl Pts',(2.36103654431604,-35.3189216230598,8.83985681612805));
#57477=CARTESIAN_POINT('Ctrl Pts',(2.29054178984295,-35.3201202251008,8.87716969763973));
#57478=CARTESIAN_POINT('Ctrl Pts',(2.22132063725928,-35.3212560237631,8.91122630180714));
#57479=CARTESIAN_POINT('Ctrl Pts',(2.1536701020784,-35.3223214184583,8.94236687148854));
#57480=CARTESIAN_POINT('Ctrl Pts',(2.08494789805377,-35.3234036903342,8.97400074662887));
#57481=CARTESIAN_POINT('Ctrl Pts',(2.0178463214947,-35.3244133041604,9.00262592005154));
#57482=CARTESIAN_POINT('Ctrl Pts',(1.95262311278269,-35.3253470381652,9.02859536222033));
#57483=CARTESIAN_POINT('Ctrl Pts',(1.88507526932016,-35.3263140515894,9.05549038699859));
#57484=CARTESIAN_POINT('Ctrl Pts',(1.81954192555313,-35.3271997062196,9.0795375553486));
#57485=CARTESIAN_POINT('Ctrl Pts',(1.75625188784759,-35.3280053709617,9.10111818708299));
#57486=CARTESIAN_POINT('Ctrl Pts',(1.69179021281346,-35.3288259503242,9.12309832361515));
#57487=CARTESIAN_POINT('Ctrl Pts',(1.62965570329652,-35.3295636157407,9.14252004395282));
#57488=CARTESIAN_POINT('Ctrl Pts',(1.57003931091995,-35.3302240353103,9.15976651693667));
#57489=CARTESIAN_POINT('Ctrl Pts',(1.5279546430745,-35.3306902416191,9.17194122355841));
#57490=CARTESIAN_POINT('Ctrl Pts',(1.48712382691784,-35.3311180448658,9.18303150086806));
#57491=CARTESIAN_POINT('Ctrl Pts',(1.44760068982356,-35.3315103566297,9.19316480258379));
#57492=CARTESIAN_POINT('Ctrl Pts',(1.42783912127643,-35.3317065125117,9.19823145344166));
#57493=CARTESIAN_POINT('Ctrl Pts',(1.40840430687648,-35.331893805453,9.20305875978609));
#57494=CARTESIAN_POINT('Ctrl Pts',(1.38930206702301,-35.332072648973,9.20766201286909));
#57495=CARTESIAN_POINT('Ctrl Pts',(1.37975094709627,-35.332162070733,9.20996363941059));
#57496=CARTESIAN_POINT('Ctrl Pts',(1.37028296542892,-35.3322493805427,9.21220924488872));
#57497=CARTESIAN_POINT('Ctrl Pts',(1.36089878598297,-35.3323346325335,9.21440070110702));
#57498=CARTESIAN_POINT('Ctrl Pts',(1.35855274112149,-35.3323559455312,9.2149485651616));
#57499=CARTESIAN_POINT('Ctrl Pts',(1.3562119338634,-35.3323771299207,9.21549304471547));
#57500=CARTESIAN_POINT('Ctrl Pts',(1.3538763743911,-35.3323981865595,9.21603416870073));
#57501=CARTESIAN_POINT('Ctrl Pts',(1.35212470478687,-35.3324139790386,9.21644001168968));
#57502=CARTESIAN_POINT('Ctrl Pts',(1.35037598705937,-35.332429699658,9.21684396716901));
#57503=CARTESIAN_POINT('Ctrl Pts',(1.34863022545477,-35.3324453487813,9.21724604730288));
#57504=CARTESIAN_POINT('Ctrl Pts',(1.34825195219046,-35.3324487396481,9.21733317040397));
#57505=CARTESIAN_POINT('Ctrl Pts',(1.34787429415118,-35.3324521228457,9.21742009462205));
#57506=CARTESIAN_POINT('Ctrl Pts',(1.34750862334315,-35.3324553967057,9.21750420799601));
#57507=CARTESIAN_POINT('Ctrl Pts',(1.34322339306478,-35.332493762481,9.21848991746203));
#57508=CARTESIAN_POINT('Ctrl Pts',(1.3401117239812,-35.3325214994015,9.2192024335089));
#57509=CARTESIAN_POINT('Ctrl Pts',(1.33464358697006,-35.3325697621369,9.2204418813168));
#57510=CARTESIAN_POINT('Ctrl Pts',(1.33411798538048,-35.3325744011886,9.22056101800571));
#57511=CARTESIAN_POINT('Ctrl Pts',(1.33357060365973,-35.3325792284085,9.22068498414979));
#57512=CARTESIAN_POINT('Ctrl Pts',(1.33299830070387,-35.3325842703551,9.22081446104479));
#57513=CARTESIAN_POINT('Ctrl Pts',(1.22309618033819,-35.3335524998829,9.24567853898191));
#57514=CARTESIAN_POINT('Ctrl Pts',(1.11238400514564,-35.3343710619394,9.26599310258083));
#57515=CARTESIAN_POINT('Ctrl Pts',(1.0012607468286,-35.3350043564305,9.28172514514179));
#57516=CARTESIAN_POINT('Ctrl Pts',(0.892850208941656,-35.3356221910536,
9.29707313998935));
#57517=CARTESIAN_POINT('Ctrl Pts',(0.784048819329241,-35.3360637385827,
9.3080595459942));
#57518=CARTESIAN_POINT('Ctrl Pts',(0.675207822854559,-35.3363181886785,
9.31469184807216));
#57519=CARTESIAN_POINT('Ctrl Pts',(0.568801182897241,-35.3365669476995,
9.32117581093685));
#57520=CARTESIAN_POINT('Ctrl Pts',(0.462357137263987,-35.3366369812772,
9.32349823724202));
#57521=CARTESIAN_POINT('Ctrl Pts',(0.356179114394229,-35.3365386439424,
9.32170372792902));
#57522=CARTESIAN_POINT('Ctrl Pts',(0.253833191420349,-35.3364438557272,
9.31997398473961));
#57523=CARTESIAN_POINT('Ctrl Pts',(0.151734892334258,-35.3361927823853,
9.31441921880504));
#57524=CARTESIAN_POINT('Ctrl Pts',(0.0501262832644089,-35.3358120216967,
9.30511395701379));
#57525=CARTESIAN_POINT('Ctrl Pts',(0.0334043515955558,-35.3357493591499,
9.3035825715017));
#57526=CARTESIAN_POINT('Ctrl Pts',(0.0166956057676047,-35.3356832206361,
9.30194968430529));
#57527=CARTESIAN_POINT('Ctrl Pts',(1.02886205599617E-6,-35.3356137675225,
9.30021571864812));
#57528=CARTESIAN_POINT('Ctrl Pts',(-2.60523473148,-35.3742356128,8.65541043601));
#57529=CARTESIAN_POINT('Ctrl Pts',(-2.76838711967,-34.7942356128,8.92400932641));
#57530=CARTESIAN_POINT('Ctrl Pts',(-2.93016897988,-34.2142356128,9.19332068473));
#57531=CARTESIAN_POINT('Ctrl Pts',(-3.09077135202,-33.6342356128,9.46303508034));
#57532=CARTESIAN_POINT('Ctrl Pts',(-3.25037602177,-33.0542356128,9.73294848656));
#57533=CARTESIAN_POINT('Ctrl Pts',(-3.40914395912,-32.4742356128,10.0029291615));
#57534=CARTESIAN_POINT('Ctrl Pts',(-2.08749540657,-35.3742356128,8.79956130216));
#57535=CARTESIAN_POINT('Ctrl Pts',(-2.20333316497,-34.7942356128,9.04664158555));
#57536=CARTESIAN_POINT('Ctrl Pts',(-2.31825723806,-34.2142356128,9.29419684756));
#57537=CARTESIAN_POINT('Ctrl Pts',(-2.43239498576,-33.6342356128,9.5420208011));
#57538=CARTESIAN_POINT('Ctrl Pts',(-2.54586759853,-33.0542356128,9.78997742837));
#57539=CARTESIAN_POINT('Ctrl Pts',(-2.6587823897,-32.4742356128,10.0379789015));
#57540=CARTESIAN_POINT('Ctrl Pts',(-1.56975608167,-35.3742356128,8.94371216831));
#57541=CARTESIAN_POINT('Ctrl Pts',(-1.63827921028,-34.7942356128,9.1692738447));
#57542=CARTESIAN_POINT('Ctrl Pts',(-1.70634549623,-34.2142356128,9.39507301039));
#57543=CARTESIAN_POINT('Ctrl Pts',(-1.77401861949,-33.6342356128,9.62100652185));
#57544=CARTESIAN_POINT('Ctrl Pts',(-1.84135917528,-33.0542356128,9.84700637017));
#57545=CARTESIAN_POINT('Ctrl Pts',(-1.90842082028,-32.4742356128,10.0730286414));
#57546=CARTESIAN_POINT('Ctrl Pts',(-1.05201675677,-35.3742356128,9.08786303446));
#57547=CARTESIAN_POINT('Ctrl Pts',(-1.07322525559,-34.7942356128,9.29190610384));
#57548=CARTESIAN_POINT('Ctrl Pts',(-1.09443375441,-34.2142356128,9.49594917322));
#57549=CARTESIAN_POINT('Ctrl Pts',(-1.11564225322,-33.6342356128,9.6999922426));
#57550=CARTESIAN_POINT('Ctrl Pts',(-1.13685075204,-33.0542356128,9.90403531198));
#57551=CARTESIAN_POINT('Ctrl Pts',(-1.15805925086,-32.4742356128,10.1080783814));
#57552=CARTESIAN_POINT('Ctrl Pts',(0.511836420903,-35.3742356128,9.5232767248));
#57553=CARTESIAN_POINT('Ctrl Pts',(0.628849173616,-34.7942356128,9.66130309814));
#57554=CARTESIAN_POINT('Ctrl Pts',(0.745861926328,-34.2142356128,9.79932947148));
#57555=CARTESIAN_POINT('Ctrl Pts',(0.862874679041,-33.6342356128,9.93735584482));
#57556=CARTESIAN_POINT('Ctrl Pts',(0.979887431754,-33.0542356128,10.0753822182));
#57557=CARTESIAN_POINT('Ctrl Pts',(1.09690018447,-32.4742356128,10.2134085915));
#57558=CARTESIAN_POINT('Ctrl Pts',(2.16072134347,-35.3742356128,9.16274026182));
#57559=CARTESIAN_POINT('Ctrl Pts',(2.3948826075,-34.7942356128,9.28181994923));
#57560=CARTESIAN_POINT('Ctrl Pts',(2.62904387153,-34.2142356128,9.40089963664));
#57561=CARTESIAN_POINT('Ctrl Pts',(2.86320513556,-33.6342356128,9.51997932405));
#57562=CARTESIAN_POINT('Ctrl Pts',(3.09736639959,-33.0542356128,9.63905901146));
#57563=CARTESIAN_POINT('Ctrl Pts',(3.33152766362,-32.4742356128,9.75813869887));
#57564=CARTESIAN_POINT('Ctrl Pts',(3.13619409311,-35.3742356128,8.55164595878));
#57565=CARTESIAN_POINT('Ctrl Pts',(3.45938700394,-34.7942356128,8.6832339856));
#57566=CARTESIAN_POINT('Ctrl Pts',(3.78257991477,-34.2142356128,8.81482201242));
#57567=CARTESIAN_POINT('Ctrl Pts',(4.1057728256,-33.6342356128,8.94641003924));
#57568=CARTESIAN_POINT('Ctrl Pts',(4.42896573643,-33.0542356128,9.07799806607));
#57569=CARTESIAN_POINT('Ctrl Pts',(4.75215864726,-32.4742356128,9.20958609289));
#57570=CARTESIAN_POINT('Ctrl Pts',(3.83208911107,-35.3742356128,7.6674137228));
#57571=CARTESIAN_POINT('Ctrl Pts',(4.27752956283,-34.7942356128,7.82055675035));
#57572=CARTESIAN_POINT('Ctrl Pts',(4.7229700146,-34.2142356128,7.97369977791));
#57573=CARTESIAN_POINT('Ctrl Pts',(5.16841046636,-33.6342356128,8.12684280547));
#57574=CARTESIAN_POINT('Ctrl Pts',(5.61385091813,-33.0542356128,8.27998583302));
#57575=CARTESIAN_POINT('Ctrl Pts',(6.05929136989,-32.4742356128,8.43312886058));
#57576=CARTESIAN_POINT('Ctrl Pts',(4.19318797439,-35.3742356128,6.66283715371));
#57577=CARTESIAN_POINT('Ctrl Pts',(4.79568377915,-34.7942356128,6.82348987203));
#57578=CARTESIAN_POINT('Ctrl Pts',(5.3981795839,-34.2142356128,6.98414259034));
#57579=CARTESIAN_POINT('Ctrl Pts',(6.00067538866,-33.6342356128,7.14479530865));
#57580=CARTESIAN_POINT('Ctrl Pts',(6.60317119342,-33.0542356128,7.30544802697));
#57581=CARTESIAN_POINT('Ctrl Pts',(7.20566699818,-32.4742356128,7.46610074528));
#57582=CARTESIAN_POINT('',(-1.71543475557812E-5,-32.7425794170381,10.0435077220134));
#57583=CARTESIAN_POINT('Ctrl Pts',(6.71017463815815E-10,-35.3356164375956,
9.30022551106375));
#57584=CARTESIAN_POINT('Ctrl Pts',(9.35141029305416E-9,-35.1420353216907,
9.35303380178583));
#57585=CARTESIAN_POINT('Ctrl Pts',(-5.65694962445924E-5,-34.9391902220334,
9.40909973890534));
#57586=CARTESIAN_POINT('Ctrl Pts',(-0.000103461444640018,-34.72708113854,
9.46852350682398));
#57587=CARTESIAN_POINT('Ctrl Pts',(-0.000150448019398666,-34.514544026102,
9.52806718989308));
#57588=CARTESIAN_POINT('Ctrl Pts',(-0.000187656962521676,-34.2927055032922,
9.59098216616354));
#57589=CARTESIAN_POINT('Ctrl Pts',(-0.000191091383847208,-34.0615655700265,
9.6573387038564));
#57590=CARTESIAN_POINT('Ctrl Pts',(-0.000194539831505515,-33.8294816507689,
9.72396624466482));
#57591=CARTESIAN_POINT('Ctrl Pts',(-0.000163896434727065,-33.5880201911472,
9.79406343861578));
#57592=CARTESIAN_POINT('Ctrl Pts',(-0.000118572553254648,-33.337181191076,
9.86767201279748));
#57593=CARTESIAN_POINT('Ctrl Pts',(-8.37595163062467E-5,-33.1445130635043,
9.92421037468217));
#57594=CARTESIAN_POINT('Ctrl Pts',(-4.11726282365265E-5,-32.9463124721712,
9.98281974137946));
#57595=CARTESIAN_POINT('Ctrl Pts',(-1.71543475557812E-5,-32.7425794170381,
10.0435077220134));
#57596=CARTESIAN_POINT('',(-7.77156117238E-15,-32.4742356128,10.1236848855));
#57597=CARTESIAN_POINT('Ctrl Pts',(-1.71543475557812E-5,-32.7425794170381,
10.0435077220134));
#57598=CARTESIAN_POINT('Ctrl Pts',(-6.73205891155968E-6,-32.6541732261376,
10.0698421486866));
#57599=CARTESIAN_POINT('Ctrl Pts',(5.83743083992971E-14,-32.5647252913926,
10.0965678485074));
#57600=CARTESIAN_POINT('Ctrl Pts',(8.39328606616618E-14,-32.4742356128,
10.1236848854971));
#57601=CARTESIAN_POINT('',(7.20566699818,-32.4742356128,7.46610074528));
#57602=CARTESIAN_POINT('Ctrl Pts',(-7.77156117238E-15,-32.4742356128,10.1236848855));
#57603=CARTESIAN_POINT('Ctrl Pts',(0.0686255073634253,-32.4742356128,10.1230144724525));
#57604=CARTESIAN_POINT('Ctrl Pts',(0.137239296162275,-32.4742356128,10.1219531731961));
#57605=CARTESIAN_POINT('Ctrl Pts',(0.205839273380599,-32.4742356128,10.1204615805581));
#57606=CARTESIAN_POINT('Ctrl Pts',(1.77362452481901,-32.4742356128,10.0755367445611));
#57607=CARTESIAN_POINT('Ctrl Pts',(3.33152766362,-32.4742356128,9.75813869887));
#57608=CARTESIAN_POINT('Ctrl Pts',(4.75215864726,-32.4742356128,9.20958609289));
#57609=CARTESIAN_POINT('Ctrl Pts',(6.05929136989,-32.4742356128,8.43312886058));
#57610=CARTESIAN_POINT('Ctrl Pts',(7.20566699818,-32.4742356128,7.46610074528));
#57611=CARTESIAN_POINT('',(4.2854138145,-35.285453273,6.68742874721));
#57612=CARTESIAN_POINT('Ctrl Pts',(2.60523473148,-35.3742356128,8.65541043601));
#57613=CARTESIAN_POINT('Ctrl Pts',(2.76838711967,-34.7942356128,8.92400932641));
#57614=CARTESIAN_POINT('Ctrl Pts',(2.93016897988,-34.2142356128,9.19332068473));
#57615=CARTESIAN_POINT('Ctrl Pts',(3.09077135202,-33.6342356128,9.46303508034));
#57616=CARTESIAN_POINT('Ctrl Pts',(3.25037602177,-33.0542356128,9.73294848656));
#57617=CARTESIAN_POINT('Ctrl Pts',(3.40914395912,-32.4742356128,10.0029291615));
#57618=CARTESIAN_POINT('Ctrl Pts',(2.08749540657,-35.3742356128,8.79956130216));
#57619=CARTESIAN_POINT('Ctrl Pts',(2.20333316497,-34.7942356128,9.04664158555));
#57620=CARTESIAN_POINT('Ctrl Pts',(2.31825723806,-34.2142356128,9.29419684756));
#57621=CARTESIAN_POINT('Ctrl Pts',(2.43239498576,-33.6342356128,9.5420208011));
#57622=CARTESIAN_POINT('Ctrl Pts',(2.54586759853,-33.0542356128,9.78997742837));
#57623=CARTESIAN_POINT('Ctrl Pts',(2.6587823897,-32.4742356128,10.0379789015));
#57624=CARTESIAN_POINT('Ctrl Pts',(1.56975608167,-35.3742356128,8.94371216831));
#57625=CARTESIAN_POINT('Ctrl Pts',(1.63827921028,-34.7942356128,9.1692738447));
#57626=CARTESIAN_POINT('Ctrl Pts',(1.70634549623,-34.2142356128,9.39507301039));
#57627=CARTESIAN_POINT('Ctrl Pts',(1.77401861949,-33.6342356128,9.62100652185));
#57628=CARTESIAN_POINT('Ctrl Pts',(1.84135917528,-33.0542356128,9.84700637017));
#57629=CARTESIAN_POINT('Ctrl Pts',(1.90842082028,-32.4742356128,10.0730286414));
#57630=CARTESIAN_POINT('Ctrl Pts',(1.05201675677,-35.3742356128,9.08786303446));
#57631=CARTESIAN_POINT('Ctrl Pts',(1.07322525559,-34.7942356128,9.29190610384));
#57632=CARTESIAN_POINT('Ctrl Pts',(1.09443375441,-34.2142356128,9.49594917322));
#57633=CARTESIAN_POINT('Ctrl Pts',(1.11564225322,-33.6342356128,9.6999922426));
#57634=CARTESIAN_POINT('Ctrl Pts',(1.13685075204,-33.0542356128,9.90403531198));
#57635=CARTESIAN_POINT('Ctrl Pts',(1.15805925086,-32.4742356128,10.1080783814));
#57636=CARTESIAN_POINT('Ctrl Pts',(-0.511836420903,-35.3742356128,9.5232767248));
#57637=CARTESIAN_POINT('Ctrl Pts',(-0.628849173616,-34.7942356128,9.66130309814));
#57638=CARTESIAN_POINT('Ctrl Pts',(-0.745861926328,-34.2142356128,9.79932947148));
#57639=CARTESIAN_POINT('Ctrl Pts',(-0.862874679041,-33.6342356128,9.93735584482));
#57640=CARTESIAN_POINT('Ctrl Pts',(-0.979887431754,-33.0542356128,10.0753822182));
#57641=CARTESIAN_POINT('Ctrl Pts',(-1.09690018447,-32.4742356128,10.2134085915));
#57642=CARTESIAN_POINT('Ctrl Pts',(-2.16072134347,-35.3742356128,9.16274026182));
#57643=CARTESIAN_POINT('Ctrl Pts',(-2.3948826075,-34.7942356128,9.28181994923));
#57644=CARTESIAN_POINT('Ctrl Pts',(-2.62904387153,-34.2142356128,9.40089963664));
#57645=CARTESIAN_POINT('Ctrl Pts',(-2.86320513556,-33.6342356128,9.51997932405));
#57646=CARTESIAN_POINT('Ctrl Pts',(-3.09736639959,-33.0542356128,9.63905901146));
#57647=CARTESIAN_POINT('Ctrl Pts',(-3.33152766362,-32.4742356128,9.75813869887));
#57648=CARTESIAN_POINT('Ctrl Pts',(-3.13619409311,-35.3742356128,8.55164595878));
#57649=CARTESIAN_POINT('Ctrl Pts',(-3.45938700394,-34.7942356128,8.6832339856));
#57650=CARTESIAN_POINT('Ctrl Pts',(-3.78257991477,-34.2142356128,8.81482201242));
#57651=CARTESIAN_POINT('Ctrl Pts',(-4.1057728256,-33.6342356128,8.94641003924));
#57652=CARTESIAN_POINT('Ctrl Pts',(-4.42896573643,-33.0542356128,9.07799806607));
#57653=CARTESIAN_POINT('Ctrl Pts',(-4.75215864726,-32.4742356128,9.20958609289));
#57654=CARTESIAN_POINT('Ctrl Pts',(-3.83208911107,-35.3742356128,7.6674137228));
#57655=CARTESIAN_POINT('Ctrl Pts',(-4.27752956283,-34.7942356128,7.82055675035));
#57656=CARTESIAN_POINT('Ctrl Pts',(-4.7229700146,-34.2142356128,7.97369977791));
#57657=CARTESIAN_POINT('Ctrl Pts',(-5.16841046636,-33.6342356128,8.12684280547));
#57658=CARTESIAN_POINT('Ctrl Pts',(-5.61385091813,-33.0542356128,8.27998583302));
#57659=CARTESIAN_POINT('Ctrl Pts',(-6.05929136989,-32.4742356128,8.43312886058));
#57660=CARTESIAN_POINT('Ctrl Pts',(-4.19318797439,-35.3742356128,6.66283715371));
#57661=CARTESIAN_POINT('Ctrl Pts',(-4.79568377915,-34.7942356128,6.82348987203));
#57662=CARTESIAN_POINT('Ctrl Pts',(-5.3981795839,-34.2142356128,6.98414259034));
#57663=CARTESIAN_POINT('Ctrl Pts',(-6.00067538866,-33.6342356128,7.14479530865));
#57664=CARTESIAN_POINT('Ctrl Pts',(-6.60317119342,-33.0542356128,7.30544802697));
#57665=CARTESIAN_POINT('Ctrl Pts',(-7.20566699818,-32.4742356128,7.46610074528));
#57666=CARTESIAN_POINT('',(-7.20566699818,-32.4742356128,7.46610074528));
#57667=CARTESIAN_POINT('',(-4.2854138145,-35.285453273,6.68742874721));
#57668=CARTESIAN_POINT('Ctrl Pts',(2.05391259555654E-14,-32.4742356128,
10.1236848854971));
#57669=CARTESIAN_POINT('Ctrl Pts',(-0.723226925025329,-32.4742356128,10.1166195707796));
#57670=CARTESIAN_POINT('Ctrl Pts',(-2.22086602908888,-32.4742356128001,
10.0501259104731));
#57671=CARTESIAN_POINT('Ctrl Pts',(-5.15748989495571,-32.4742356128001,
8.91985491792444));
#57672=CARTESIAN_POINT('Ctrl Pts',(-6.24653783595315,-32.4742356128,8.27517662162345));
#57673=CARTESIAN_POINT('Ctrl Pts',(-7.20566699818,-32.4742356128,7.46610074528));
#57674=CARTESIAN_POINT('Ctrl Pts',(-4.19318797439,-35.3742356128,6.66283715371));
#57675=CARTESIAN_POINT('Ctrl Pts',(-7.20566699818,-32.4742356128,7.46610074528));
#57676=CARTESIAN_POINT('Ctrl Pts',(-4.25225922259,-35.3742356128,6.49850101766));
#57677=CARTESIAN_POINT('Ctrl Pts',(-7.39320029639,-32.4742356128,7.30790654658));
#57678=CARTESIAN_POINT('Ctrl Pts',(-4.30237103799,-35.3742356128,6.33094436873));
#57679=CARTESIAN_POINT('Ctrl Pts',(-7.53221837753,-32.4742356128,7.09219938589));
#57680=CARTESIAN_POINT('Ctrl Pts',(-4.34319574155,-35.3742356128,6.16124819217));
#57681=CARTESIAN_POINT('Ctrl Pts',(-7.59868325739,-32.4742356128,6.83930575178));
#57682=CARTESIAN_POINT('Ctrl Pts',(-4.37477641654,-35.3742356128,5.98923343741));
#57683=CARTESIAN_POINT('Ctrl Pts',(-7.58368665883,-32.4742356128,6.58312083129));
#57684=CARTESIAN_POINT('Ctrl Pts',(-4.3969132289,-35.3742356128,5.81601178901));
#57685=CARTESIAN_POINT('Ctrl Pts',(-7.49816640227,-32.4742356128,6.35316338263));
#57686=CARTESIAN_POINT('',(-7.49816640227,-32.4742356128,6.35316338263));
#57687=CARTESIAN_POINT('',(-4.49212120371,-35.2852060782,5.83250225674));
#57688=CARTESIAN_POINT('Origin',(-6.56088648981501,-32.4742356127961,6.70173548960406));
#57689=CARTESIAN_POINT('Ctrl Pts',(-4.3969132289,-35.3742356128,5.81601178901));
#57690=CARTESIAN_POINT('Ctrl Pts',(-7.49816640227,-32.4742356128,6.35316338263));
#57691=CARTESIAN_POINT('Ctrl Pts',(-4.48962392508,-35.3742356128,5.0905460197));
#57692=CARTESIAN_POINT('Ctrl Pts',(-7.14000207598,-32.4742356128,5.39008683572));
#57693=CARTESIAN_POINT('Ctrl Pts',(-4.41668920588,-35.3742356128,4.34391151104));
#57694=CARTESIAN_POINT('Ctrl Pts',(-6.73176998559,-32.4742356128,4.44563102148));
#57695=CARTESIAN_POINT('Ctrl Pts',(-4.17142295951,-35.3742356128,3.62676818174));
#57696=CARTESIAN_POINT('Ctrl Pts',(-6.27486238853,-32.4742356128,3.52346144896));
#57697=CARTESIAN_POINT('Ctrl Pts',(-3.771858743,-35.3742356128,2.99184297704));
#57698=CARTESIAN_POINT('Ctrl Pts',(-5.77073547798,-32.4742356128,2.62651750489));
#57699=CARTESIAN_POINT('Ctrl Pts',(-3.25430421882,-35.3742356128,2.47509045608));
#57700=CARTESIAN_POINT('Ctrl Pts',(-5.22146332445,-32.4742356128,1.7581292142));
#57701=CARTESIAN_POINT('',(-5.22146332445,-32.4742356128,1.7581292142));
#57702=CARTESIAN_POINT('',(-3.30528109741,-35.2990851344,2.45651115251));
#57703=CARTESIAN_POINT('Origin',(15.657527533216,-32.4742356128,14.9645861152497));
#57704=CARTESIAN_POINT('Ctrl Pts',(-3.25430421882,-35.3742356128,2.47509045608));
#57705=CARTESIAN_POINT('Ctrl Pts',(-5.22146332445,-32.4742356128,1.7581292142));
#57706=CARTESIAN_POINT('Ctrl Pts',(-3.2239318541,-35.3742356128,2.44476515183));
#57707=CARTESIAN_POINT('Ctrl Pts',(-5.1892302237,-32.4742356128,1.70716932646));
#57708=CARTESIAN_POINT('Ctrl Pts',(-3.19898265017,-35.3742356128,2.40900827334));
#57709=CARTESIAN_POINT('Ctrl Pts',(-5.15684165406,-32.4742356128,1.65630777433));
#57710=CARTESIAN_POINT('Ctrl Pts',(-3.18021147649,-35.3742356128,2.36763482469));
#57711=CARTESIAN_POINT('Ctrl Pts',(-5.1231181514,-32.4742356128,1.60370991526));
#57712=CARTESIAN_POINT('Ctrl Pts',(-3.16973557012,-35.3742356128,2.32531139715));
#57713=CARTESIAN_POINT('Ctrl Pts',(-5.09041537382,-32.4742356128,1.55304981975));
#57714=CARTESIAN_POINT('Ctrl Pts',(-3.16691857253,-35.3742356128,2.28248419619));
#57715=CARTESIAN_POINT('Ctrl Pts',(-5.05755834899,-32.4742356128,1.50248996551));
#57716=CARTESIAN_POINT('',(-5.05755834899,-32.4742356128,1.50248996551));
#57717=CARTESIAN_POINT('',(-3.2167330984,-35.297826491,2.26193292922));
#57718=CARTESIAN_POINT('Origin',(15.7711771435274,-32.4742356128,15.0373502450657));
#57719=CARTESIAN_POINT('Ctrl Pts',(-3.16691857253,-35.3742356128,2.28248419619));
#57720=CARTESIAN_POINT('Ctrl Pts',(-5.05755834899,-32.4742356128,1.50248996551));
#57721=CARTESIAN_POINT('Ctrl Pts',(-3.14279442744,-35.3742356128,1.91572108521));
#57722=CARTESIAN_POINT('Ctrl Pts',(-4.77617249442,-32.4742356128,1.06949799882));
#57723=CARTESIAN_POINT('Ctrl Pts',(-3.11867028235,-35.3742356128,1.54895799245));
#57724=CARTESIAN_POINT('Ctrl Pts',(-4.48347398519,-32.4742356128,0.643857892919));
#57725=CARTESIAN_POINT('Ctrl Pts',(-3.09450967796,-35.3742356128,1.18164054895));
#57726=CARTESIAN_POINT('Ctrl Pts',(-4.17925298698,-32.4742356128,0.225336592507));
#57727=CARTESIAN_POINT('Ctrl Pts',(-3.07038553283,-35.3742356128,0.814877455407));
#57728=CARTESIAN_POINT('Ctrl Pts',(-3.86470492801,-32.4742356128,-0.184421152381));
#57729=CARTESIAN_POINT('Ctrl Pts',(-3.0462613877,-35.3742356128,0.448114344193));
#57730=CARTESIAN_POINT('Ctrl Pts',(-3.53967296235,-32.4742356128,-0.585686978861));
#57731=CARTESIAN_POINT('',(-3.53967296235,-32.4742356128,-0.585686978861));
#57732=CARTESIAN_POINT('',(-3.05109044571,-35.345853084,0.437996449075));
#57733=CARTESIAN_POINT('Ctrl Pts',(-3.53967296235,-32.4742356128,-0.585686978860996));
#57734=CARTESIAN_POINT('Ctrl Pts',(-3.81069940134122,-32.4742356128,-0.251093278764725));
#57735=CARTESIAN_POINT('Ctrl Pts',(-4.07285675309246,-32.4742356128,0.0904475661883553));
#57736=CARTESIAN_POINT('Ctrl Pts',(-4.57894874401687,-32.4742356128,0.786685671920166));
#57737=CARTESIAN_POINT('Ctrl Pts',(-4.8229261644615,-32.4742356128,1.14144178423942));
#57738=CARTESIAN_POINT('Ctrl Pts',(-5.05755834899,-32.4742356128,1.50248996551));
#57739=CARTESIAN_POINT('Ctrl Pts',(-3.0462613877,-35.3742356128,0.448114344193));
#57740=CARTESIAN_POINT('Ctrl Pts',(-3.53967296235,-32.4742356128,-0.585686978861));
#57741=CARTESIAN_POINT('Ctrl Pts',(-3.04377855919,-35.3742356128,0.410367561768));
#57742=CARTESIAN_POINT('Ctrl Pts',(-3.50622171659,-32.4742356128,-0.626983968707));
#57743=CARTESIAN_POINT('Ctrl Pts',(-3.03534613584,-35.3742356128,0.373012120652));
#57744=CARTESIAN_POINT('Ctrl Pts',(-3.4726594259,-32.4742356128,-0.668191011718));
#57745=CARTESIAN_POINT('Ctrl Pts',(-3.02058192311,-35.3742356128,0.336333109732));
#57746=CARTESIAN_POINT('Ctrl Pts',(-3.4380400694,-32.4742356128,-0.710460650811));
#57747=CARTESIAN_POINT('Ctrl Pts',(-3.00078302788,-35.3742356128,0.30355295586));
#57748=CARTESIAN_POINT('Ctrl Pts',(-3.40425418736,-32.4742356128,-0.75148456633));
#57749=CARTESIAN_POINT('Ctrl Pts',(-2.97642257165,-35.3742356128,0.274612461872));
#57750=CARTESIAN_POINT('Ctrl Pts',(-3.37035823989,-32.4742356128,-0.792417339984));
#57751=CARTESIAN_POINT('',(-3.37035823989,-32.4742356128,-0.792417339984));
#57752=CARTESIAN_POINT('',(-2.98281092224,-35.3272070795,0.257308721649));
#57753=CARTESIAN_POINT('Origin',(-3.43621138602758,-32.4742356128,-0.673649465592228));
#57754=CARTESIAN_POINT('Ctrl Pts',(-2.97642257165,-35.3742356128,0.274612461872));
#57755=CARTESIAN_POINT('Ctrl Pts',(-3.37035823989,-32.4742356128,-0.792417339984));
#57756=CARTESIAN_POINT('Ctrl Pts',(-2.53990923767,-35.3742356128,-0.243970172904));
#57757=CARTESIAN_POINT('Ctrl Pts',(-2.76296793319,-32.4742356128,-1.52590236845));
#57758=CARTESIAN_POINT('Ctrl Pts',(-1.99045494271,-35.3742356128,-0.667485652616));
#57759=CARTESIAN_POINT('Ctrl Pts',(-2.12023572482,-32.4742356128,-2.23012174203));
#57760=CARTESIAN_POINT('Ctrl Pts',(-1.35568684616,-35.3742356128,-0.962884347862));
#57761=CARTESIAN_POINT('Ctrl Pts',(-1.44418220412,-32.4742356128,-2.90267037222));
#57762=CARTESIAN_POINT('Ctrl Pts',(-0.677843520645,-35.3742356128,-1.11051031269));
#57763=CARTESIAN_POINT('Ctrl Pts',(-0.736632181986,-32.4742356128,-3.54173296481));
#57764=CARTESIAN_POINT('Ctrl Pts',(-3.34917279095E-15,-35.3742356128,-1.11051031258));
#57765=CARTESIAN_POINT('Ctrl Pts',(-1.48930250848E-13,-32.4742356128,-4.14530259747));
#57766=CARTESIAN_POINT('',(-1.487698853E-13,-32.4742356128,-4.14530259747));
#57767=CARTESIAN_POINT('',(-7.77156117238E-15,-35.2855840756,-1.20328238204));
#57768=CARTESIAN_POINT('Origin',(15.6577121383952,-32.4742356128,14.9644107719153));
#57769=CARTESIAN_POINT('Ctrl Pts',(2.97642257165,-35.3742356128,0.274612461872));
#57770=CARTESIAN_POINT('Ctrl Pts',(3.37035823989,-32.4742356128,-0.792417339984));
#57771=CARTESIAN_POINT('Ctrl Pts',(2.53990923767,-35.3742356128,-0.243970172904));
#57772=CARTESIAN_POINT('Ctrl Pts',(2.76296793319,-32.4742356128,-1.52590236845));
#57773=CARTESIAN_POINT('Ctrl Pts',(1.99045494271,-35.3742356128,-0.667485652616));
#57774=CARTESIAN_POINT('Ctrl Pts',(2.12023572482,-32.4742356128,-2.23012174203));
#57775=CARTESIAN_POINT('Ctrl Pts',(1.35568684616,-35.3742356128,-0.962884347862));
#57776=CARTESIAN_POINT('Ctrl Pts',(1.44418220412,-32.4742356128,-2.90267037222));
#57777=CARTESIAN_POINT('Ctrl Pts',(0.677843520645,-35.3742356128,-1.11051031269));
#57778=CARTESIAN_POINT('Ctrl Pts',(0.736632181986,-32.4742356128,-3.54173296481));
#57779=CARTESIAN_POINT('Ctrl Pts',(1.42787016778E-15,-35.3742356128,-1.11051031258));
#57780=CARTESIAN_POINT('Ctrl Pts',(1.50638760725E-13,-32.4742356128,-4.14530259747));
#57781=CARTESIAN_POINT('',(3.37035823989,-32.4742356128,-0.792417339984));
#57782=CARTESIAN_POINT('',(2.98281092222467,-35.3272070794932,0.257308721661903));
#57783=CARTESIAN_POINT('Origin',(-15.6577121383927,-32.4742356127996,14.9644107719132));
#57784=CARTESIAN_POINT('Ctrl Pts',(3.0462613877,-35.3742356128,0.448114344193));
#57785=CARTESIAN_POINT('Ctrl Pts',(3.53967296235,-32.4742356128,-0.585686978861));
#57786=CARTESIAN_POINT('Ctrl Pts',(3.04377855919,-35.3742356128,0.410367561768));
#57787=CARTESIAN_POINT('Ctrl Pts',(3.50622171659,-32.4742356128,-0.626983968707));
#57788=CARTESIAN_POINT('Ctrl Pts',(3.03534613584,-35.3742356128,0.373012120652));
#57789=CARTESIAN_POINT('Ctrl Pts',(3.4726594259,-32.4742356128,-0.668191011718));
#57790=CARTESIAN_POINT('Ctrl Pts',(3.02058192311,-35.3742356128,0.336333109732));
#57791=CARTESIAN_POINT('Ctrl Pts',(3.4380400694,-32.4742356128,-0.710460650811));
#57792=CARTESIAN_POINT('Ctrl Pts',(3.00078302788,-35.3742356128,0.30355295586));
#57793=CARTESIAN_POINT('Ctrl Pts',(3.40425418736,-32.4742356128,-0.75148456633));
#57794=CARTESIAN_POINT('Ctrl Pts',(2.97642257165,-35.3742356128,0.274612461872));
#57795=CARTESIAN_POINT('Ctrl Pts',(3.37035823989,-32.4742356128,-0.792417339984));
#57796=CARTESIAN_POINT('',(3.53967296235,-32.4742356128,-0.585686978861));
#57797=CARTESIAN_POINT('',(3.05109044570917,-35.3458530839998,0.437996449075061));
#57798=CARTESIAN_POINT('Origin',(3.43621138602758,-32.4742356128,-0.673649465592228));
#57799=CARTESIAN_POINT('Ctrl Pts',(3.16691857253,-35.3742356128,2.28248419619));
#57800=CARTESIAN_POINT('Ctrl Pts',(5.05755834899,-32.4742356128,1.50248996551));
#57801=CARTESIAN_POINT('Ctrl Pts',(3.14279442744,-35.3742356128,1.91572108521));
#57802=CARTESIAN_POINT('Ctrl Pts',(4.77617249442,-32.4742356128,1.06949799882));
#57803=CARTESIAN_POINT('Ctrl Pts',(3.11867028235,-35.3742356128,1.54895799245));
#57804=CARTESIAN_POINT('Ctrl Pts',(4.48347398519,-32.4742356128,0.643857892919));
#57805=CARTESIAN_POINT('Ctrl Pts',(3.09450967796,-35.3742356128,1.18164054895));
#57806=CARTESIAN_POINT('Ctrl Pts',(4.17925298698,-32.4742356128,0.225336592507));
#57807=CARTESIAN_POINT('Ctrl Pts',(3.07038553283,-35.3742356128,0.814877455407));
#57808=CARTESIAN_POINT('Ctrl Pts',(3.86470492801,-32.4742356128,-0.184421152381));
#57809=CARTESIAN_POINT('Ctrl Pts',(3.0462613877,-35.3742356128,0.448114344193));
#57810=CARTESIAN_POINT('Ctrl Pts',(3.53967296235,-32.4742356128,-0.585686978861));
#57811=CARTESIAN_POINT('',(5.05755834899,-32.4742356128,1.50248996551));
#57812=CARTESIAN_POINT('',(3.21673309838426,-35.2978264909894,2.26193292922132));
#57813=CARTESIAN_POINT('Ctrl Pts',(3.53967296235,-32.4742356128,-0.585686978860997));
#57814=CARTESIAN_POINT('Ctrl Pts',(3.81069940134122,-32.4742356128,-0.251093278764735));
#57815=CARTESIAN_POINT('Ctrl Pts',(4.07285675309245,-32.4742356128,0.0904475661883362));
#57816=CARTESIAN_POINT('Ctrl Pts',(4.57894874401687,-32.4742356128,0.786685671920158));
#57817=CARTESIAN_POINT('Ctrl Pts',(4.8229261644615,-32.4742356128,1.14144178423942));
#57818=CARTESIAN_POINT('Ctrl Pts',(5.05755834899,-32.4742356128,1.50248996551));
#57819=CARTESIAN_POINT('Ctrl Pts',(3.25430421882,-35.3742356128,2.47509045608));
#57820=CARTESIAN_POINT('Ctrl Pts',(5.22146332445,-32.4742356128,1.7581292142));
#57821=CARTESIAN_POINT('Ctrl Pts',(3.2239318541,-35.3742356128,2.44476515183));
#57822=CARTESIAN_POINT('Ctrl Pts',(5.1892302237,-32.4742356128,1.70716932646));
#57823=CARTESIAN_POINT('Ctrl Pts',(3.19898265017,-35.3742356128,2.40900827334));
#57824=CARTESIAN_POINT('Ctrl Pts',(5.15684165406,-32.4742356128,1.65630777433));
#57825=CARTESIAN_POINT('Ctrl Pts',(3.18021147649,-35.3742356128,2.36763482469));
#57826=CARTESIAN_POINT('Ctrl Pts',(5.1231181514,-32.4742356128,1.60370991526));
#57827=CARTESIAN_POINT('Ctrl Pts',(3.16973557012,-35.3742356128,2.32531139715));
#57828=CARTESIAN_POINT('Ctrl Pts',(5.09041537382,-32.4742356128,1.55304981975));
#57829=CARTESIAN_POINT('Ctrl Pts',(3.16691857253,-35.3742356128,2.28248419619));
#57830=CARTESIAN_POINT('Ctrl Pts',(5.05755834899,-32.4742356128,1.50248996551));
#57831=CARTESIAN_POINT('',(5.22146332445,-32.4742356128,1.7581292142));
#57832=CARTESIAN_POINT('',(3.30528109740205,-35.2990851343927,2.45651115251783));
#57833=CARTESIAN_POINT('Origin',(-15.7711771435274,-32.4742356128,15.0373502450657));
#57834=CARTESIAN_POINT('Ctrl Pts',(4.3969132289,-35.3742356128,5.81601178901));
#57835=CARTESIAN_POINT('Ctrl Pts',(7.49816640227,-32.4742356128,6.35316338263));
#57836=CARTESIAN_POINT('Ctrl Pts',(4.48962392508,-35.3742356128,5.0905460197));
#57837=CARTESIAN_POINT('Ctrl Pts',(7.14000207598,-32.4742356128,5.39008683572));
#57838=CARTESIAN_POINT('Ctrl Pts',(4.41668920588,-35.3742356128,4.34391151104));
#57839=CARTESIAN_POINT('Ctrl Pts',(6.73176998559,-32.4742356128,4.44563102148));
#57840=CARTESIAN_POINT('Ctrl Pts',(4.17142295951,-35.3742356128,3.62676818174));
#57841=CARTESIAN_POINT('Ctrl Pts',(6.27486238853,-32.4742356128,3.52346144896));
#57842=CARTESIAN_POINT('Ctrl Pts',(3.771858743,-35.3742356128,2.99184297704));
#57843=CARTESIAN_POINT('Ctrl Pts',(5.77073547798,-32.4742356128,2.62651750489));
#57844=CARTESIAN_POINT('Ctrl Pts',(3.25430421882,-35.3742356128,2.47509045608));
#57845=CARTESIAN_POINT('Ctrl Pts',(5.22146332445,-32.4742356128,1.7581292142));
#57846=CARTESIAN_POINT('',(7.49816640227,-32.4742356128,6.35316338263));
#57847=CARTESIAN_POINT('',(4.49212120367077,-35.2852060781573,5.83250225673578));
#57848=CARTESIAN_POINT('Origin',(-15.657527533216,-32.4742356128,14.9645861152497));
#57849=CARTESIAN_POINT('Ctrl Pts',(4.19318797439,-35.3742356128,6.66283715371));
#57850=CARTESIAN_POINT('Ctrl Pts',(7.20566699818,-32.4742356128,7.46610074528));
#57851=CARTESIAN_POINT('Ctrl Pts',(4.25225922259,-35.3742356128,6.49850101766));
#57852=CARTESIAN_POINT('Ctrl Pts',(7.39320029639,-32.4742356128,7.30790654658));
#57853=CARTESIAN_POINT('Ctrl Pts',(4.30237103799,-35.3742356128,6.33094436873));
#57854=CARTESIAN_POINT('Ctrl Pts',(7.53221837753,-32.4742356128,7.09219938589));
#57855=CARTESIAN_POINT('Ctrl Pts',(4.34319574155,-35.3742356128,6.16124819217));
#57856=CARTESIAN_POINT('Ctrl Pts',(7.59868325739,-32.4742356128,6.83930575178));
#57857=CARTESIAN_POINT('Ctrl Pts',(4.37477641654,-35.3742356128,5.98923343741));
#57858=CARTESIAN_POINT('Ctrl Pts',(7.58368665883,-32.4742356128,6.58312083129));
#57859=CARTESIAN_POINT('Ctrl Pts',(4.3969132289,-35.3742356128,5.81601178901));
#57860=CARTESIAN_POINT('Ctrl Pts',(7.49816640227,-32.4742356128,6.35316338263));
#57861=CARTESIAN_POINT('Origin',(6.56088648981501,-32.4742356127961,6.70173548960406));
#57862=CARTESIAN_POINT('Origin',(-6.22337865086E-16,-32.4742356128,0.));
#57863=CARTESIAN_POINT('',(-1.27198391691,-32.4742356128,-10.1164167671));
#57864=CARTESIAN_POINT('',(1.27198391691,-32.4742356128,-10.1164167671));
#57865=CARTESIAN_POINT('Origin',(-4.01123091196E-15,-32.4742356128,-5.28091711198));
#57866=CARTESIAN_POINT('',(-10.831624024,-32.4742356128,-3.11921515388));
#57867=CARTESIAN_POINT('Origin',(2.84607155346,-32.4742356128,5.53854202767));
#57868=CARTESIAN_POINT('',(-10.32132295,-32.4742356128,5.39142026885));
#57869=CARTESIAN_POINT('Origin',(15.2935262605,-32.4742356128,-0.415072883442));
#57870=CARTESIAN_POINT('',(1.45716771982E-15,-32.4742356128,11.1232430723));
#57871=CARTESIAN_POINT('Origin',(0.0657457778947,-32.4742356128,-1.15388688513));
#57872=CARTESIAN_POINT('',(10.32132295,-32.4742356128,5.39142026885));
#57873=CARTESIAN_POINT('Origin',(-0.0657457778947,-32.4742356128,-1.15388688513));
#57874=CARTESIAN_POINT('',(10.831624024,-32.4742356128,-3.11921515388));
#57875=CARTESIAN_POINT('Origin',(-15.2935262605,-32.4742356128,-0.415072883442));
#57876=CARTESIAN_POINT('Origin',(-2.84607155346,-32.4742356128,5.53854202767));
#57877=CARTESIAN_POINT('Origin',(2.84607155346,-34.4242356128,5.53854202767));
#57878=CARTESIAN_POINT('',(-10.831624024,-32.8742356128,-3.11921515388));
#57879=CARTESIAN_POINT('',(-1.27198391691,-32.8742356128,-10.1164167671));
#57880=CARTESIAN_POINT('Origin',(2.84607155346,-32.8742356127999,5.53854202766998));
#57881=CARTESIAN_POINT('',(-10.831624024,-34.4242356128,-3.11921515388));
#57882=CARTESIAN_POINT('',(-1.27198391691,-32.6742356128,-10.1164167671));
#57883=CARTESIAN_POINT('Origin',(15.2935262605,-34.4242356128,-0.415072883442));
#57884=CARTESIAN_POINT('',(-10.32132295,-32.8742356128,5.39142026885));
#57885=CARTESIAN_POINT('',(-10.32132295,-34.4242356128,5.39142026885));
#57886=CARTESIAN_POINT('Origin',(15.2935262604996,-32.8742356127997,-0.415072883442075));
#57887=CARTESIAN_POINT('Origin',(0.0657457778947,-34.4242356128,-1.15388688513));
#57888=CARTESIAN_POINT('',(1.36002320517E-15,-32.8742356128,11.1232430723));
#57889=CARTESIAN_POINT('',(-1.1338152639E-14,-34.4242356128,11.1232430723));
#57890=CARTESIAN_POINT('Origin',(0.0657457778947039,-32.8742356128,-1.15388688512999));
#57891=CARTESIAN_POINT('Origin',(-0.0657457778947,-34.4242356128,-1.15388688513));
#57892=CARTESIAN_POINT('',(10.32132295,-32.8742356128,5.39142026885));
#57893=CARTESIAN_POINT('Origin',(-0.0657457778946926,-32.8742356128,-1.15388688513));
#57894=CARTESIAN_POINT('',(10.32132295,-34.4242356128,5.39142026885));
#57895=CARTESIAN_POINT('Origin',(-15.2935262605,-34.4242356128,-0.415072883442));
#57896=CARTESIAN_POINT('',(10.831624024,-32.8742356128,-3.11921515388));
#57897=CARTESIAN_POINT('Origin',(-15.2935262605,-32.8742356128002,-0.415072883441909));
#57898=CARTESIAN_POINT('',(10.831624024,-34.4242356128,-3.11921515388));
#57899=CARTESIAN_POINT('Origin',(-2.84607155346,-34.4242356128,5.53854202767));
#57900=CARTESIAN_POINT('',(1.27198391691,-32.8742356128,-10.1164167671));
#57901=CARTESIAN_POINT('Origin',(-2.84607155345998,-32.8742356128,5.53854202767));
#57902=CARTESIAN_POINT('',(1.27198391691,-32.6742356128,-10.1164167671));
#57903=CARTESIAN_POINT('Origin',(-4.06021678393E-15,-32.6742356128,-5.28091711198));
#57904=CARTESIAN_POINT('Origin',(3.05311331771918E-15,-32.8742356128,-5.28091711198007));
#57905=CARTESIAN_POINT('Origin',(-7.20309609018E-16,-32.8742356128,4.89858719659E-17));
#98281=UNCERTAINTY_MEASURE_WITH_UNIT(LENGTH_MEASURE(0.01),#98303,
'DISTANCE_ACCURACY_VALUE',
'Maximum model space distance between geometric entities at asserted c
onnectivities');
#98290=UNCERTAINTY_MEASURE_WITH_UNIT(LENGTH_MEASURE(0.01),#98303,
'DISTANCE_ACCURACY_VALUE',
'Maximum model space distance between geometric entities at asserted c
onnectivities');
#98293=(
GEOMETRIC_REPRESENTATION_CONTEXT(3)
GLOBAL_UNCERTAINTY_ASSIGNED_CONTEXT((#98281))
GLOBAL_UNIT_ASSIGNED_CONTEXT((#98303,#98305,#98306))
REPRESENTATION_CONTEXT('','3D')
);
#98302=(
GEOMETRIC_REPRESENTATION_CONTEXT(3)
GLOBAL_UNCERTAINTY_ASSIGNED_CONTEXT((#98290))
GLOBAL_UNIT_ASSIGNED_CONTEXT((#98303,#98305,#98306))
REPRESENTATION_CONTEXT('','3D')
);
#98303=(
LENGTH_UNIT()
NAMED_UNIT(*)
SI_UNIT(.MILLI.,.METRE.)
);
#98305=(
NAMED_UNIT(*)
PLANE_ANGLE_UNIT()
SI_UNIT($,.RADIAN.)
);
#98306=(
NAMED_UNIT(*)
SI_UNIT($,.STERADIAN.)
SOLID_ANGLE_UNIT()
);
#98309=SHAPE_DEFINITION_REPRESENTATION(#98320,#98341);
#98320=PRODUCT_DEFINITION_SHAPE('',$,#98353);
#98341=SHAPE_REPRESENTATION('',(#34303),#98293);
#98350=PRODUCT_DEFINITION_CONTEXT('part definition',#98385,'design');
#98353=PRODUCT_DEFINITION('Fixed Ceramic Disc','Fixed Ceramic Disc',#98364,
#98350);
#98364=PRODUCT_DEFINITION_FORMATION('',$,#98389);
#98385=APPLICATION_CONTEXT(
'Core Data for Automotive Mechanical Design Process');
#98386=PRODUCT_CONTEXT('part definition',#98385,'mechanical');
#98389=PRODUCT('Fixed Ceramic Disc','Fixed Ceramic Disc',$,(#98386));
#98399=PRESENTATION_STYLE_ASSIGNMENT((#98401));
#98401=SURFACE_STYLE_USAGE(.BOTH.,#98403);
#98403=SURFACE_SIDE_STYLE('',(#98405));
#98405=SURFACE_STYLE_FILL_AREA(#98407);
#98407=FILL_AREA_STYLE('Opaque(202,209,238)',(#98409));
#98409=FILL_AREA_STYLE_COLOUR('Opaque(202,209,238)',#98411);
#98411=COLOUR_RGB('Opaque(202,209,238)', 0.31764706, 0.68627451, 0.89019608);
ENDSEC;
END-ISO-10303-21;
